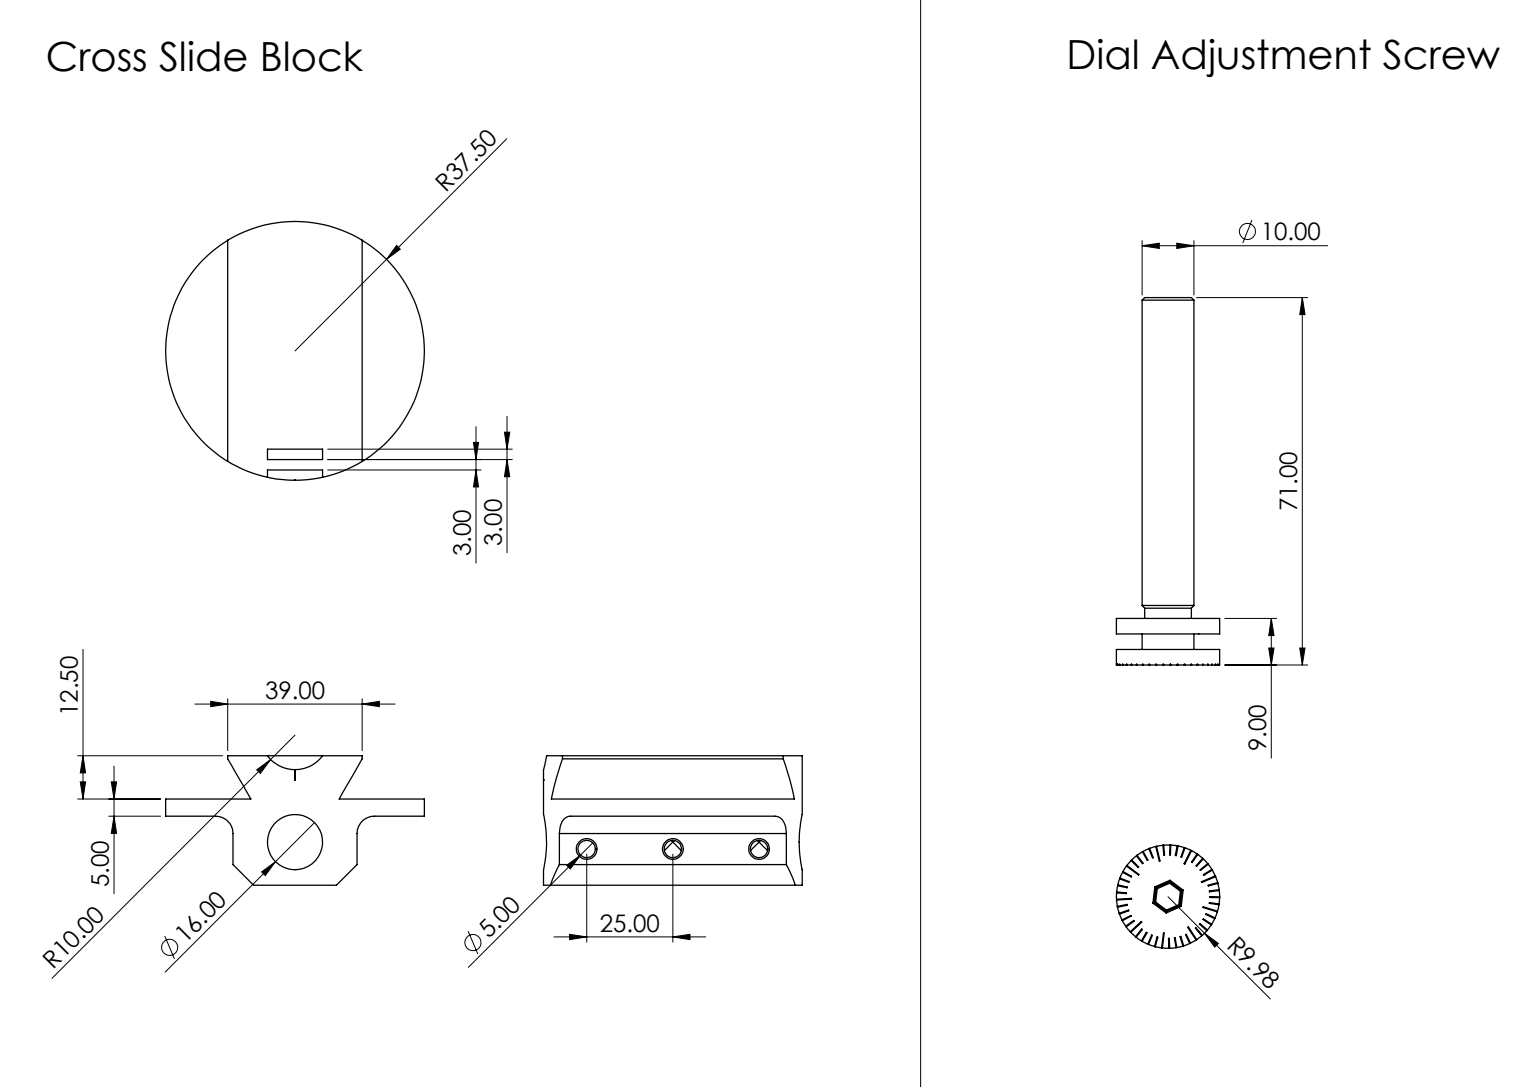
ISO-10303-21;
HEADER;
FILE_DESCRIPTION (('STEP AP214'),
    '1' );
FILE_NAME ('Dial Adjustment Screw.step',
    '2026-10-09T18:50:44',
    ( '' ),
    ( '' ),
    'SwSTEP 2.0',
    'SolidWorks 2026',
    '' );
FILE_SCHEMA (( 'AUTOMOTIVE_DESIGN' ));
ENDSEC;

DATA;
#4=EDGE_CURVE ( 'NONE', #9153, #8466, #14460, .T. ) ;
#6=LINE ( 'NONE', #11551, #10906 ) ;
#7=EDGE_CURVE ( 'NONE', #9450, #4202, #8492, .T. ) ;
#8=LINE ( 'NONE', #14787, #7820 ) ;
#11=ORIENTED_EDGE ( 'NONE', *, *, #1671, .F. ) ;
#12=DIRECTION ( 'NONE',  ( 8.018662683283438208E-16, -5.975035461963189015E-16, -1.000000000000000000 ) ) ;
#13=EDGE_LOOP ( 'NONE', ( #14568, #7332, #7097, #12565 ) ) ;
#14=CARTESIAN_POINT ( 'NONE',  ( -24.38380099443793725, -15.36048369738253427, 57.00231026484397745 ) ) ;
#15=ORIENTED_EDGE ( 'NONE', *, *, #4138, .F. ) ;
#17=VERTEX_POINT ( 'NONE', #8566 ) ;
#18=AXIS2_PLACEMENT_3D ( 'NONE', #7899, #12589, #2105 ) ;
#20=ORIENTED_EDGE ( 'NONE', *, *, #787, .F. ) ;
#25=ADVANCED_FACE ( 'NONE', ( #12243 ), #13329, .T. ) ;
#27=CARTESIAN_POINT ( 'NONE',  ( -8.600581100527527667, -9.311215824554304632, 56.85231026484400019 ) ) ;
#30=PLANE ( 'NONE',  #7847 ) ;
#31=ORIENTED_EDGE ( 'NONE', *, *, #8737, .F. ) ;
#32=DIRECTION ( 'NONE',  ( 0.4895147004624025855, -0.8719950447285834683, 9.135454576425998749E-16 ) ) ;
#33=VERTEX_POINT ( 'NONE', #4056 ) ;
#34=VERTEX_POINT ( 'NONE', #8713 ) ;
#35=CARTESIAN_POINT ( 'NONE',  ( -10.39628701978575975, -6.002951807498697612, 56.85231026484398598 ) ) ;
#43=CARTESIAN_POINT ( 'NONE',  ( -15.50552586659557797, -13.55703840903364288, 56.85231026484398598 ) ) ;
#46=CARTESIAN_POINT ( 'NONE',  ( -15.17726793795939599, -10.75904990174046461, 51.00231026484399166 ) ) ;
#49=ORIENTED_EDGE ( 'NONE', *, *, #8035, .T. ) ;
#52=ORIENTED_EDGE ( 'NONE', *, *, #5707, .T. ) ;
#54=EDGE_LOOP ( 'NONE', ( #11405, #3978, #7502, #8559 ) ) ;
#55=EDGE_CURVE ( 'NONE', #11066, #9490, #2977, .T. ) ;
#56=VECTOR ( 'NONE', #14424, 999.9999999999998863 ) ;
#57=VECTOR ( 'NONE', #8652, 999.9999999999998863 ) ;
#58=DIRECTION ( 'NONE',  ( -0.5104125104778984845, -0.8599296884906632021, 1.045284632676530333E-16 ) ) ;
#61=CARTESIAN_POINT ( 'NONE',  ( -12.46042140754850713, -23.00808483377100444, 57.00231026484399166 ) ) ;
#62=ORIENTED_EDGE ( 'NONE', *, *, #12874, .F. ) ;
#63=DIRECTION ( 'NONE',  ( -0.3306575217771102193, 0.9437508163134058492, -8.290375725550400094E-16 ) ) ;
#65=DIRECTION ( 'NONE',  ( 0.9354976265738682573, -0.3533329742249642913, 9.612616959383187437E-16 ) ) ;
#66=ORIENTED_EDGE ( 'NONE', *, *, #12766, .T. ) ;
#67=CIRCLE ( 'NONE', #8607, 9.974999999999999645 ) ;
#68=AXIS2_PLACEMENT_3D ( 'NONE', #8168, #77, #12858 ) ;
#70=ORIENTED_EDGE ( 'NONE', *, *, #13189, .F. ) ;
#72=EDGE_LOOP ( 'NONE', ( #9972, #5659, #4429, #2400 ) ) ;
#77=DIRECTION ( 'NONE',  ( 0.7350174335289139105, -0.6780482080269579770, 9.945218953682734920E-16 ) ) ;
#78=DIRECTION ( 'NONE',  ( 0.9931883319083343320, -0.1165201156931293391, 8.660254037844387408E-16 ) ) ;
#80=VECTOR ( 'NONE', #13700, 1000.000000000000114 ) ;
#83=PLANE ( 'NONE',  #4186 ) ;
#84=CARTESIAN_POINT ( 'NONE',  ( -7.424382730750140880, -13.52981220323889566, 56.85231026484400019 ) ) ;
#85=ORIENTED_EDGE ( 'NONE', *, *, #97, .F. ) ;
#87=ORIENTED_EDGE ( 'NONE', *, *, #11967, .T. ) ;
#94=LINE ( 'NONE', #9566, #672 ) ;
#96=DIRECTION ( 'NONE',  ( -8.018662683283438208E-16, 5.975035461963189015E-16, 1.000000000000000000 ) ) ;
#97=EDGE_CURVE ( 'NONE', #6821, #6890, #11166, .T. ) ;
#100=LINE ( 'NONE', #14015, #4170 ) ;
#105=CARTESIAN_POINT ( 'NONE',  ( -11.67714598312096008, -19.46131314156662384, 56.85231026484400019 ) ) ;
#113=ORIENTED_EDGE ( 'NONE', *, *, #12612, .F. ) ;
#115=EDGE_CURVE ( 'NONE', #11608, #7250, #12699, .T. ) ;
#117=EDGE_CURVE ( 'NONE', #4448, #10428, #688, .T. ) ;
#118=VERTEX_POINT ( 'NONE', #5499 ) ;
#119=CARTESIAN_POINT ( 'NONE',  ( -15.49969986081092088, -13.50737899243822504, 57.00231026484397745 ) ) ;
#123=LINE ( 'NONE', #4934, #14525 ) ;
#124=COLOUR_RGB ( '', 0.72549020, 0.75294118, 0.79215686) ;
#127=ORIENTED_EDGE ( 'NONE', *, *, #115, .F. ) ;
#129=DIRECTION ( 'NONE',  ( 0.9645173894937585368, 0.2640193276336892936, 6.156614753256587028E-16 ) ) ;
#131=CARTESIAN_POINT ( 'NONE',  ( -8.744347237509680681, -17.93190845158491342, 57.00231026484399166 ) ) ;
#132=ADVANCED_FACE ( 'NONE', ( #4206 ), #14685, .F. ) ;
#135=ORIENTED_EDGE ( 'NONE', *, *, #11324, .F. ) ;
#137=VECTOR ( 'NONE', #5946, 999.9999999999998863 ) ;
#141=DIRECTION ( 'NONE',  ( -8.018662683283438208E-16, 5.975035461963189015E-16, 1.000000000000000000 ) ) ;
#149=PLANE ( 'NONE',  #14987 ) ;
#150=VERTEX_POINT ( 'NONE', #916 ) ;
#154=FACE_OUTER_BOUND ( 'NONE', #467, .T. ) ;
#156=CARTESIAN_POINT ( 'NONE',  ( -17.71860670988920816, -11.85398021090886367, 51.00231026484399166 ) ) ;
#157=VECTOR ( 'NONE', #7597, 1000.000000000000114 ) ;
#159=EDGE_CURVE ( 'NONE', #10747, #3108, #3053, .T. ) ;
#165=ORIENTED_EDGE ( 'NONE', *, *, #2149, .T. ) ;
#166=DIRECTION ( 'NONE',  ( 8.018662683283438208E-16, -5.975035461963189015E-16, -1.000000000000000000 ) ) ;
#167=ORIENTED_EDGE ( 'NONE', *, *, #12641, .F. ) ;
#169=ORIENTED_EDGE ( 'NONE', *, *, #13036, .F. ) ;
#171=CARTESIAN_POINT ( 'NONE',  ( -15.49969986081092088, -13.50737899243822504, 56.85231026484398598 ) ) ;
#173=FACE_OUTER_BOUND ( 'NONE', #4854, .T. ) ;
#175=SHAPE_REPRESENTATION_RELATIONSHIP ( 'NONE' , 'NONE' ,  #13495, #6601 ) ;
#176=CARTESIAN_POINT ( 'NONE',  ( -18.41596830400278506, -14.76384693893611910, 57.00231026484397745 ) ) ;
#178=AXIS2_PLACEMENT_3D ( 'NONE', #14596, #7550, #6095 ) ;
#183=EDGE_LOOP ( 'NONE', ( #8383, #10689, #169, #12159 ) ) ;
#185=AXIS2_PLACEMENT_3D ( 'NONE', #4466, #10423, #5753 ) ;
#186=VERTEX_POINT ( 'NONE', #14912 ) ;
#188=ORIENTED_EDGE ( 'NONE', *, *, #5314, .T. ) ;
#191=FACE_OUTER_BOUND ( 'NONE', #10169, .T. ) ;
#192=DIRECTION ( 'NONE',  ( 0.5975035461963189576, 0.8018662683283437342, 0.000000000000000000 ) ) ;
#193=EDGE_CURVE ( 'NONE', #1606, #4275, #8746, .T. ) ;
#194=EDGE_CURVE ( 'NONE', #4315, #8561, #7264, .T. ) ;
#195=CARTESIAN_POINT ( 'NONE',  ( -15.49969986081091022, -13.50737899243823215, 46.00231026484398456 ) ) ;
#196=LINE ( 'NONE', #3708, #2723 ) ;
#197=CARTESIAN_POINT ( 'NONE',  ( -8.681233859935401753, -6.226640953275941470, 56.85231026484398598 ) ) ;
#203=EDGE_LOOP ( 'NONE', ( #1328, #2305, #6910, #14868 ) ) ;
#204=ORIENTED_EDGE ( 'NONE', *, *, #10815, .T. ) ;
#207=ORIENTED_EDGE ( 'NONE', *, *, #11956, .F. ) ;
#210=CARTESIAN_POINT ( 'NONE',  ( -17.47506273705024071, -21.33739760717825718, 56.85231026484400019 ) ) ;
#211=EDGE_CURVE ( 'NONE', #12427, #2827, #11544, .T. ) ;
#212=DIRECTION ( 'NONE',  ( 0.6859287159822015090, -0.7276687409742212953, 9.848077530122081084E-16 ) ) ;
#215=ORIENTED_EDGE ( 'NONE', *, *, #13065, .F. ) ;
#217=CARTESIAN_POINT ( 'NONE',  ( -10.84210729886283531, -6.910555398701176522, 56.85231026484398598 ) ) ;
#218=ORIENTED_EDGE ( 'NONE', *, *, #1842, .T. ) ;
#221=VERTEX_POINT ( 'NONE', #11762 ) ;
#224=ORIENTED_EDGE ( 'NONE', *, *, #12134, .T. ) ;
#225=FACE_OUTER_BOUND ( 'NONE', #3388, .T. ) ;
#227=EDGE_CURVE ( 'NONE', #9086, #8293, #11691, .T. ) ;
#230=VECTOR ( 'NONE', #6999, 1000.000000000000000 ) ;
#235=DIRECTION ( 'NONE',  ( -8.018662683283438208E-16, 5.975035461963189015E-16, 1.000000000000000000 ) ) ;
#236=CARTESIAN_POINT ( 'NONE',  ( -16.32407967933980686, -20.53418644068968746, 57.00231026484399166 ) ) ;
#239=DIRECTION ( 'NONE',  ( 8.018662683283438208E-16, -5.975035461963189015E-16, -1.000000000000000000 ) ) ;
#242=CARTESIAN_POINT ( 'NONE',  ( -18.04596724311489808, -11.61005040962811563, 57.00231026484397745 ) ) ;
#247=ORIENTED_EDGE ( 'NONE', *, *, #4682, .F. ) ;
#252=DIRECTION ( 'NONE',  ( 0.5975035461963189576, 0.8018662683283437342, 0.000000000000000000 ) ) ;
#254=CARTESIAN_POINT ( 'NONE',  ( -24.01584079503567182, -10.37104457333969876, 57.00231026484397745 ) ) ;
#255=CARTESIAN_POINT ( 'NONE',  ( -15.47224238247604511, -13.54916519690201149, 56.85231026484398598 ) ) ;
#256=VECTOR ( 'NONE', #11415, 1000.000000000000114 ) ;
#257=ORIENTED_EDGE ( 'NONE', *, *, #6613, .T. ) ;
#262=ORIENTED_EDGE ( 'NONE', *, *, #3647, .F. ) ;
#263=CARTESIAN_POINT ( 'NONE',  ( -23.39388780995641781, -11.80648316271623877, 56.85231026484398598 ) ) ;
#270=CIRCLE ( 'NONE', #3683, 9.974999999999999645 ) ;
#282=EDGE_CURVE ( 'NONE', #626, #3416, #13005, .T. ) ;
#284=ADVANCED_FACE ( 'NONE', ( #2513 ), #11846, .F. ) ;
#286=AXIS2_PLACEMENT_3D ( 'NONE', #4236, #8813, #2856 ) ;
#288=EDGE_CURVE ( 'NONE', #14042, #11463, #13916, .T. ) ;
#289=CARTESIAN_POINT ( 'NONE',  ( -24.32830346761242879, -18.15026423267100597, 56.85231026484398598 ) ) ;
#291=ORIENTED_EDGE ( 'NONE', *, *, #2351, .F. ) ;
#294=ORIENTED_EDGE ( 'NONE', *, *, #11168, .F. ) ;
#295=DIRECTION ( 'NONE',  ( 0.9437508163134050720, 0.3306575217771122732, 5.591929034707472732E-16 ) ) ;
#298=LINE ( 'NONE', #4183, #349 ) ;
#306=DIRECTION ( 'NONE',  ( 0.2301973227387160703, -0.9731439732146149879, 7.660444431189776467E-16 ) ) ;
#307=VECTOR ( 'NONE', #2927, 999.9999999999998863 ) ;
#308=CIRCLE ( 'NONE', #8106, 9.974999999999999645 ) ;
#309=VECTOR ( 'NONE', #4436, 1000.000000000000000 ) ;
#310=LINE ( 'NONE', #9632, #1371 ) ;
#315=CARTESIAN_POINT ( 'NONE',  ( -23.54151295824578227, -12.77219731018227300, 57.00231026484397745 ) ) ;
#316=CARTESIAN_POINT ( 'NONE',  ( -6.938526287600617515, -8.388108336439909607, 57.00231026484399166 ) ) ;
#319=ORIENTED_EDGE ( 'NONE', *, *, #11952, .F. ) ;
#320=DIRECTION ( 'NONE',  ( -0.1855175943453192255, -0.9826409426582660700, 4.383711467890751032E-16 ) ) ;
#321=FACE_OUTER_BOUND ( 'NONE', #7198, .T. ) ;
#322=EDGE_LOOP ( 'NONE', ( #14404, #10872, #12403, #8371 ) ) ;
#323=VECTOR ( 'NONE', #13122, 1000.000000000000114 ) ;
#325=DIRECTION ( 'NONE',  ( 0.9988970074402866439, -0.04695496274985035134, 8.290375725550441510E-16 ) ) ;
#326=VECTOR ( 'NONE', #4845, 1000.000000000000000 ) ;
#329=DIRECTION ( 'NONE',  ( -8.018662683283438208E-16, 5.975035461963189015E-16, 1.000000000000000000 ) ) ;
#336=DIRECTION ( 'NONE',  ( 8.018662683283438208E-16, -5.975035461963189015E-16, -1.000000000000000000 ) ) ;
#337=VERTEX_POINT ( 'NONE', #13812 ) ;
#341=LINE ( 'NONE', #7503, #3156 ) ;
#343=ORIENTED_EDGE ( 'NONE', *, *, #4783, .T. ) ;
#346=ORIENTED_EDGE ( 'NONE', *, *, #6966, .T. ) ;
#347=LINE ( 'NONE', #11884, #5404 ) ;
#348=DIRECTION ( 'NONE',  ( 8.018662683283438208E-16, -5.975035461963189015E-16, -1.000000000000000000 ) ) ;
#349=VECTOR ( 'NONE', #8838, 1000.000000000000114 ) ;
#351=CARTESIAN_POINT ( 'NONE',  ( -16.26465502354534465, -4.464365468230401923, 56.85231026484398598 ) ) ;
#353=CARTESIAN_POINT ( 'NONE',  ( -15.49969986081091022, -13.50737899243823215, 45.50231026484398456 ) ) ;
#354=EDGE_CURVE ( 'NONE', #745, #9450, #1038, .T. ) ;
#355=CARTESIAN_POINT ( 'NONE',  ( -20.31707134655588121, -4.772760685475329723, 57.00231026484397745 ) ) ;
#358=CARTESIAN_POINT ( 'NONE',  ( -17.98267069058175593, -13.21607870320540279, 51.25231026484399166 ) ) ;
#359=CARTESIAN_POINT ( 'NONE',  ( -14.15531688186919901, -11.70317988869945580, 51.25231026484399166 ) ) ;
#361=ORIENTED_EDGE ( 'NONE', *, *, #5740, .T. ) ;
#362=VECTOR ( 'NONE', #6575, 1000.000000000000000 ) ;
#366=AXIS2_PLACEMENT_3D ( 'NONE', #8590, #7864, #7944 ) ;
#368=VECTOR ( 'NONE', #4802, 1000.000000000000000 ) ;
#369=LINE ( 'NONE', #7224, #14846 ) ;
#371=CARTESIAN_POINT ( 'NONE',  ( -9.204203523554131294, -8.449911655164932256, 56.85231026484398598 ) ) ;
#373=DIRECTION ( 'NONE',  ( -8.018662683283438208E-16, 5.975035461963189015E-16, 1.000000000000000000 ) ) ;
#375=LINE ( 'NONE', #5935, #15083 ) ;
#378=EDGE_CURVE ( 'NONE', #12795, #6835, #5541, .T. ) ;
#382=LINE ( 'NONE', #13374, #828 ) ;
#383=EDGE_LOOP ( 'NONE', ( #11482, #7292, #5223, #897 ) ) ;
#391=EDGE_CURVE ( 'NONE', #6478, #4633, #15029, .T. ) ;
#392=CARTESIAN_POINT ( 'NONE',  ( -7.829332545557822876, -7.130382030772259405, 54.00231026484399166 ) ) ;
#395=CARTESIAN_POINT ( 'NONE',  ( -10.27295246487022240, -6.088325032597582620, 56.85231026484398598 ) ) ;
#396=ORIENTED_EDGE ( 'NONE', *, *, #11686, .F. ) ;
#398=EDGE_LOOP ( 'NONE', ( #9560, #11347, #6065, #9121, #218, #1341, #14177, #5755, #9138, #2250, #8409, #841, #3009, #12196, #3012, #215, #6805, #10450, #11048, #3124, #8673, #4543, #13338, #1727, #6461, #20, #10686, #9196, #12441, #10883, #7309, #5437, #1481, #5195, #2738, #14936, #13462, #1244, #15109, #5142, #4772, #10095, #7336, #13120, #462, #7253, #2154, #14889, #4656, #3287, #6719, #5542, #5255, #5721, #5056, #7185, #6602, #11840, #12110, #9524, #2176, #7888, #3618, #840, #2267, #1060, #11943, #5202, #12654, #8703, #7274, #1364, #12906, #13394, #10919, #9271, #428, #5605, #11, #4999, #1774, #7100, #4480, #2417, #10113, #7120, #11578, #6781, #13390, #6535, #3685, #6336, #9887, #10899, #2644, #11457 ) ) ;
#400=PLANE ( 'NONE',  #4949 ) ;
#401=CARTESIAN_POINT ( 'NONE',  ( -7.426192534185826588, -13.67980128487994129, 56.85231026484400019 ) ) ;
#403=CIRCLE ( 'NONE', #7222, 9.974999999999999645 ) ;
#407=CARTESIAN_POINT ( 'NONE',  ( -8.639554752241616953, -9.247137322136806503, 57.00231026484399166 ) ) ;
#408=CARTESIAN_POINT ( 'NONE',  ( -15.83606446161809522, -16.37446674635458166, 56.75231026484397745 ) ) ;
#413=VERTEX_POINT ( 'NONE', #3179 ) ;
#414=CARTESIAN_POINT ( 'NONE',  ( -17.86883904694317593, -3.817807045405069655, 56.85231026484398598 ) ) ;
#417=CARTESIAN_POINT ( 'NONE',  ( -15.49969986081092088, -13.50737899243822504, 57.00231026484397745 ) ) ;
#420=DIRECTION ( 'NONE',  ( -8.018662683283438208E-16, 5.975035461963189015E-16, 1.000000000000000000 ) ) ;
#423=PRODUCT_DEFINITION_SHAPE ( 'NONE', 'NONE',  #14249 ) ;
#426=ORIENTED_EDGE ( 'NONE', *, *, #5229, .F. ) ;
#428=ORIENTED_EDGE ( 'NONE', *, *, #3740, .T. ) ;
#430=ORIENTED_EDGE ( 'NONE', *, *, #211, .T. ) ;
#432=PLANE ( 'NONE',  #8349 ) ;
#436=CARTESIAN_POINT ( 'NONE',  ( -15.54961651457173488, -13.51026476396819831, 56.85231026484398598 ) ) ;
#439=FACE_OUTER_BOUND ( 'NONE', #5049, .T. ) ;
#440=CARTESIAN_POINT ( 'NONE',  ( -6.488891646287396675, -12.42729319905174634, 57.00231026484399166 ) ) ;
#443=CARTESIAN_POINT ( 'NONE',  ( -18.18846581869435042, -17.11577719991577595, 48.00231026484398456 ) ) ;
#446=LINE ( 'NONE', #6386, #12519 ) ;
#449=CARTESIAN_POINT ( 'NONE',  ( -14.10579935493720782, -22.47500361547664127, 56.85231026484400019 ) ) ;
#450=ORIENTED_EDGE ( 'NONE', *, *, #10660, .T. ) ;
#451=DIRECTION ( 'NONE',  ( -0.4491835085186243748, -0.8934395198752397294, 1.736481776669299976E-16 ) ) ;
#452=AXIS2_PLACEMENT_3D ( 'NONE', #12447, #14978, #15050 ) ;
#456=AXIS2_PLACEMENT_3D ( 'NONE', #14616, #2988, #10880 ) ;
#457=FACE_OUTER_BOUND ( 'NONE', #11590, .T. ) ;
#462=ORIENTED_EDGE ( 'NONE', *, *, #5462, .T. ) ;
#464=CARTESIAN_POINT ( 'NONE',  ( -6.766506000727597225, -11.03906478995046214, 57.00231026484399166 ) ) ;
#467=EDGE_LOOP ( 'NONE', ( #13198, #13690 ) ) ;
#469=ORIENTED_EDGE ( 'NONE', *, *, #1383, .F. ) ;
#471=DIRECTION ( 'NONE',  ( 0.02283895005205794151, -0.9997391571607663341, 6.156614753256579139E-16 ) ) ;
#473=ADVANCED_FACE ( 'NONE', ( #4936 ), #4865, .T. ) ;
#474=EDGE_CURVE ( 'NONE', #5883, #11022, #2563, .T. ) ;
#475=CARTESIAN_POINT ( 'NONE',  ( -9.452813543643186378, -20.27468391147722926, 56.85231026484400019 ) ) ;
#480=PLANE ( 'NONE',  #13859 ) ;
#482=EDGE_CURVE ( 'NONE', #8690, #13854, #8445, .T. ) ;
#485=ORIENTED_EDGE ( 'NONE', *, *, #2144, .T. ) ;
#489=PLANE ( 'NONE',  #5895 ) ;
#494=DIRECTION ( 'NONE',  ( -8.018662683283438208E-16, 5.975035461963189015E-16, 1.000000000000000000 ) ) ;
#495=DIRECTION ( 'NONE',  ( 8.018662683283438208E-16, -5.975035461963189015E-16, -1.000000000000000000 ) ) ;
#497=FACE_OUTER_BOUND ( 'NONE', #9125, .T. ) ;
#498=ORIENTED_EDGE ( 'NONE', *, *, #6384, .T. ) ;
#500=DIRECTION ( 'NONE',  ( -8.018662683283438208E-16, 5.975035461963189015E-16, 1.000000000000000000 ) ) ;
#501=ORIENTED_EDGE ( 'NONE', *, *, #8338, .F. ) ;
#502=ORIENTED_EDGE ( 'NONE', *, *, #12063, .T. ) ;
#503=EDGE_CURVE ( 'NONE', #10963, #7558, #4786, .T. ) ;
#505=VERTEX_POINT ( 'NONE', #5991 ) ;
#506=CARTESIAN_POINT ( 'NONE',  ( -25.21423696146293736, -11.24278324042066046, 54.00231026484397745 ) ) ;
#512=CARTESIAN_POINT ( 'NONE',  ( -11.08622897860377954, -4.561882931743225456, 56.85231026484398598 ) ) ;
#514=EDGE_LOOP ( 'NONE', ( #9562, #13979, #13683, #11446 ) ) ;
#517=DIRECTION ( 'NONE',  ( -8.018662683283438208E-16, 5.975035461963189015E-16, 1.000000000000000000 ) ) ;
#519=LINE ( 'NONE', #449, #1066 ) ;
#520=ORIENTED_EDGE ( 'NONE', *, *, #7971, .F. ) ;
#522=VECTOR ( 'NONE', #10897, 1000.000000000000114 ) ;
#523=FACE_OUTER_BOUND ( 'NONE', #3562, .T. ) ;
#524=CARTESIAN_POINT ( 'NONE',  ( -7.426192534185826588, -13.67980128487993952, 57.00231026484399166 ) ) ;
#527=ORIENTED_EDGE ( 'NONE', *, *, #9531, .T. ) ;
#529=LINE ( 'NONE', #4977, #7993 ) ;
#530=AXIS2_PLACEMENT_3D ( 'NONE', #12947, #6943, #12 ) ;
#532=VERTEX_POINT ( 'NONE', #13131 ) ;
#533=ORIENTED_EDGE ( 'NONE', *, *, #1466, .T. ) ;
#536=ORIENTED_EDGE ( 'NONE', *, *, #10912, .T. ) ;
#537=DIRECTION ( 'NONE',  ( 0.1165201156931293391, 0.9931883319083343320, -4.999999999999998416E-16 ) ) ;
#538=DIRECTION ( 'NONE',  ( -0.9673062255102924389, 0.2536112499260064768, -9.271838545667833343E-16 ) ) ;
#539=VECTOR ( 'NONE', #6589, 999.9999999999998863 ) ;
#541=VECTOR ( 'NONE', #2213, 1000.000000000000000 ) ;
#544=CARTESIAN_POINT ( 'NONE',  ( -5.526612771747954511, -13.70272205979775215, 57.00231026484399166 ) ) ;
#550=CIRCLE ( 'NONE', #2008, 5.000000000000000000 ) ;
#551=VERTEX_POINT ( 'NONE', #4711 ) ;
#552=AXIS2_PLACEMENT_3D ( 'NONE', #3432, #12781, #11690 ) ;
#553=ORIENTED_EDGE ( 'NONE', *, *, #12726, .F. ) ;
#555=ORIENTED_EDGE ( 'NONE', *, *, #2708, .T. ) ;
#557=CIRCLE ( 'NONE', #1776, 9.974999999999999645 ) ;
#560=VERTEX_POINT ( 'NONE', #197 ) ;
#561=DIRECTION ( 'NONE',  ( -0.9183863840214728791, -0.3956847857120156520, -4.999999999999998416E-16 ) ) ;
#564=CARTESIAN_POINT ( 'NONE',  ( -9.204203523554131294, -8.449911655164932256, 56.85231026484398598 ) ) ;
#568=EDGE_CURVE ( 'NONE', #9210, #8324, #1106, .T. ) ;
#572=VERTEX_POINT ( 'NONE', #7518 ) ;
#579=VECTOR ( 'NONE', #5511, 1000.000000000000000 ) ;
#580=CIRCLE ( 'NONE', #12062, 9.974999999999999645 ) ;
#585=AXIS2_PLACEMENT_3D ( 'NONE', #3960, #12144, #9989 ) ;
#586=DIRECTION ( 'NONE',  ( -8.018662683283438208E-16, 5.975035461963189015E-16, 1.000000000000000000 ) ) ;
#588=ORIENTED_EDGE ( 'NONE', *, *, #6627, .F. ) ;
#591=CARTESIAN_POINT ( 'NONE',  ( -12.69917084408742269, -12.16466883763078144, 57.00231026484397745 ) ) ;
#592=EDGE_LOOP ( 'NONE', ( #1009, #7727, #14645, #8081 ) ) ;
#593=EDGE_CURVE ( 'NONE', #3314, #3333, #9963, .T. ) ;
#595=PLANE ( 'NONE',  #7643 ) ;
#596=AXIS2_PLACEMENT_3D ( 'NONE', #4175, #9910, #7609 ) ;
#597=ORIENTED_EDGE ( 'NONE', *, *, #4963, .F. ) ;
#598=LINE ( 'NONE', #13310, #13985 ) ;
#599=VECTOR ( 'NONE', #12678, 1000.000000000000114 ) ;
#600=FACE_OUTER_BOUND ( 'NONE', #3661, .T. ) ;
#601=EDGE_CURVE ( 'NONE', #7394, #8222, #3773, .T. ) ;
#602=CARTESIAN_POINT ( 'NONE',  ( -24.36945568363038461, -11.58678490633884373, 56.85231026484398598 ) ) ;
#604=DIRECTION ( 'NONE',  ( -8.018662683283439195E-16, 5.975035461963190001E-16, 1.000000000000000000 ) ) ;
#612=VERTEX_POINT ( 'NONE', #6137 ) ;
#614=FACE_OUTER_BOUND ( 'NONE', #3144, .T. ) ;
#615=ORIENTED_EDGE ( 'NONE', *, *, #11602, .F. ) ;
#616=CARTESIAN_POINT ( 'NONE',  ( -22.67472226038933059, -17.21206232108429290, 56.85231026484398598 ) ) ;
#617=LINE ( 'NONE', #14613, #11114 ) ;
#618=VECTOR ( 'NONE', #14146, 1000.000000000000000 ) ;
#619=EDGE_CURVE ( 'NONE', #13349, #1021, #9822, .T. ) ;
#621=CARTESIAN_POINT ( 'NONE',  ( -8.971570239337625097, -21.04953708182106453, 54.00231026484400587 ) ) ;
#625=DIRECTION ( 'NONE',  ( 8.018662683283438208E-16, -5.975035461963189015E-16, -1.000000000000000000 ) ) ;
#626=VERTEX_POINT ( 'NONE', #2711 ) ;
#628=LINE ( 'NONE', #12406, #4473 ) ;
#629=ORIENTED_EDGE ( 'NONE', *, *, #8780, .T. ) ;
#631=DIRECTION ( 'NONE',  ( 0.7953815700667045130, 0.6061090314441981430, 2.756373558170028881E-16 ) ) ;
#635=ADVANCED_FACE ( 'NONE', ( #7365 ), #7594, .F. ) ;
#636=LINE ( 'NONE', #10968, #4651 ) ;
#637=DIRECTION ( 'NONE',  ( 0.9885168150181788960, -0.1511109077013150503, 8.829475928589270966E-16 ) ) ;
#638=EDGE_CURVE ( 'NONE', #2290, #7645, #5016, .T. ) ;
#639=CIRCLE ( 'NONE', #9181, 5.000000000000000000 ) ;
#640=DIRECTION ( 'NONE',  ( 0.2196982563774038943, 0.9755678736739584744, -4.067366430757999696E-16 ) ) ;
#642=VERTEX_POINT ( 'NONE', #14489 ) ;
#643=LINE ( 'NONE', #8596, #7755 ) ;
#646=ORIENTED_EDGE ( 'NONE', *, *, #10912, .F. ) ;
#652=CARTESIAN_POINT ( 'NONE',  ( -7.902754534677060683, -18.47202114588016642, 57.00231026484399166 ) ) ;
#653=ADVANCED_FACE ( 'NONE', ( #8814 ), #3427, .T. ) ;
#656=EDGE_CURVE ( 'NONE', #2388, #14032, #13686, .T. ) ;
#657=DIRECTION ( 'NONE',  ( 0.9918751611018171710, 0.1272150336605075427, 7.193398003386516820E-16 ) ) ;
#659=ORIENTED_EDGE ( 'NONE', *, *, #13177, .F. ) ;
#660=DIRECTION ( 'NONE',  ( -8.018662683283438208E-16, 5.975035461963189015E-16, 1.000000000000000000 ) ) ;
#662=EDGE_CURVE ( 'NONE', #1582, #10428, #4356, .T. ) ;
#664=CARTESIAN_POINT ( 'NONE',  ( -25.21423696146293736, -11.24278324042065869, 57.00231026484397745 ) ) ;
#667=CARTESIAN_POINT ( 'NONE',  ( -20.33437667196779586, -7.039214636791314206, 57.00231026484397745 ) ) ;
#668=PLANE ( 'NONE',  #10986 ) ;
#669=EDGE_CURVE ( 'NONE', #6892, #5883, #6927, .T. ) ;
#671=FACE_OUTER_BOUND ( 'NONE', #6924, .T. ) ;
#672=VECTOR ( 'NONE', #3759, 1000.000000000000000 ) ;
#673=CARTESIAN_POINT ( 'NONE',  ( -22.55857771067089246, -13.99059064457067336, 56.85231026484398598 ) ) ;
#674=LINE ( 'NONE', #5559, #2557 ) ;
#675=ORIENTED_EDGE ( 'NONE', *, *, #3273, .T. ) ;
#678=ORIENTED_EDGE ( 'NONE', *, *, #6782, .T. ) ;
#679=VECTOR ( 'NONE', #12925, 1000.000000000000000 ) ;
#683=ORIENTED_EDGE ( 'NONE', *, *, #15059, .F. ) ;
#685=VECTOR ( 'NONE', #13993, 1000.000000000000000 ) ;
#686=VECTOR ( 'NONE', #8907, 1000.000000000000000 ) ;
#688=LINE ( 'NONE', #14986, #1664 ) ;
#689=FACE_OUTER_BOUND ( 'NONE', #11088, .T. ) ;
#692=AXIS2_PLACEMENT_3D ( 'NONE', #11251, #12556, #6566 ) ;
#693=DIRECTION ( 'NONE',  ( 8.018662683283438208E-16, -5.975035461963189015E-16, -1.000000000000000000 ) ) ;
#694=CARTESIAN_POINT ( 'NONE',  ( -15.82213178366242978, -16.25570808313599258, 51.00231026484399166 ) ) ;
#695=VECTOR ( 'NONE', #3479, 1000.000000000000000 ) ;
#696=CARTESIAN_POINT ( 'NONE',  ( -10.39628701978575975, -6.002951807498697612, 57.00231026484397745 ) ) ;
#699=LINE ( 'NONE', #12712, #5166 ) ;
#701=FACE_OUTER_BOUND ( 'NONE', #3699, .T. ) ;
#704=ORIENTED_EDGE ( 'NONE', *, *, #9052, .F. ) ;
#705=VECTOR ( 'NONE', #1786, 1000.000000000000000 ) ;
#707=DIRECTION ( 'NONE',  ( -0.9999272109403024578, 0.01206535623792159839, -8.090169943749490479E-16 ) ) ;
#710=PLANE ( 'NONE',  #9268 ) ;
#711=DIRECTION ( 'NONE',  ( 8.018662683283438208E-16, -5.975035461963189015E-16, -1.000000000000000000 ) ) ;
#712=FACE_OUTER_BOUND ( 'NONE', #3959, .T. ) ;
#715=CARTESIAN_POINT ( 'NONE',  ( -12.72810521832141362, -22.14910990341453001, 56.85231026484400019 ) ) ;
#719=CARTESIAN_POINT ( 'NONE',  ( -14.19354049678269192, -21.47604090745013750, 57.00231026484399166 ) ) ;
#721=ORIENTED_EDGE ( 'NONE', *, *, #9534, .T. ) ;
#725=ORIENTED_EDGE ( 'NONE', *, *, #11167, .T. ) ;
#727=VECTOR ( 'NONE', #4187, 1000.000000000000114 ) ;
#729=EDGE_CURVE ( 'NONE', #10731, #4396, #14907, .T. ) ;
#731=PLANE ( 'NONE',  #6812 ) ;
#735=ORIENTED_EDGE ( 'NONE', *, *, #7834, .F. ) ;
#737=PLANE ( 'NONE',  #10590 ) ;
#738=ORIENTED_EDGE ( 'NONE', *, *, #13177, .T. ) ;
#739=PLANE ( 'NONE',  #6134 ) ;
#743=EDGE_CURVE ( 'NONE', #11608, #1039, #13759, .T. ) ;
#744=LINE ( 'NONE', #11372, #7897 ) ;
#745=VERTEX_POINT ( 'NONE', #8076 ) ;
#747=EDGE_CURVE ( 'NONE', #1568, #4448, #14520, .T. ) ;
#748=DIRECTION ( 'NONE',  ( 0.05771543059946733500, -0.9983330752162417054, 6.427876096865391919E-16 ) ) ;
#751=AXIS2_PLACEMENT_3D ( 'NONE', #13106, #11949, #1467 ) ;
#754=CARTESIAN_POINT ( 'NONE',  ( -22.64031343690345111, -17.27870339600297811, 56.85231026484398598 ) ) ;
#757=DIRECTION ( 'NONE',  ( 0.5975035461963189576, 0.8018662683283437342, 0.000000000000000000 ) ) ;
#758=ADVANCED_FACE ( 'NONE', ( #14979 ), #10465, .T. ) ;
#764=DIRECTION ( 'NONE',  ( 0.5975035461963189576, 0.8018662683283437342, 0.000000000000000000 ) ) ;
#769=VECTOR ( 'NONE', #4307, 1000.000000000000000 ) ;
#772=FACE_OUTER_BOUND ( 'NONE', #10937, .T. ) ;
#773=ORIENTED_EDGE ( 'NONE', *, *, #13542, .F. ) ;
#782=ORIENTED_EDGE ( 'NONE', *, *, #10510, .F. ) ;
#783=CIRCLE ( 'NONE', #9322, 9.974999999999999645 ) ;
#784=CARTESIAN_POINT ( 'NONE',  ( -19.55678615628314532, -20.48959216528617233, 57.00231026484397745 ) ) ;
#785=CARTESIAN_POINT ( 'NONE',  ( -12.72810521832141362, -22.14910990341453001, 56.85231026484400019 ) ) ;
#787=EDGE_CURVE ( 'NONE', #6222, #34, #13589, .T. ) ;
#788=EDGE_CURVE ( 'NONE', #4102, #4546, #10127, .T. ) ;
#789=AXIS2_PLACEMENT_3D ( 'NONE', #6840, #972, #4339 ) ;
#791=DIRECTION ( 'NONE',  ( -0.9885168150181790070, 0.1511109077013141622, -8.829475928589267021E-16 ) ) ;
#792=AXIS2_PLACEMENT_3D ( 'NONE', #7913, #13894, #1044 ) ;
#796=ORIENTED_EDGE ( 'NONE', *, *, #4234, .T. ) ;
#797=PLANE ( 'NONE',  #14704 ) ;
#799=DIRECTION ( 'NONE',  ( -8.018662683283438208E-16, 5.975035461963189015E-16, 1.000000000000000000 ) ) ;
#800=ORIENTED_EDGE ( 'NONE', *, *, #7591, .F. ) ;
#801=EDGE_LOOP ( 'NONE', ( #1209, #6569, #11149, #361 ) ) ;
#805=CIRCLE ( 'NONE', #7388, 4.499999999999998224 ) ;
#806=AXIS2_PLACEMENT_3D ( 'NONE', #12633, #6793, #12710 ) ;
#807=LINE ( 'NONE', #13439, #14531 ) ;
#808=DIRECTION ( 'NONE',  ( 0.8772189822852974883, -0.4800904676395346682, 9.902680687415700047E-16 ) ) ;
#812=DIRECTION ( 'NONE',  ( -0.1165201156931293391, -0.9931883319083343320, 4.999999999999998416E-16 ) ) ;
#814=ORIENTED_EDGE ( 'NONE', *, *, #6711, .T. ) ;
#817=ORIENTED_EDGE ( 'NONE', *, *, #4925, .F. ) ;
#819=AXIS2_PLACEMENT_3D ( 'NONE', #10441, #15107, #1187 ) ;
#822=AXIS2_PLACEMENT_3D ( 'NONE', #13222, #373, #9613 ) ;
#825=ORIENTED_EDGE ( 'NONE', *, *, #1377, .T. ) ;
#826=CARTESIAN_POINT ( 'NONE',  ( -14.00594099532011683, -11.50271332161736915, 51.00231026484399166 ) ) ;
#828=VECTOR ( 'NONE', #1734, 1000.000000000000000 ) ;
#829=ADVANCED_FACE ( 'NONE', ( #5322 ), #8908, .F. ) ;
#830=DIRECTION ( 'NONE',  ( -0.7276687409742212953, -0.6859287159822015090, -1.736481776669299729E-16 ) ) ;
#831=CARTESIAN_POINT ( 'NONE',  ( -6.405625242116715690, -17.60596799715947114, 54.00231026484400587 ) ) ;
#832=LINE ( 'NONE', #11155, #5240 ) ;
#833=ADVANCED_FACE ( 'NONE', ( #14511 ), #1957, .F. ) ;
#834=ORIENTED_EDGE ( 'NONE', *, *, #12625, .T. ) ;
#839=CARTESIAN_POINT ( 'NONE',  ( -15.16333526000375187, -10.64029123852186132, 56.75231026484397745 ) ) ;
#840=ORIENTED_EDGE ( 'NONE', *, *, #4770, .F. ) ;
#841=ORIENTED_EDGE ( 'NONE', *, *, #7865, .F. ) ;
#843=FACE_OUTER_BOUND ( 'NONE', #937, .T. ) ;
#845=FACE_OUTER_BOUND ( 'NONE', #6168, .T. ) ;
#848=CARTESIAN_POINT ( 'NONE',  ( -11.71495923925436955, -5.812446346369147143, 56.85231026484398598 ) ) ;
#850=VECTOR ( 'NONE', #9016, 1000.000000000000000 ) ;
#852=CARTESIAN_POINT ( 'NONE',  ( -8.561607448813433052, -9.375294326971793879, 56.85231026484400019 ) ) ;
#853=CARTESIAN_POINT ( 'NONE',  ( -23.49646891012291050, -9.216349422280851300, 57.00231026484397745 ) ) ;
#854=CARTESIAN_POINT ( 'NONE',  ( -17.47506273705024071, -21.33739760717825718, 56.85231026484400019 ) ) ;
#856=CARTESIAN_POINT ( 'NONE',  ( -5.859109405273538407, -10.94619944609606677, 56.85231026484400019 ) ) ;
#857=ORIENTED_EDGE ( 'NONE', *, *, #5983, .F. ) ;
#858=VERTEX_POINT ( 'NONE', #4329 ) ;
#860=ORIENTED_EDGE ( 'NONE', *, *, #8404, .T. ) ;
#864=LINE ( 'NONE', #5521, #4901 ) ;
#867=ORIENTED_EDGE ( 'NONE', *, *, #6524, .T. ) ;
#868=LINE ( 'NONE', #11344, #14453 ) ;
#869=DIRECTION ( 'NONE',  ( 8.018662683283438208E-16, -5.975035461963189015E-16, -1.000000000000000000 ) ) ;
#870=ORIENTED_EDGE ( 'NONE', *, *, #5351, .F. ) ;
#873=CARTESIAN_POINT ( 'NONE',  ( -10.16926643994361967, -19.57302854922115287, 56.85231026484400019 ) ) ;
#875=ORIENTED_EDGE ( 'NONE', *, *, #14446, .F. ) ;
#877=DIRECTION ( 'NONE',  ( -0.9805849309054472940, -0.1960948578651647567, -6.691306063588586415E-16 ) ) ;
#878=EDGE_LOOP ( 'NONE', ( #6994, #13171 ) ) ;
#883=VECTOR ( 'NONE', #3949, 1000.000000000000000 ) ;
#889=CARTESIAN_POINT ( 'NONE',  ( -21.24026693782044717, -7.828337292084670551, 56.85231026484398598 ) ) ;
#891=ORIENTED_EDGE ( 'NONE', *, *, #9996, .T. ) ;
#892=ORIENTED_EDGE ( 'NONE', *, *, #11461, .F. ) ;
#893=CARTESIAN_POINT ( 'NONE',  ( -11.58094331127308507, -5.879823872646938732, 56.85231026484398598 ) ) ;
#896=CARTESIAN_POINT ( 'NONE',  ( -15.53979317422733786, -13.47750381512840967, 56.85231026484398598 ) ) ;
#897=ORIENTED_EDGE ( 'NONE', *, *, #7816, .T. ) ;
#898=LINE ( 'NONE', #7919, #2506 ) ;
#902=VECTOR ( 'NONE', #9320, 999.9999999999998863 ) ;
#903=CARTESIAN_POINT ( 'NONE',  ( -15.49969986081092088, -13.50737899243822504, 57.00231026484397745 ) ) ;
#904=CARTESIAN_POINT ( 'NONE',  ( -17.40065610530428586, -5.145404622917534532, 57.00231026484397745 ) ) ;
#905=ORIENTED_EDGE ( 'NONE', *, *, #10838, .F. ) ;
#909=VECTOR ( 'NONE', #11459, 1000.000000000000000 ) ;
#910=ORIENTED_EDGE ( 'NONE', *, *, #13189, .T. ) ;
#915=DIRECTION ( 'NONE',  ( 8.018662683283438208E-16, -5.975035461963189015E-16, -1.000000000000000000 ) ) ;
#916=CARTESIAN_POINT ( 'NONE',  ( -15.34686821047329808, -23.48120812104550481, 57.00231026484399166 ) ) ;
#917=VECTOR ( 'NONE', #12215, 1000.000000000000000 ) ;
#918=EDGE_CURVE ( 'NONE', #15017, #6821, #3177, .T. ) ;
#921=CARTESIAN_POINT ( 'NONE',  ( -7.785174720008381399, -8.727488632615573394, 56.85231026484400019 ) ) ;
#922=LINE ( 'NONE', #7863, #14085 ) ;
#924=AXIS2_PLACEMENT_3D ( 'NONE', #9119, #4238, #5750 ) ;
#926=DIRECTION ( 'NONE',  ( 0.8772189822852964891, -0.4800904676395362780, 9.902680687415700047E-16 ) ) ;
#928=ORIENTED_EDGE ( 'NONE', *, *, #12469, .F. ) ;
#931=DIRECTION ( 'NONE',  ( 8.018662683283438208E-16, -5.975035461963189015E-16, -1.000000000000000000 ) ) ;
#932=ORIENTED_EDGE ( 'NONE', *, *, #12744, .T. ) ;
#934=EDGE_CURVE ( 'NONE', #6732, #13413, #5465, .T. ) ;
#936=EDGE_CURVE ( 'NONE', #12614, #1243, #12290, .T. ) ;
#937=EDGE_LOOP ( 'NONE', ( #1043, #14759, #7080, #4736 ) ) ;
#940=AXIS2_PLACEMENT_3D ( 'NONE', #10481, #5955, #3518 ) ;
#943=ORIENTED_EDGE ( 'NONE', *, *, #194, .F. ) ;
#949=ORIENTED_EDGE ( 'NONE', *, *, #5249, .F. ) ;
#950=PLANE ( 'NONE',  #12385 ) ;
#951=VERTEX_POINT ( 'NONE', #12745 ) ;
#955=ADVANCED_FACE ( 'NONE', ( #11434 ), #13956, .F. ) ;
#956=ORIENTED_EDGE ( 'NONE', *, *, #1466, .F. ) ;
#964=VERTEX_POINT ( 'NONE', #3327 ) ;
#965=PLANE ( 'NONE',  #1419 ) ;
#966=AXIS2_PLACEMENT_3D ( 'NONE', #3927, #561, #13271 ) ;
#968=EDGE_LOOP ( 'NONE', ( #5953, #3847, #10193, #5384 ) ) ;
#972=DIRECTION ( 'NONE',  ( -8.018662683283438208E-16, 5.975035461963189015E-16, 1.000000000000000000 ) ) ;
#976=LINE ( 'NONE', #4567, #14165 ) ;
#979=EDGE_CURVE ( 'NONE', #13413, #2196, #9368, .T. ) ;
#982=AXIS2_PLACEMENT_3D ( 'NONE', #10415, #14932, #7803 ) ;
#983=ORIENTED_EDGE ( 'NONE', *, *, #9725, .T. ) ;
#985=( BOUNDED_CURVE ( )  B_SPLINE_CURVE ( 3, ( #10218, #8919, #14893, #13522 ),
 .UNSPECIFIED., .F., .T. ) 
 B_SPLINE_CURVE_WITH_KNOTS ( ( 4, 4 ),
 ( 3.141592653589792672, 4.712388980384689674 ),
 .UNSPECIFIED. ) 
 CURVE ( )  GEOMETRIC_REPRESENTATION_ITEM ( )  RATIONAL_B_SPLINE_CURVE ( ( 1.000000000000000000, 0.8047378541243649375, 0.8047378541243649375, 1.000000000000000000 ) ) 
 REPRESENTATION_ITEM ( '' )  );
#987=DIRECTION ( 'NONE',  ( -8.018662683283438208E-16, 5.975035461963189015E-16, 1.000000000000000000 ) ) ;
#988=PLANE ( 'NONE',  #14150 ) ;
#989=ORIENTED_EDGE ( 'NONE', *, *, #11826, .F. ) ;
#990=EDGE_LOOP ( 'NONE', ( #3817, #11633, #11103, #5759 ) ) ;
#991=DIRECTION ( 'NONE',  ( 0.1165201156931293391, 0.9931883319083343320, -4.999999999999998416E-16 ) ) ;
#993=AXIS2_PLACEMENT_3D ( 'NONE', #8792, #10014, #8719 ) ;
#995=CARTESIAN_POINT ( 'NONE',  ( -24.53816276005083452, -12.69040994830970703, 57.00231026484397745 ) ) ;
#999=DIRECTION ( 'NONE',  ( 8.018662683283438208E-16, -5.975035461963189015E-16, -1.000000000000000000 ) ) ;
#1003=VERTEX_POINT ( 'NONE', #11587 ) ;
#1004=CARTESIAN_POINT ( 'NONE',  ( -22.70654572567255869, -20.40389968624657513, 57.00231026484397745 ) ) ;
#1005=LINE ( 'NONE', #6798, #579 ) ;
#1009=ORIENTED_EDGE ( 'NONE', *, *, #2438, .T. ) ;
#1010=CARTESIAN_POINT ( 'NONE',  ( -23.43263029221230198, -15.01730109988151440, 57.00231026484397745 ) ) ;
#1014=ORIENTED_EDGE ( 'NONE', *, *, #11151, .F. ) ;
#1017=ORIENTED_EDGE ( 'NONE', *, *, #13083, .T. ) ;
#1018=CARTESIAN_POINT ( 'NONE',  ( -11.30335942247960546, -22.55676305576680818, 56.85231026484400019 ) ) ;
#1020=LINE ( 'NONE', #3317, #4324 ) ;
#1021=VERTEX_POINT ( 'NONE', #6832 ) ;
#1022=VERTEX_POINT ( 'NONE', #5762 ) ;
#1023=PLANE ( 'NONE',  #4211 ) ;
#1029=DIRECTION ( 'NONE',  ( 8.018662683283438208E-16, -5.975035461963189015E-16, -1.000000000000000000 ) ) ;
#1031=LINE ( 'NONE', #3474, #9523 ) ;
#1034=ADVANCED_FACE ( 'NONE', ( #4550 ), #10434, .T. ) ;
#1035=ADVANCED_FACE ( 'NONE', ( #13129 ), #9671, .T. ) ;
#1037=PLANE ( 'NONE',  #13732 ) ;
#1038=LINE ( 'NONE', #13736, #15097 ) ;
#1039=VERTEX_POINT ( 'NONE', #9593 ) ;
#1041=DIRECTION ( 'NONE',  ( -8.018662683283439195E-16, 5.975035461963190001E-16, 1.000000000000000000 ) ) ;
#1043=ORIENTED_EDGE ( 'NONE', *, *, #1994, .T. ) ;
#1044=DIRECTION ( 'NONE',  ( 8.018662683283438208E-16, -5.975035461963189015E-16, -1.000000000000000000 ) ) ;
#1048=CARTESIAN_POINT ( 'NONE',  ( -5.524802968312260809, -13.55273297815670119, 57.00231026484399166 ) ) ;
#1049=VECTOR ( 'NONE', #12327, 999.9999999999998863 ) ;
#1057=DIRECTION ( 'NONE',  ( -0.5691548339926012501, -0.8222303661035965661, 3.489949670251134954E-17 ) ) ;
#1059=CARTESIAN_POINT ( 'NONE',  ( -15.49969986081092088, -13.50737899243822504, 57.00231026484397745 ) ) ;
#1060=ORIENTED_EDGE ( 'NONE', *, *, #211, .F. ) ;
#1061=DIRECTION ( 'NONE',  ( -0.9918751611018178371, -0.1272150336605033238, -7.193398003386547388E-16 ) ) ;
#1062=ORIENTED_EDGE ( 'NONE', *, *, #6172, .F. ) ;
#1063=LINE ( 'NONE', #4812, #9093 ) ;
#1065=EDGE_CURVE ( 'NONE', #3619, #10638, #2411, .T. ) ;
#1066=VECTOR ( 'NONE', #11148, 1000.000000000000114 ) ;
#1069=DIRECTION ( 'NONE',  ( 8.018662683283438208E-16, -5.975035461963189015E-16, -1.000000000000000000 ) ) ;
#1070=LINE ( 'NONE', #6640, #9198 ) ;
#1073=DIRECTION ( 'NONE',  ( 0.5196486895212314439, -0.8543800322332368857, 9.271838545667882647E-16 ) ) ;
#1074=CIRCLE ( 'NONE', #5710, 9.974999999999999645 ) ;
#1075=CARTESIAN_POINT ( 'NONE',  ( -12.81093390292747713, -9.898980784960684787, 46.00231026484398456 ) ) ;
#1076=ORIENTED_EDGE ( 'NONE', *, *, #13342, .T. ) ;
#1083=VERTEX_POINT ( 'NONE', #11813 ) ;
#1085=EDGE_CURVE ( 'NONE', #13264, #8564, #9747, .T. ) ;
#1086=CARTESIAN_POINT ( 'NONE',  ( -22.55857771067089246, -13.99059064457067336, 57.00231026484397745 ) ) ;
#1087=VECTOR ( 'NONE', #14752, 1000.000000000000000 ) ;
#1088=DIRECTION ( 'NONE',  ( -0.9085715390340232123, 0.4177292884839972631, -9.781476007338056784E-16 ) ) ;
#1090=ORIENTED_EDGE ( 'NONE', *, *, #13626, .T. ) ;
#1095=ORIENTED_EDGE ( 'NONE', *, *, #8887, .F. ) ;
#1096=STYLED_ITEM ( 'NONE', ( #2295 ), #7285 ) ;
#1098=EDGE_LOOP ( 'NONE', ( #10426, #1549, #6086, #13428 ) ) ;
#1106=LINE ( 'NONE', #1413, #14279 ) ;
#1110=ORIENTED_EDGE ( 'NONE', *, *, #4, .F. ) ;
#1114=CARTESIAN_POINT ( 'NONE',  ( -8.701256315749452241, -15.46758698257906950, 56.85231026484400019 ) ) ;
#1115=ORIENTED_EDGE ( 'NONE', *, *, #13289, .T. ) ;
#1116=CARTESIAN_POINT ( 'NONE',  ( -22.80943503306988873, -20.29474937510043375, 54.00231026484399166 ) ) ;
#1118=EDGE_CURVE ( 'NONE', #13967, #642, #123, .T. ) ;
#1120=CARTESIAN_POINT ( 'NONE',  ( -7.731023390221355207, -11.30308411758414877, 57.00231026484399166 ) ) ;
#1122=CARTESIAN_POINT ( 'NONE',  ( -15.49969986081092088, -13.50737899243822504, 57.00231026484397745 ) ) ;
#1123=CARTESIAN_POINT ( 'NONE',  ( -24.21370508435883906, -8.652820519829269585, 57.00231026484397745 ) ) ;
#1129=ORIENTED_EDGE ( 'NONE', *, *, #13105, .F. ) ;
#1134=EDGE_CURVE ( 'NONE', #13353, #11163, #4261, .T. ) ;
#1138=CARTESIAN_POINT ( 'NONE',  ( -15.16333526000375187, -10.64029123852186132, 56.75231026484397745 ) ) ;
#1139=DIRECTION ( 'NONE',  ( 0.5975035461963189576, 0.8018662683283437342, 0.000000000000000000 ) ) ;
#1142=CARTESIAN_POINT ( 'NONE',  ( -15.12053853660593283, -5.441285657357897598, 56.85231026484398598 ) ) ;
#1146=VERTEX_POINT ( 'NONE', #1489 ) ;
#1147=CARTESIAN_POINT ( 'NONE',  ( -19.55678615628314532, -20.48959216528617233, 56.85231026484398598 ) ) ;
#1152=ORIENTED_EDGE ( 'NONE', *, *, #4117, .T. ) ;
#1153=VECTOR ( 'NONE', #6236, 999.9999999999998863 ) ;
#1158=VECTOR ( 'NONE', #12137, 999.9999999999998863 ) ;
#1165=VERTEX_POINT ( 'NONE', #10822 ) ;
#1167=ORIENTED_EDGE ( 'NONE', *, *, #4732, .F. ) ;
#1168=CARTESIAN_POINT ( 'NONE',  ( -15.49969986081091378, -13.50737899243822859, 51.00231026484399166 ) ) ;
#1169=ORIENTED_EDGE ( 'NONE', *, *, #6172, .T. ) ;
#1171=LINE ( 'NONE', #1402, #14226 ) ;
#1173=CONICAL_SURFACE ( 'NONE', #7510, 5.000000000000000000, 0.7853981633974476129 ) ;
#1175=CARTESIAN_POINT ( 'NONE',  ( -5.650856670168512785, -15.08880645082408556, 57.00231026484399166 ) ) ;
#1177=VECTOR ( 'NONE', #10955, 1000.000000000000227 ) ;
#1181=ADVANCED_FACE ( 'NONE', ( #2709 ), #10664, .F. ) ;
#1186=CARTESIAN_POINT ( 'NONE',  ( -24.39712111458418775, -18.01698208283363556, 54.00231026484399166 ) ) ;
#1187=DIRECTION ( 'NONE',  ( -0.5975035461963188466, -0.8018662683283439563, 0.000000000000000000 ) ) ;
#1188=ORIENTED_EDGE ( 'NONE', *, *, #5624, .T. ) ;
#1190=CARTESIAN_POINT ( 'NONE',  ( -7.064541492512758758, -18.83173137575486678, 54.00231026484400587 ) ) ;
#1192=DIRECTION ( 'NONE',  ( -8.018662683283438208E-16, 5.975035461963189015E-16, 1.000000000000000000 ) ) ;
#1195=ORIENTED_EDGE ( 'NONE', *, *, #11513, .T. ) ;
#1200=LINE ( 'NONE', #13754, #10653 ) ;
#1201=EDGE_CURVE ( 'NONE', #12600, #10787, #12478, .T. ) ;
#1207=EDGE_CURVE ( 'NONE', #9069, #118, #5432, .T. ) ;
#1209=ORIENTED_EDGE ( 'NONE', *, *, #3266, .T. ) ;
#1211=ORIENTED_EDGE ( 'NONE', *, *, #1496, .F. ) ;
#1212=FACE_BOUND ( 'NONE', #878, .T. ) ;
#1214=ADVANCED_FACE ( 'NONE', ( #7439 ), #9097, .F. ) ;
#1215=CIRCLE ( 'NONE', #11469, 9.974999999999999645 ) ;
#1216=CARTESIAN_POINT ( 'NONE',  ( -17.12834591918736749, -6.622385381944812188, 56.85231026484398598 ) ) ;
#1217=SURFACE_SIDE_STYLE ('',( #13995 ) ) ;
#1218=CARTESIAN_POINT ( 'NONE',  ( -18.86735971344653962, -5.080035572537331845, 57.00231026484397745 ) ) ;
#1226=DIRECTION ( 'NONE',  ( 0.5975035461963188466, 0.8018662683283437342, 0.000000000000000000 ) ) ;
#1227=ORIENTED_EDGE ( 'NONE', *, *, #3624, .T. ) ;
#1228=CARTESIAN_POINT ( 'NONE',  ( -19.45253106704483770, -6.466019006254929202, 56.85231026484398598 ) ) ;
#1230=ORIENTED_EDGE ( 'NONE', *, *, #13605, .F. ) ;
#1232=CARTESIAN_POINT ( 'NONE',  ( -23.12048770254168062, -16.17743848078839619, 56.85231026484398598 ) ) ;
#1233=ORIENTED_EDGE ( 'NONE', *, *, #9921, .T. ) ;
#1234=CARTESIAN_POINT ( 'NONE',  ( -12.84854673063649599, -12.36513540471286809, 51.25231026484399166 ) ) ;
#1236=CARTESIAN_POINT ( 'NONE',  ( -7.285742840713465007, -17.36641515085804599, 56.85231026484400019 ) ) ;
#1239=CYLINDRICAL_SURFACE ( 'NONE', #3766, 0.2500000000000004441 ) ;
#1240=DIRECTION ( 'NONE',  ( -0.5975035461963188466, -0.8018662683283439563, 0.000000000000000000 ) ) ;
#1243=VERTEX_POINT ( 'NONE', #2148 ) ;
#1244=ORIENTED_EDGE ( 'NONE', *, *, #4054, .F. ) ;
#1245=ORIENTED_EDGE ( 'NONE', *, *, #14708, .T. ) ;
#1246=DIRECTION ( 'NONE',  ( 0.7276687409742212953, 0.6859287159822015090, 1.736481776669299976E-16 ) ) ;
#1248=AXIS2_PLACEMENT_3D ( 'NONE', #13525, #7691, #12375 ) ;
#1250=EDGE_CURVE ( 'NONE', #1699, #13647, #7714, .T. ) ;
#1253=AXIS2_PLACEMENT_3D ( 'NONE', #8330, #166, #9328 ) ;
#1254=DIRECTION ( 'NONE',  ( 8.018662683283438208E-16, -5.975035461963189015E-16, -1.000000000000000000 ) ) ;
#1256=CARTESIAN_POINT ( 'NONE',  ( -19.87664613915258371, -5.557310358991672139, 57.00231026484397745 ) ) ;
#1258=FACE_OUTER_BOUND ( 'NONE', #72, .T. ) ;
#1269=ADVANCED_FACE ( 'NONE', ( #12632 ), #4370, .F. ) ;
#1271=LINE ( 'NONE', #10840, #12360 ) ;
#1272=PLANE ( 'NONE',  #15007 ) ;
#1273=VECTOR ( 'NONE', #11597, 1000.000000000000114 ) ;
#1274=ORIENTED_EDGE ( 'NONE', *, *, #14320, .F. ) ;
#1275=CARTESIAN_POINT ( 'NONE',  ( -17.72286745096104355, -3.783277446994212312, 54.00231026484397745 ) ) ;
#1276=AXIS2_PLACEMENT_3D ( 'NONE', #1608, #11091, #13328 ) ;
#1277=LINE ( 'NONE', #5937, #679 ) ;
#1280=AXIS2_PLACEMENT_3D ( 'NONE', #7638, #12245, #11247 ) ;
#1283=DIRECTION ( 'NONE',  ( -0.02283895005206026604, 0.9997391571607663341, -6.156614753256598861E-16 ) ) ;
#1285=CARTESIAN_POINT ( 'NONE',  ( -7.425287632467987287, -13.60480674405941492, 56.85231026484400019 ) ) ;
#1287=CARTESIAN_POINT ( 'NONE',  ( -22.04595456446742929, -18.23578246029658345, 56.85231026484398598 ) ) ;
#1288=ADVANCED_FACE ( 'NONE', ( #4217 ), #8871, .T. ) ;
#1289=LINE ( 'NONE', #9629, #10065 ) ;
#1291=VECTOR ( 'NONE', #13358, 1000.000000000000000 ) ;
#1292=VECTOR ( 'NONE', #13779, 1000.000000000000114 ) ;
#1295=FACE_OUTER_BOUND ( 'NONE', #14589, .T. ) ;
#1296=ORIENTED_EDGE ( 'NONE', *, *, #7957, .T. ) ;
#1298=LINE ( 'NONE', #8326, #6779 ) ;
#1299=LINE ( 'NONE', #4670, #10833 ) ;
#1300=ORIENTED_EDGE ( 'NONE', *, *, #5722, .T. ) ;
#1301=PLANE ( 'NONE',  #14942 ) ;
#1304=ADVANCED_FACE ( 'NONE', ( #13776 ), #6715, .F. ) ;
#1305=FACE_OUTER_BOUND ( 'NONE', #8694, .T. ) ;
#1306=ORIENTED_EDGE ( 'NONE', *, *, #5188, .T. ) ;
#1310=DIRECTION ( 'NONE',  ( 0.8018662683283436232, -0.5975035461963189576, 9.999999999999996833E-16 ) ) ;
#1313=CARTESIAN_POINT ( 'NONE',  ( -23.36093307149983289, -11.66014798166512634, 57.00231026484397745 ) ) ;
#1315=EDGE_CURVE ( 'NONE', #10582, #1699, #3140, .T. ) ;
#1316=LINE ( 'NONE', #8419, #6466 ) ;
#1318=CARTESIAN_POINT ( 'NONE',  ( -21.67659902633306146, -21.33978230808610022, 56.85231026484398598 ) ) ;
#1320=CARTESIAN_POINT ( 'NONE',  ( -18.15085299098534222, -14.64962258016358732, 56.89875687425072215 ) ) ;
#1323=FACE_OUTER_BOUND ( 'NONE', #14535, .T. ) ;
#1325=VERTEX_POINT ( 'NONE', #5577 ) ;
#1328=ORIENTED_EDGE ( 'NONE', *, *, #3030, .T. ) ;
#1329=ORIENTED_EDGE ( 'NONE', *, *, #11138, .T. ) ;
#1330=DIRECTION ( 'NONE',  ( -8.018662683283438208E-16, 5.975035461963189015E-16, 1.000000000000000000 ) ) ;
#1331=ORIENTED_EDGE ( 'NONE', *, *, #3928, .F. ) ;
#1332=CARTESIAN_POINT ( 'NONE',  ( -10.84210729886283531, -6.910555398701176522, 57.00231026484397745 ) ) ;
#1333=VECTOR ( 'NONE', #8633, 1000.000000000000000 ) ;
#1341=ORIENTED_EDGE ( 'NONE', *, *, #13293, .F. ) ;
#1344=ORIENTED_EDGE ( 'NONE', *, *, #13456, .T. ) ;
#1345=ORIENTED_EDGE ( 'NONE', *, *, #2264, .F. ) ;
#1347=ADVANCED_FACE ( 'NONE', ( #3932 ), #13278, .T. ) ;
#1349=VERTEX_POINT ( 'NONE', #1375 ) ;
#1350=DIRECTION ( 'NONE',  ( -0.9983330752162417054, -0.05771543059946733500, -7.660444431189781397E-16 ) ) ;
#1351=VECTOR ( 'NONE', #1366, 1000.000000000000000 ) ;
#1352=PLANE ( 'NONE',  #3170 ) ;
#1354=PLANE ( 'NONE',  #15041 ) ;
#1355=PLANE ( 'NONE',  #3232 ) ;
#1357=CARTESIAN_POINT ( 'NONE',  ( -12.38873450203231030, -7.152605626181999909, 56.85231026484398598 ) ) ;
#1360=ADVANCED_FACE ( 'NONE', ( #7094 ), #4521, .F. ) ;
#1361=DIRECTION ( 'NONE',  ( -8.018662683283438208E-16, 5.975035461963189015E-16, 1.000000000000000000 ) ) ;
#1363=LINE ( 'NONE', #8314, #10601 ) ;
#1364=ORIENTED_EDGE ( 'NONE', *, *, #8217, .F. ) ;
#1366=DIRECTION ( 'NONE',  ( 8.018662683283438208E-16, -5.975035461963189015E-16, -1.000000000000000000 ) ) ;
#1368=FILL_AREA_STYLE ('',( #14149 ) ) ;
#1370=CARTESIAN_POINT ( 'NONE',  ( -9.251715890255169938, -8.391880844292892050, 57.00231026484397745 ) ) ;
#1371=VECTOR ( 'NONE', #14303, 1000.000000000000000 ) ;
#1372=LINE ( 'NONE', #14229, #10895 ) ;
#1374=DIRECTION ( 'NONE',  ( -8.018662683283438208E-16, 5.975035461963189015E-16, 1.000000000000000000 ) ) ;
#1375=CARTESIAN_POINT ( 'NONE',  ( -7.480766807389218620, -12.55450823271226746, 57.00231026484399166 ) ) ;
#1377=EDGE_CURVE ( 'NONE', #1475, #9010, #11552, .T. ) ;
#1378=VERTEX_POINT ( 'NONE', #84 ) ;
#1381=ORIENTED_EDGE ( 'NONE', *, *, #12726, .T. ) ;
#1383=EDGE_CURVE ( 'NONE', #7657, #9919, #8251, .T. ) ;
#1384=DIRECTION ( 'NONE',  ( 8.018662683283438208E-16, -5.975035461963189015E-16, -1.000000000000000000 ) ) ;
#1387=FACE_OUTER_BOUND ( 'NONE', #203, .T. ) ;
#1390=LINE ( 'NONE', #14017, #1912 ) ;
#1392=AXIS2_PLACEMENT_3D ( 'NONE', #13825, #830, #8925 ) ;
#1394=EDGE_CURVE ( 'NONE', #11477, #118, #11776, .T. ) ;
#1396=EDGE_CURVE ( 'NONE', #5861, #745, #8020, .T. ) ;
#1402=CARTESIAN_POINT ( 'NONE',  ( -22.54723635769173384, -9.564857042577559199, 56.85231026484398598 ) ) ;
#1403=ORIENTED_EDGE ( 'NONE', *, *, #11594, .F. ) ;
#1404=DIRECTION ( 'NONE',  ( -8.018662683283438208E-16, 5.975035461963189015E-16, 1.000000000000000000 ) ) ;
#1405=LINE ( 'NONE', #3849, #8849 ) ;
#1407=EDGE_CURVE ( 'NONE', #2678, #8358, #1298, .T. ) ;
#1408=CARTESIAN_POINT ( 'NONE',  ( -14.07534335717186202, -5.558639560896826204, 56.85231026484398598 ) ) ;
#1409=CIRCLE ( 'NONE', #4101, 9.974999999999999645 ) ;
#1410=LINE ( 'NONE', #6059, #7036 ) ;
#1411=DIRECTION ( 'NONE',  ( -8.018662683283438208E-16, 5.975035461963189015E-16, 1.000000000000000000 ) ) ;
#1413=CARTESIAN_POINT ( 'NONE',  ( -8.667632128016617088, -19.48099602858229318, 57.00231026484399166 ) ) ;
#1416=CARTESIAN_POINT ( 'NONE',  ( -15.49969986081092088, -13.50737899243822504, 56.85231026484398598 ) ) ;
#1419=AXIS2_PLACEMENT_3D ( 'NONE', #5617, #10131, #3181 ) ;
#1420=CARTESIAN_POINT ( 'NONE',  ( -8.791486474964735010, -6.124933722071896014, 57.00231026484397745 ) ) ;
#1421=ORIENTED_EDGE ( 'NONE', *, *, #8034, .T. ) ;
#1425=CARTESIAN_POINT ( 'NONE',  ( -11.30335942247960190, -22.55676305576680818, 54.00231026484399166 ) ) ;
#1433=DIRECTION ( 'NONE',  ( -8.018662683283439195E-16, 5.975035461963190001E-16, 1.000000000000000000 ) ) ;
#1436=PLANE ( 'NONE',  #6755 ) ;
#1437=FACE_OUTER_BOUND ( 'NONE', #183, .T. ) ;
#1440=DIRECTION ( 'NONE',  ( -8.018662683283439195E-16, 5.975035461963190001E-16, 1.000000000000000000 ) ) ;
#1441=ORIENTED_EDGE ( 'NONE', *, *, #7113, .T. ) ;
#1443=ORIENTED_EDGE ( 'NONE', *, *, #5114, .T. ) ;
#1448=ADVANCED_FACE ( 'NONE', ( #1453 ), #1173, .T. ) ;
#1449=FACE_OUTER_BOUND ( 'NONE', #11049, .T. ) ;
#1451=VERTEX_POINT ( 'NONE', #9863 ) ;
#1453=FACE_OUTER_BOUND ( 'NONE', #7463, .T. ) ;
#1454=PLANE ( 'NONE',  #7150 ) ;
#1455=VERTEX_POINT ( 'NONE', #13243 ) ;
#1460=VERTEX_POINT ( 'NONE', #14530 ) ;
#1461=ORIENTED_EDGE ( 'NONE', *, *, #1671, .T. ) ;
#1462=VECTOR ( 'NONE', #2494, 1000.000000000000000 ) ;
#1463=DIRECTION ( 'NONE',  ( -0.3533329742249643468, -0.9354976265738683683, 2.756373558169988451E-16 ) ) ;
#1466=EDGE_CURVE ( 'NONE', #2901, #8324, #6287, .T. ) ;
#1467=DIRECTION ( 'NONE',  ( 0.5975035461963188466, 0.8018662683283437342, 0.000000000000000000 ) ) ;
#1470=DIRECTION ( 'NONE',  ( -0.02283895005205794151, 0.9997391571607663341, -6.156614753256579139E-16 ) ) ;
#1472=ORIENTED_EDGE ( 'NONE', *, *, #4194, .T. ) ;
#1475=VERTEX_POINT ( 'NONE', #8636 ) ;
#1476=( BOUNDED_CURVE ( )  B_SPLINE_CURVE ( 3, ( #1533, #8487, #10714, #242 ),
 .UNSPECIFIED., .F., .T. ) 
 B_SPLINE_CURVE_WITH_KNOTS ( ( 4, 4 ),
 ( -8.881784197001252323E-16, 1.570796326794895670 ),
 .UNSPECIFIED. ) 
 CURVE ( )  GEOMETRIC_REPRESENTATION_ITEM ( )  RATIONAL_B_SPLINE_CURVE ( ( 1.000000000000000000, 0.8047378541243649375, 0.8047378541243649375, 1.000000000000000000 ) ) 
 REPRESENTATION_ITEM ( '' )  );
#1477=LINE ( 'NONE', #13191, #12443 ) ;
#1478=ORIENTED_EDGE ( 'NONE', *, *, #10848, .F. ) ;
#1481=ORIENTED_EDGE ( 'NONE', *, *, #1803, .T. ) ;
#1482=CARTESIAN_POINT ( 'NONE',  ( -8.681233859935403530, -6.226640953275949464, 54.00231026484399166 ) ) ;
#1483=CARTESIAN_POINT ( 'NONE',  ( -6.424455519809837867, -13.54187755947681993, 56.85231026484400019 ) ) ;
#1484=EDGE_CURVE ( 'NONE', #3312, #4359, #4097, .T. ) ;
#1489=CARTESIAN_POINT ( 'NONE',  ( -19.27841348868324545, -22.73895244004356897, 56.85231026484400019 ) ) ;
#1491=DIRECTION ( 'NONE',  ( -8.018662683283438208E-16, 5.975035461963189015E-16, 1.000000000000000000 ) ) ;
#1496=EDGE_CURVE ( 'NONE', #11960, #951, #7556, .T. ) ;
#1497=EDGE_LOOP ( 'NONE', ( #9660, #8651, #10886, #469 ) ) ;
#1498=DIRECTION ( 'NONE',  ( 0.7276687409742212953, 0.6859287159822015090, 1.736481776669299976E-16 ) ) ;
#1499=ORIENTED_EDGE ( 'NONE', *, *, #15040, .F. ) ;
#1501=EDGE_CURVE ( 'NONE', #2831, #10753, #529, .T. ) ;
#1504=AXIS2_PLACEMENT_3D ( 'NONE', #14260, #6843, #10451 ) ;
#1510=PLANE ( 'NONE',  #3630 ) ;
#1511=ORIENTED_EDGE ( 'NONE', *, *, #2712, .F. ) ;
#1512=VECTOR ( 'NONE', #8602, 1000.000000000000227 ) ;
#1517=DIRECTION ( 'NONE',  ( 8.018662683283438208E-16, -5.975035461963189015E-16, -1.000000000000000000 ) ) ;
#1519=FACE_OUTER_BOUND ( 'NONE', #6294, .T. ) ;
#1521=EDGE_CURVE ( 'NONE', #14564, #3602, #10864, .T. ) ;
#1525=VECTOR ( 'NONE', #13691, 1000.000000000000000 ) ;
#1532=ORIENTED_EDGE ( 'NONE', *, *, #14867, .T. ) ;
#1533=CARTESIAN_POINT ( 'NONE',  ( -17.81448839017816965, -11.78253482624722182, 56.75231026484397745 ) ) ;
#1534=EDGE_LOOP ( 'NONE', ( #4719, #13247, #10313, #11778 ) ) ;
#1535=EDGE_CURVE ( 'NONE', #413, #14491, #6253, .T. ) ;
#1540=AXIS2_PLACEMENT_3D ( 'NONE', #1483, #9361, #14033 ) ;
#1541=CARTESIAN_POINT ( 'NONE',  ( -11.16775676328319200, -22.49263881059494707, 56.85231026484400019 ) ) ;
#1542=DIRECTION ( 'NONE',  ( -8.018662683283438208E-16, 5.975035461963189015E-16, 1.000000000000000000 ) ) ;
#1544=CARTESIAN_POINT ( 'NONE',  ( -5.898712304418589625, -10.80152183767200214, 56.85231026484400019 ) ) ;
#1549=ORIENTED_EDGE ( 'NONE', *, *, #5722, .F. ) ;
#1550=CARTESIAN_POINT ( 'NONE',  ( -11.55178736972959008, -19.37894070656199474, 57.00231026484399166 ) ) ;
#1554=EDGE_CURVE ( 'NONE', #12810, #14661, #10938, .T. ) ;
#1558=FACE_OUTER_BOUND ( 'NONE', #9767, .T. ) ;
#1560=LINE ( 'NONE', #1630, #4366 ) ;
#1562=DIRECTION ( 'NONE',  ( -8.018662683283439195E-16, 5.975035461963190001E-16, 1.000000000000000000 ) ) ;
#1563=DIRECTION ( 'NONE',  ( 0.5975035461963189576, 0.8018662683283437342, 0.000000000000000000 ) ) ;
#1564=CARTESIAN_POINT ( 'NONE',  ( -20.00744539586189319, -5.630737564061013778, 56.85231026484398598 ) ) ;
#1568=VERTEX_POINT ( 'NONE', #14826 ) ;
#1571=EDGE_CURVE ( 'NONE', #13071, #7355, #12161, .T. ) ;
#1572=CARTESIAN_POINT ( 'NONE',  ( -24.88854884048805971, -16.87637585156647191, 57.00231026484397745 ) ) ;
#1573=ORIENTED_EDGE ( 'NONE', *, *, #10585, .T. ) ;
#1574=EDGE_CURVE ( 'NONE', #2365, #4448, #9080, .T. ) ;
#1577=CARTESIAN_POINT ( 'NONE',  ( -24.32830346761242879, -18.15026423267100597, 57.00231026484397745 ) ) ;
#1578=CARTESIAN_POINT ( 'NONE',  ( -24.93814746875458610, -16.73481322911949931, 54.00231026484397745 ) ) ;
#1580=DIRECTION ( 'NONE',  ( -0.6780482080269577549, -0.7350174335289139105, -1.045284632676540317E-16 ) ) ;
#1582=VERTEX_POINT ( 'NONE', #3280 ) ;
#1584=CARTESIAN_POINT ( 'NONE',  ( -23.40321606353253614, -15.16438883951732741, 56.85231026484398598 ) ) ;
#1586=DIRECTION ( 'NONE',  ( 0.5975035461963189576, 0.8018662683283437342, 0.000000000000000000 ) ) ;
#1588=PLANE ( 'NONE',  #7166 ) ;
#1594=CARTESIAN_POINT ( 'NONE',  ( -17.72867398697626129, -22.30470383268854562, 56.85231026484400019 ) ) ;
#1595=DIRECTION ( 'NONE',  ( -0.9225966037272086417, 0.3857661296576204712, -9.702957262759976898E-16 ) ) ;
#1596=PLANE ( 'NONE',  #9628 ) ;
#1600=ORIENTED_EDGE ( 'NONE', *, *, #3069, .F. ) ;
#1601=CARTESIAN_POINT ( 'NONE',  ( -8.667632128016617088, -19.48099602858229318, 56.85231026484400019 ) ) ;
#1603=EDGE_CURVE ( 'NONE', #2842, #10291, #8931, .T. ) ;
#1604=ORIENTED_EDGE ( 'NONE', *, *, #7269, .F. ) ;
#1606=VERTEX_POINT ( 'NONE', #14906 ) ;
#1608=CARTESIAN_POINT ( 'NONE',  ( -15.49969986081092088, -13.50737899243822504, 57.00231026484397745 ) ) ;
#1611=VECTOR ( 'NONE', #14316, 1000.000000000000114 ) ;
#1612=DIRECTION ( 'NONE',  ( -8.018662683283438208E-16, 5.975035461963189015E-16, 1.000000000000000000 ) ) ;
#1617=EDGE_CURVE ( 'NONE', #7427, #6732, #1277, .T. ) ;
#1619=CARTESIAN_POINT ( 'NONE',  ( -23.42445533997705454, -9.084766574938008432, 57.00231026484397745 ) ) ;
#1623=LINE ( 'NONE', #14403, #9014 ) ;
#1630=CARTESIAN_POINT ( 'NONE',  ( -9.291286065451624054, -6.887949398765353060, 57.00231026484397745 ) ) ;
#1631=AXIS2_PLACEMENT_3D ( 'NONE', #14464, #1542, #13474 ) ;
#1632=EDGE_CURVE ( 'NONE', #2532, #6446, #6775, .T. ) ;
#1639=ORIENTED_EDGE ( 'NONE', *, *, #12846, .F. ) ;
#1640=LINE ( 'NONE', #10596, #10649 ) ;
#1646=CARTESIAN_POINT ( 'NONE',  ( -23.37741044072812713, -11.73331557219068877, 57.00231026484397745 ) ) ;
#1654=CARTESIAN_POINT ( 'NONE',  ( -13.74242962142780478, -4.603826257390357668, 56.85231026484398598 ) ) ;
#1655=AXIS2_PLACEMENT_3D ( 'NONE', #14779, #707, #9031 ) ;
#1660=APPLICATION_CONTEXT ( 'automotive_design' ) ;
#1663=FACE_OUTER_BOUND ( 'NONE', #12423, .T. ) ;
#1664=VECTOR ( 'NONE', #5646, 1000.000000000000000 ) ;
#1665=DIRECTION ( 'NONE',  ( -8.018662683283438208E-16, 5.975035461963189015E-16, 1.000000000000000000 ) ) ;
#1666=EDGE_CURVE ( 'NONE', #8353, #2842, #10464, .T. ) ;
#1667=CARTESIAN_POINT ( 'NONE',  ( -17.54662770128649285, -5.179934221328323929, 57.00231026484397745 ) ) ;
#1670=CARTESIAN_POINT ( 'NONE',  ( -15.49969986081091733, -13.50737899243822682, 54.00231026484399166 ) ) ;
#1671=EDGE_CURVE ( 'NONE', #3333, #15014, #7014, .T. ) ;
#1674=AXIS2_PLACEMENT_3D ( 'NONE', #4104, #3026, #11144 ) ;
#1675=CARTESIAN_POINT ( 'NONE',  ( -15.49969986081092088, -13.50737899243822504, 57.00231026484397745 ) ) ;
#1676=EDGE_LOOP ( 'NONE', ( #3977, #3251, #588, #13714 ) ) ;
#1681=ORIENTED_EDGE ( 'NONE', *, *, #7069, .T. ) ;
#1683=DIRECTION ( 'NONE',  ( -8.018662683283439195E-16, 5.975035461963190001E-16, 1.000000000000000000 ) ) ;
#1688=EDGE_CURVE ( 'NONE', #2290, #10422, #8075, .T. ) ;
#1690=DIRECTION ( 'NONE',  ( -8.018662683283439195E-16, 5.975035461963190001E-16, 1.000000000000000000 ) ) ;
#1696=ORIENTED_EDGE ( 'NONE', *, *, #1250, .T. ) ;
#1697=LINE ( 'NONE', #12108, #10242 ) ;
#1699=VERTEX_POINT ( 'NONE', #4805 ) ;
#1701=CARTESIAN_POINT ( 'NONE',  ( -19.19431052208641475, -4.241825740657185762, 56.85231026484398598 ) ) ;
#1703=CYLINDRICAL_SURFACE ( 'NONE', #2024, 4.499999999999999112 ) ;
#1704=AXIS2_PLACEMENT_3D ( 'NONE', #5318, #808, #4025 ) ;
#1706=CARTESIAN_POINT ( 'NONE',  ( -13.74242962142780478, -4.603826257390357668, 57.00231026484397745 ) ) ;
#1707=ADVANCED_FACE ( 'NONE', ( #5858 ), #4654, .F. ) ;
#1711=ORIENTED_EDGE ( 'NONE', *, *, #7591, .T. ) ;
#1713=ORIENTED_EDGE ( 'NONE', *, *, #288, .T. ) ;
#1718=ORIENTED_EDGE ( 'NONE', *, *, #227, .F. ) ;
#1719=CARTESIAN_POINT ( 'NONE',  ( -15.83606446161809167, -16.37446674635458521, 51.00231026484399166 ) ) ;
#1722=DIRECTION ( 'NONE',  ( 0.09252159378507134047, -0.9957106782009873536, 6.691306063588577540E-16 ) ) ;
#1726=FACE_OUTER_BOUND ( 'NONE', #5471, .T. ) ;
#1727=ORIENTED_EDGE ( 'NONE', *, *, #13289, .F. ) ;
#1729=DIRECTION ( 'NONE',  ( -0.04695496274985035828, -0.9988970074402867549, 5.591929034707432303E-16 ) ) ;
#1733=ORIENTED_EDGE ( 'NONE', *, *, #1808, .F. ) ;
#1734=DIRECTION ( 'NONE',  ( 0.1165201156931293391, 0.9931883319083343320, -4.999999999999998416E-16 ) ) ;
#1736=DIRECTION ( 'NONE',  ( 0.5975035461963189576, 0.8018662683283437342, 0.000000000000000000 ) ) ;
#1738=VECTOR ( 'NONE', #3700, 1000.000000000000227 ) ;
#1739=LINE ( 'NONE', #11076, #9021 ) ;
#1742=DIRECTION ( 'NONE',  ( 8.018662683283438208E-16, -5.975035461963189015E-16, -1.000000000000000000 ) ) ;
#1743=FACE_OUTER_BOUND ( 'NONE', #13369, .T. ) ;
#1744=ORIENTED_EDGE ( 'NONE', *, *, #4194, .F. ) ;
#1749=EDGE_LOOP ( 'NONE', ( #9395, #13866, #8340, #4658 ) ) ;
#1753=VERTEX_POINT ( 'NONE', #11682 ) ;
#1754=EDGE_CURVE ( 'NONE', #8324, #7478, #4887, .T. ) ;
#1757=ADVANCED_FACE ( 'NONE', ( #8542 ), #14434, .T. ) ;
#1759=DIRECTION ( 'NONE',  ( -8.018662683283438208E-16, 5.975035461963189015E-16, 1.000000000000000000 ) ) ;
#1762=AXIS2_PLACEMENT_3D ( 'NONE', #4116, #9853, #7473 ) ;
#1764=DIRECTION ( 'NONE',  ( 0.5975035461963217331, 0.8018662683283416248, 0.000000000000000000 ) ) ;
#1766=ADVANCED_FACE ( 'NONE', ( #7389 ), #6085, .T. ) ;
#1767=LINE ( 'NONE', #1619, #12286 ) ;
#1769=CARTESIAN_POINT ( 'NONE',  ( -15.49969986081086226, -13.50737899243826767, -13.49768973515600301 ) ) ;
#1770=AXIS2_PLACEMENT_3D ( 'NONE', #8491, #537, #4989 ) ;
#1772=LINE ( 'NONE', #12034, #5116 ) ;
#1773=DIRECTION ( 'NONE',  ( -8.018662683283438208E-16, 5.975035461963189015E-16, 1.000000000000000000 ) ) ;
#1774=ORIENTED_EDGE ( 'NONE', *, *, #7676, .T. ) ;
#1776=AXIS2_PLACEMENT_3D ( 'NONE', #10188, #5823, #5598 ) ;
#1778=DIRECTION ( 'NONE',  ( 0.1511109077013141899, 0.9885168150181791180, -4.694715627858909121E-16 ) ) ;
#1781=VERTEX_POINT ( 'NONE', #2584 ) ;
#1783=DIRECTION ( 'NONE',  ( -8.018662683283438208E-16, 5.975035461963189015E-16, 1.000000000000000000 ) ) ;
#1785=DIRECTION ( 'NONE',  ( -0.4177292884839868270, -0.9085715390340278752, 2.079116908177700458E-16 ) ) ;
#1786=DIRECTION ( 'NONE',  ( -8.018662683283438208E-16, 5.975035461963189015E-16, 1.000000000000000000 ) ) ;
#1789=CARTESIAN_POINT ( 'NONE',  ( -24.36945568363038461, -11.58678490633884373, 56.85231026484398598 ) ) ;
#1790=CARTESIAN_POINT ( 'NONE',  ( -22.61924992783766797, -9.696439889920343447, 56.85231026484398598 ) ) ;
#1792=CARTESIAN_POINT ( 'NONE',  ( -18.10194853779420043, -23.13696500758647190, 54.00231026484399166 ) ) ;
#1793=VERTEX_POINT ( 'NONE', #6232 ) ;
#1794=LINE ( 'NONE', #13351, #11380 ) ;
#1795=ORIENTED_EDGE ( 'NONE', *, *, #4686, .F. ) ;
#1796=ORIENTED_EDGE ( 'NONE', *, *, #5413, .F. ) ;
#1800=ORIENTED_EDGE ( 'NONE', *, *, #12612, .T. ) ;
#1802=VECTOR ( 'NONE', #6555, 1000.000000000000114 ) ;
#1803=EDGE_CURVE ( 'NONE', #1165, #7506, #4327, .T. ) ;
#1805=LINE ( 'NONE', #6304, #10117 ) ;
#1806=PLANE ( 'NONE',  #1704 ) ;
#1807=CARTESIAN_POINT ( 'NONE',  ( -12.11547932532413263, -20.83938426843124603, 57.00231026484399166 ) ) ;
#1808=EDGE_CURVE ( 'NONE', #10889, #6707, #6009, .T. ) ;
#1809=VECTOR ( 'NONE', #14780, 1000.000000000000000 ) ;
#1810=CARTESIAN_POINT ( 'NONE',  ( -6.488891646287396675, -12.42729319905174634, 56.85231026484400019 ) ) ;
#1811=DIRECTION ( 'NONE',  ( 0.5975035461963189576, 0.8018662683283437342, 0.000000000000000000 ) ) ;
#1820=DIRECTION ( 'NONE',  ( 0.5975035461963189576, 0.8018662683283437342, 0.000000000000000000 ) ) ;
#1823=LINE ( 'NONE', #6469, #1887 ) ;
#1824=EDGE_CURVE ( 'NONE', #2908, #4255, #3953, .T. ) ;
#1825=PLANE ( 'NONE',  #5279 ) ;
#1826=LINE ( 'NONE', #8927, #4996 ) ;
#1829=DIRECTION ( 'NONE',  ( 8.018662683283438208E-16, -5.975035461963189015E-16, -1.000000000000000000 ) ) ;
#1830=ORIENTED_EDGE ( 'NONE', *, *, #7449, .F. ) ;
#1832=ORIENTED_EDGE ( 'NONE', *, *, #8780, .F. ) ;
#1833=EDGE_LOOP ( 'NONE', ( #1115, #6516, #7526, #11408 ) ) ;
#1834=DIRECTION ( 'NONE',  ( -0.5779813897169993053, 0.8160499452489450301, -9.510565162951571123E-16 ) ) ;
#1835=CARTESIAN_POINT ( 'NONE',  ( -11.55238169831532957, -21.67927775123549594, 57.00231026484399166 ) ) ;
#1837=DIRECTION ( 'NONE',  ( 8.018662683283438208E-16, -5.975035461963189015E-16, -1.000000000000000000 ) ) ;
#1841=CARTESIAN_POINT ( 'NONE',  ( -16.99345872630171428, -15.51204466325908982, 51.25231026484399166 ) ) ;
#1842=EDGE_CURVE ( 'NONE', #7908, #8391, #3593, .T. ) ;
#1844=DIRECTION ( 'NONE',  ( -0.6061090314442014737, 0.7953815700667020705, -9.612616959383187437E-16 ) ) ;
#1846=ADVANCED_FACE ( 'NONE', ( #9616 ), #1510, .F. ) ;
#1847=EDGE_LOOP ( 'NONE', ( #5397, #11160, #13721, #7720 ) ) ;
#1849=ORIENTED_EDGE ( 'NONE', *, *, #1085, .T. ) ;
#1850=PLANE ( 'NONE',  #6796 ) ;
#1852=ORIENTED_EDGE ( 'NONE', *, *, #1484, .T. ) ;
#1853=CARTESIAN_POINT ( 'NONE',  ( -9.328067836852527606, -18.71527762440592468, 56.85231026484400019 ) ) ;
#1855=VERTEX_POINT ( 'NONE', #13073 ) ;
#1856=VECTOR ( 'NONE', #7773, 1000.000000000000000 ) ;
#1859=CARTESIAN_POINT ( 'NONE',  ( -6.540243082598547808, -14.95284924095401458, 56.85231026484400019 ) ) ;
#1861=ADVANCED_FACE ( 'NONE', ( #1437 ), #4958, .F. ) ;
#1864=DIRECTION ( 'NONE',  ( 8.018662683283438208E-16, -5.975035461963189015E-16, -1.000000000000000000 ) ) ;
#1865=EDGE_CURVE ( 'NONE', #13612, #8489, #12217, .T. ) ;
#1866=VERTEX_POINT ( 'NONE', #10213 ) ;
#1873=ADVANCED_FACE ( 'NONE', ( #13516 ), #7826, .T. ) ;
#1875=VECTOR ( 'NONE', #6712, 1000.000000000000000 ) ;
#1877=DIRECTION ( 'NONE',  ( 0.1272150336605032961, -0.9918751611018177261, 6.946583704589934213E-16 ) ) ;
#1878=CARTESIAN_POINT ( 'NONE',  ( -12.84854673063650132, -12.36513540471286454, 56.75231026484397745 ) ) ;
#1879=CIRCLE ( 'NONE', #14342, 9.974999999999999645 ) ;
#1880=EDGE_CURVE ( 'NONE', #2588, #6205, #14660, .T. ) ;
#1882=EDGE_CURVE ( 'NONE', #1083, #13264, #3103, .T. ) ;
#1887=VECTOR ( 'NONE', #3818, 1000.000000000000114 ) ;
#1889=ORIENTED_EDGE ( 'NONE', *, *, #6659, .F. ) ;
#1893=EDGE_LOOP ( 'NONE', ( #5402, #520, #6069, #2568 ) ) ;
#1894=CARTESIAN_POINT ( 'NONE',  ( -9.031792552787402784, -10.63903015472409486, 56.85231026484400019 ) ) ;
#1895=CARTESIAN_POINT ( 'NONE',  ( -15.49969986081092088, -13.50737899243822504, 57.00231026484397745 ) ) ;
#1898=PLANE ( 'NONE',  #1392 ) ;
#1899=VECTOR ( 'NONE', #11749, 1000.000000000000000 ) ;
#1901=CARTESIAN_POINT ( 'NONE',  ( -24.39712111458419130, -18.01698208283363556, 56.85231026484398598 ) ) ;
#1905=ORIENTED_EDGE ( 'NONE', *, *, #8887, .T. ) ;
#1906=VECTOR ( 'NONE', #3559, 1000.000000000000000 ) ;
#1907=CARTESIAN_POINT ( 'NONE',  ( -8.525484111995742964, -7.700351810740323266, 57.00231026484399166 ) ) ;
#1909=VERTEX_POINT ( 'NONE', #9984 ) ;
#1910=FACE_OUTER_BOUND ( 'NONE', #5741, .T. ) ;
#1912=VECTOR ( 'NONE', #6196, 1000.000000000000114 ) ;
#1913=FACE_OUTER_BOUND ( 'NONE', #2325, .T. ) ;
#1915=ADVANCED_FACE ( 'NONE', ( #5545 ), #9914, .T. ) ;
#1916=ADVANCED_FACE ( 'NONE', ( #5473 ), #14736, .F. ) ;
#1917=CARTESIAN_POINT ( 'NONE',  ( -20.39403028972282428, -7.084672814149619136, 56.85231026484398598 ) ) ;
#1920=CARTESIAN_POINT ( 'NONE',  ( -15.83606446161808456, -16.37446674635458876, 51.10586365543726117 ) ) ;
#1926=ORIENTED_EDGE ( 'NONE', *, *, #10584, .T. ) ;
#1927=DIRECTION ( 'NONE',  ( 0.7276687409742212953, 0.6859287159822015090, 1.736481776669299976E-16 ) ) ;
#1930=ORIENTED_EDGE ( 'NONE', *, *, #10174, .F. ) ;
#1931=CARTESIAN_POINT ( 'NONE',  ( -9.959408463899000807, -21.80230492564002276, 54.00231026484400587 ) ) ;
#1933=DIRECTION ( 'NONE',  ( -8.018662683283438208E-16, 5.975035461963189015E-16, 1.000000000000000000 ) ) ;
#1935=VECTOR ( 'NONE', #96, 1000.000000000000000 ) ;
#1938=VECTOR ( 'NONE', #7417, 1000.000000000000114 ) ;
#1939=ORIENTED_EDGE ( 'NONE', *, *, #13456, .F. ) ;
#1943=ORIENTED_EDGE ( 'NONE', *, *, #4054, .T. ) ;
#1946=CARTESIAN_POINT ( 'NONE',  ( -8.971570239337626873, -21.04953708182106098, 57.00231026484399166 ) ) ;
#1948=VECTOR ( 'NONE', #11790, 1000.000000000000000 ) ;
#1950=CARTESIAN_POINT ( 'NONE',  ( -12.76843194806299842, -13.82780931059433271, 56.75231026484399166 ) ) ;
#1952=EDGE_CURVE ( 'NONE', #8358, #6010, #11068, .T. ) ;
#1954=CARTESIAN_POINT ( 'NONE',  ( -5.526612771747946518, -13.70272205979775748, 56.85231026484400019 ) ) ;
#1957=PLANE ( 'NONE',  #6193 ) ;
#1960=VERTEX_POINT ( 'NONE', #10132 ) ;
#1961=FACE_OUTER_BOUND ( 'NONE', #14494, .T. ) ;
#1962=DIRECTION ( 'NONE',  ( 0.9040177279761104634, 0.4274949678123838859, 4.694715627858909121E-16 ) ) ;
#1964=ORIENTED_EDGE ( 'NONE', *, *, #10838, .T. ) ;
#1965=FACE_OUTER_BOUND ( 'NONE', #9078, .T. ) ;
#1967=CARTESIAN_POINT ( 'NONE',  ( -18.43409448121630945, -5.984417261063049942, 56.85231026484398598 ) ) ;
#1968=LINE ( 'NONE', #10061, #12820 ) ;
#1972=ADVANCED_FACE ( 'NONE', ( #11220 ), #737, .F. ) ;
#1974=CARTESIAN_POINT ( 'NONE',  ( -15.45180655762527699, -13.52173975529984418, 56.85231026484398598 ) ) ;
#1980=CARTESIAN_POINT ( 'NONE',  ( -18.15085299098534577, -14.64962258016358199, 56.75231026484397745 ) ) ;
#1983=ORIENTED_EDGE ( 'NONE', *, *, #3367, .F. ) ;
#1985=LINE ( 'NONE', #7783, #11547 ) ;
#1987=EDGE_CURVE ( 'NONE', #5856, #642, #8685, .T. ) ;
#1988=DIRECTION ( 'NONE',  ( -0.9957106782009873536, -0.09252159378507134047, -7.431448254773946593E-16 ) ) ;
#1993=DIRECTION ( 'NONE',  ( -8.018662683283438208E-16, 5.975035461963189015E-16, 1.000000000000000000 ) ) ;
#1994=EDGE_CURVE ( 'NONE', #7908, #1793, #3332, .T. ) ;
#1995=LINE ( 'NONE', #9171, #10574 ) ;
#1998=LINE ( 'NONE', #10691, #3351 ) ;
#1999=CARTESIAN_POINT ( 'NONE',  ( -9.251715890255169938, -8.391880844292892050, 56.85231026484398598 ) ) ;
#2000=EDGE_LOOP ( 'NONE', ( #9896, #8367, #1939, #14550, #9331, #7410, #910, #10343, #14966, #2582, #3013, #9491, #9674, #4922, #5681, #7893, #3016, #725, #11089, #13395, #7140, #11239, #8234, #12200, #11532, #11838, #2033, #6383, #4052, #1090, #2136, #4221, #1403, #5996, #11920, #11963, #892, #9564, #11403, #13099, #8619, #4823, #10537, #9188, #11351, #5824, #8576, #14215, #8041, #13149, #4145, #2623, #10185, #2845, #13325, #2439, #5132, #8048, #4508, #735, #13449, #6191, #10853, #5120, #14332, #8200, #9101, #7690, #12126, #10347, #15073, #9430, #11895, #2736, #4037, #6352, #1983, #3068, #10997, #6871, #5073, #8581, #14641, #2342, #2309, #5128, #2095, #9777, #8804, #15069, #7631, #2847, #2718, #5362, #13193, #9829, #13079, #5922, #5765, #773, #659, #11259, #12675, #262, #6089, #14810, #11593, #4195, #4465, #12949, #3043, #2684, #9023, #9785, #533, #10287, #13024, #6773, #10364, #4152, #4871, #6630, #10079, #6422, #3558, #10272, #8950, #9508, #1188, #905, #1852, #8740, #4243, #2080, #5034, #875, #3821, #1796, #8258, #10403, #6297, #9755, #7143, #2703, #12716, #10408, #8785, #7334, #257, #6107, #6449, #11724, #2905, #14417, #4111, #9008, #14386, #5234, #12014, #10038, #85, #10520, #5979, #11834, #14681, #11645, #4031, #1573, #11487, #11188, #6424, #5512, #6611, #1167, #5713, #7487, #1499, #5859, #3710, #1461, #9409, #1795 ) ) ;
#2002=DIRECTION ( 'NONE',  ( 0.5975035461963189576, 0.8018662683283437342, 0.000000000000000000 ) ) ;
#2003=ORIENTED_EDGE ( 'NONE', *, *, #4497, .T. ) ;
#2004=CIRCLE ( 'NONE', #3705, 9.974999999999999645 ) ;
#2007=CARTESIAN_POINT ( 'NONE',  ( -5.923714809816988058, -16.30043024566306187, 54.00231026484400587 ) ) ;
#2008=AXIS2_PLACEMENT_3D ( 'NONE', #7616, #10918, #12298 ) ;
#2010=DIRECTION ( 'NONE',  ( -8.018662683283439195E-16, 5.975035461963190001E-16, 1.000000000000000000 ) ) ;
#2014=DIRECTION ( 'NONE',  ( 0.04695496274984587576, 0.9988970074402868660, -5.591929034707467802E-16 ) ) ;
#2015=ORIENTED_EDGE ( 'NONE', *, *, #9387, .T. ) ;
#2020=VERTEX_POINT ( 'NONE', #2341 ) ;
#2024=AXIS2_PLACEMENT_3D ( 'NONE', #4230, #2704, #8583 ) ;
#2033=ORIENTED_EDGE ( 'NONE', *, *, #14429, .T. ) ;
#2036=ORIENTED_EDGE ( 'NONE', *, *, #2242, .T. ) ;
#2038=FACE_OUTER_BOUND ( 'NONE', #6532, .T. ) ;
#2039=AXIS2_PLACEMENT_3D ( 'NONE', #12387, #9930, #11161 ) ;
#2044=ORIENTED_EDGE ( 'NONE', *, *, #4686, .T. ) ;
#2046=CARTESIAN_POINT ( 'NONE',  ( -22.33089034576175180, -8.323646113680169378, 57.00231026484397745 ) ) ;
#2048=AXIS2_PLACEMENT_3D ( 'NONE', #3286, #7934, #10469 ) ;
#2050=CARTESIAN_POINT ( 'NONE',  ( -8.639554752241616953, -9.247137322136806503, 56.85231026484400019 ) ) ;
#2051=EDGE_CURVE ( 'NONE', #4847, #13967, #11515, .T. ) ;
#2061=CARTESIAN_POINT ( 'NONE',  ( -15.16333526000375365, -10.64029123852185776, 56.89875687425070794 ) ) ;
#2065=DIRECTION ( 'NONE',  ( 8.018662683283438208E-16, -5.975035461963189015E-16, -1.000000000000000000 ) ) ;
#2068=PLANE ( 'NONE',  #2985 ) ;
#2069=LINE ( 'NONE', #5502, #850 ) ;
#2075=FACE_OUTER_BOUND ( 'NONE', #2759, .T. ) ;
#2076=ORIENTED_EDGE ( 'NONE', *, *, #5249, .T. ) ;
#2077=DIRECTION ( 'NONE',  ( -8.018662683283438208E-16, 5.975035461963189015E-16, 1.000000000000000000 ) ) ;
#2078=CARTESIAN_POINT ( 'NONE',  ( -18.43409448121630945, -5.984417261063049942, 57.00231026484397745 ) ) ;
#2079=FACE_OUTER_BOUND ( 'NONE', #3086, .T. ) ;
#2080=ORIENTED_EDGE ( 'NONE', *, *, #2193, .F. ) ;
#2081=ORIENTED_EDGE ( 'NONE', *, *, #5399, .F. ) ;
#2087=ADVANCED_FACE ( 'NONE', ( #8140 ), #12673, .T. ) ;
#2094=DIRECTION ( 'NONE',  ( 8.018662683283438208E-16, -5.975035461963189015E-16, -1.000000000000000000 ) ) ;
#2095=ORIENTED_EDGE ( 'NONE', *, *, #12824, .T. ) ;
#2096=FACE_OUTER_BOUND ( 'NONE', #1893, .T. ) ;
#2097=ORIENTED_EDGE ( 'NONE', *, *, #9986, .F. ) ;
#2098=ORIENTED_EDGE ( 'NONE', *, *, #2319, .F. ) ;
#2101=CARTESIAN_POINT ( 'NONE',  ( -7.264457220180047692, -15.89840986842769333, 56.85231026484400019 ) ) ;
#2102=ADVANCED_FACE ( 'NONE', ( #5696 ), #4556, .F. ) ;
#2103=EDGE_CURVE ( 'NONE', #11708, #8808, #7400, .T. ) ;
#2104=CIRCLE ( 'NONE', #4796, 9.974999999999999645 ) ;
#2105=DIRECTION ( 'NONE',  ( -0.9805849309054471830, -0.1960948578651655061, -6.691306063588582470E-16 ) ) ;
#2106=CARTESIAN_POINT ( 'NONE',  ( -15.49969986081092088, -13.50737899243822504, 56.85231026484398598 ) ) ;
#2109=DIRECTION ( 'NONE',  ( 0.5975035461963188466, 0.8018662683283437342, 0.000000000000000000 ) ) ;
#2111=ORIENTED_EDGE ( 'NONE', *, *, #8347, .F. ) ;
#2114=VERTEX_POINT ( 'NONE', #12124 ) ;
#2115=ORIENTED_EDGE ( 'NONE', *, *, #8226, .T. ) ;
#2118=ORIENTED_EDGE ( 'NONE', *, *, #3346, .F. ) ;
#2122=DIRECTION ( 'NONE',  ( -0.8885476655824650072, -0.4587843131450243805, -4.383711467890778149E-16 ) ) ;
#2124=DIRECTION ( 'NONE',  ( -8.018662683283438208E-16, 5.975035461963189015E-16, 1.000000000000000000 ) ) ;
#2125=DIRECTION ( 'NONE',  ( -0.01206535623791937448, -0.9999272109403024578, 5.877852522924727828E-16 ) ) ;
#2134=VERTEX_POINT ( 'NONE', #1420 ) ;
#2136=ORIENTED_EDGE ( 'NONE', *, *, #11513, .F. ) ;
#2138=CARTESIAN_POINT ( 'NONE',  ( -23.54151295824578227, -12.77219731018227300, 56.85231026484398598 ) ) ;
#2142=CARTESIAN_POINT ( 'NONE',  ( -14.00164528647249007, -5.572553380472728968, 57.00231026484397745 ) ) ;
#2143=CARTESIAN_POINT ( 'NONE',  ( -15.49969986081091200, -13.50737899243823215, 48.00231026484398456 ) ) ;
#2144=EDGE_CURVE ( 'NONE', #5192, #10261, #6221, .T. ) ;
#2146=CARTESIAN_POINT ( 'NONE',  ( -15.49969986081092088, -13.50737899243822504, 57.00231026484397745 ) ) ;
#2148=CARTESIAN_POINT ( 'NONE',  ( -5.596483669297570351, -12.31283553816471432, 56.85231026484400019 ) ) ;
#2149=EDGE_CURVE ( 'NONE', #5040, #15014, #8290, .T. ) ;
#2150=CARTESIAN_POINT ( 'NONE',  ( -19.06972223273333711, -21.85101071153832919, 56.85231026484400019 ) ) ;
#2151=VECTOR ( 'NONE', #2496, 1000.000000000000000 ) ;
#2154=ORIENTED_EDGE ( 'NONE', *, *, #13626, .F. ) ;
#2157=ORIENTED_EDGE ( 'NONE', *, *, #13527, .F. ) ;
#2159=CARTESIAN_POINT ( 'NONE',  ( -21.79090396836353705, -19.33464257641254136, 57.00231026484397745 ) ) ;
#2160=CARTESIAN_POINT ( 'NONE',  ( -15.83606446161809522, -16.37446674635458166, 56.75231026484397745 ) ) ;
#2165=AXIS2_PLACEMENT_3D ( 'NONE', #11467, #12933, #8243 ) ;
#2168=DIRECTION ( 'NONE',  ( -8.018662683283438208E-16, 5.975035461963189015E-16, 1.000000000000000000 ) ) ;
#2169=ORIENTED_EDGE ( 'NONE', *, *, #12328, .F. ) ;
#2171=ORIENTED_EDGE ( 'NONE', *, *, #12744, .F. ) ;
#2173=CARTESIAN_POINT ( 'NONE',  ( -20.59651154950486784, -18.41489981358536809, 56.85231026484398598 ) ) ;
#2176=ORIENTED_EDGE ( 'NONE', *, *, #14828, .T. ) ;
#2177=CARTESIAN_POINT ( 'NONE',  ( -15.49969986081091200, -13.50737899243823037, 48.00231026484398456 ) ) ;
#2180=PLANE ( 'NONE',  #18 ) ;
#2183=LINE ( 'NONE', #4552, #10835 ) ;
#2186=CARTESIAN_POINT ( 'NONE',  ( -21.79090396836353705, -19.33464257641254136, 56.85231026484398598 ) ) ;
#2193=EDGE_CURVE ( 'NONE', #13665, #3051, #11894, .T. ) ;
#2194=DIRECTION ( 'NONE',  ( -0.4491835085186243748, -0.8934395198752397294, 1.736481776669299976E-16 ) ) ;
#2195=FACE_OUTER_BOUND ( 'NONE', #9256, .T. ) ;
#2196=VERTEX_POINT ( 'NONE', #14192 ) ;
#2197=DIRECTION ( 'NONE',  ( 8.018662683283438208E-16, -5.975035461963189015E-16, -1.000000000000000000 ) ) ;
#2199=VECTOR ( 'NONE', #9977, 1000.000000000000000 ) ;
#2200=CARTESIAN_POINT ( 'NONE',  ( -20.54757852167729837, -19.81012014412530320, 57.00231026484397745 ) ) ;
#2201=LINE ( 'NONE', #8156, #6447 ) ;
#2203=ORIENTED_EDGE ( 'NONE', *, *, #4234, .F. ) ;
#2207=ADVANCED_FACE ( 'NONE', ( #9753 ), #13057, .F. ) ;
#2208=CARTESIAN_POINT ( 'NONE',  ( -10.95221305062249684, -4.629260458021021485, 56.85231026484398598 ) ) ;
#2209=EDGE_LOOP ( 'NONE', ( #1296, #13653, #4393, #3487 ) ) ;
#2213=DIRECTION ( 'NONE',  ( -8.018662683283438208E-16, 5.975035461963189015E-16, 1.000000000000000000 ) ) ;
#2215=CARTESIAN_POINT ( 'NONE',  ( -16.34789837066771767, -3.568506607309358092, 54.00231026484397745 ) ) ;
#2216=VECTOR ( 'NONE', #12876, 999.9999999999998863 ) ;
#2219=CARTESIAN_POINT ( 'NONE',  ( -13.57551609484869282, -3.719726473329895811, 57.00231026484397745 ) ) ;
#2220=CARTESIAN_POINT ( 'NONE',  ( -10.84210729886283531, -6.910555398701176522, 56.85231026484398598 ) ) ;
#2221=CARTESIAN_POINT ( 'NONE',  ( -16.41401162527548507, -4.478243707298169340, 57.00231026484397745 ) ) ;
#2222=LINE ( 'NONE', #4371, #4233 ) ;
#2223=EDGE_CURVE ( 'NONE', #7254, #11993, #1640, .T. ) ;
#2225=FACE_OUTER_BOUND ( 'NONE', #8148, .T. ) ;
#2226=ORIENTED_EDGE ( 'NONE', *, *, #13237, .T. ) ;
#2229=EDGE_LOOP ( 'NONE', ( #10517, #10508, #4637, #14470 ) ) ;
#2231=FACE_OUTER_BOUND ( 'NONE', #9448, .T. ) ;
#2234=CARTESIAN_POINT ( 'NONE',  ( -19.51793069539949599, -6.502732608789604463, 57.00231026484397745 ) ) ;
#2235=VECTOR ( 'NONE', #8892, 1000.000000000000000 ) ;
#2236=DIRECTION ( 'NONE',  ( -8.018662683283438208E-16, 5.975035461963189015E-16, 1.000000000000000000 ) ) ;
#2237=EDGE_LOOP ( 'NONE', ( #14384, #10976, #3945, #8743 ) ) ;
#2239=ADVANCED_FACE ( 'NONE', ( #10826 ), #6140, .F. ) ;
#2242=EDGE_CURVE ( 'NONE', #10422, #14849, #6514, .T. ) ;
#2247=VECTOR ( 'NONE', #10805, 1000.000000000000114 ) ;
#2248=EDGE_CURVE ( 'NONE', #17, #10747, #2104, .T. ) ;
#2249=CARTESIAN_POINT ( 'NONE',  ( -9.452813543643186378, -20.27468391147722926, 57.00231026484399166 ) ) ;
#2250=ORIENTED_EDGE ( 'NONE', *, *, #10858, .T. ) ;
#2256=VECTOR ( 'NONE', #14650, 1000.000000000000000 ) ;
#2257=VECTOR ( 'NONE', #6759, 1000.000000000000114 ) ;
#2258=VECTOR ( 'NONE', #11093, 1000.000000000000114 ) ;
#2260=CARTESIAN_POINT ( 'NONE',  ( -10.96544185377836911, -6.825182173602284408, 57.00231026484397745 ) ) ;
#2261=CARTESIAN_POINT ( 'NONE',  ( -23.36093307149983289, -11.66014798166512634, 56.85231026484398598 ) ) ;
#2262=ORIENTED_EDGE ( 'NONE', *, *, #7855, .T. ) ;
#2264=EDGE_CURVE ( 'NONE', #12036, #10807, #1794, .T. ) ;
#2267=ORIENTED_EDGE ( 'NONE', *, *, #7549, .T. ) ;
#2268=EDGE_LOOP ( 'NONE', ( #11162, #2666, #11805, #3888 ) ) ;
#2270=ADVANCED_FACE ( 'NONE', ( #10037 ), #5237, .T. ) ;
#2274=ORIENTED_EDGE ( 'NONE', *, *, #4328, .F. ) ;
#2279=PLANE ( 'NONE',  #10446 ) ;
#2280=VECTOR ( 'NONE', #7101, 1000.000000000000227 ) ;
#2281=DIRECTION ( 'NONE',  ( -0.8599296884906622029, 0.5104125104779001498, -9.945218953682734920E-16 ) ) ;
#2287=CARTESIAN_POINT ( 'NONE',  ( -8.194314379747492438, -16.94868586237404529, 56.85231026484400019 ) ) ;
#2290=VERTEX_POINT ( 'NONE', #12426 ) ;
#2291=PLANE ( 'NONE',  #9591 ) ;
#2293=AXIS2_PLACEMENT_3D ( 'NONE', #8624, #10996, #2884 ) ;
#2294=FACE_OUTER_BOUND ( 'NONE', #2000, .T. ) ;
#2295=PRESENTATION_STYLE_ASSIGNMENT (( #10545 ) ) ;
#2296=ADVANCED_FACE ( 'NONE', ( #2862 ), #4239, .T. ) ;
#2297=CARTESIAN_POINT ( 'NONE',  ( -15.45180655762527699, -13.52173975529984418, 56.85231026484398598 ) ) ;
#2303=ORIENTED_EDGE ( 'NONE', *, *, #11629, .F. ) ;
#2305=ORIENTED_EDGE ( 'NONE', *, *, #9974, .F. ) ;
#2308=ORIENTED_EDGE ( 'NONE', *, *, #10566, .T. ) ;
#2309=ORIENTED_EDGE ( 'NONE', *, *, #7, .F. ) ;
#2310=PLANE ( 'NONE',  #2632 ) ;
#2311=ORIENTED_EDGE ( 'NONE', *, *, #5771, .T. ) ;
#2313=PLANE ( 'NONE',  #4874 ) ;
#2314=CARTESIAN_POINT ( 'NONE',  ( -15.45180655762527699, -13.52173975529984418, 56.85231026484398598 ) ) ;
#2315=VECTOR ( 'NONE', #7697, 1000.000000000000000 ) ;
#2317=CARTESIAN_POINT ( 'NONE',  ( -6.405625242116718354, -17.60596799715946759, 56.85231026484400019 ) ) ;
#2319=EDGE_CURVE ( 'NONE', #8706, #14042, #10975, .T. ) ;
#2321=ORIENTED_EDGE ( 'NONE', *, *, #8050, .F. ) ;
#2325=EDGE_LOOP ( 'NONE', ( #7781, #5567, #10277, #9935 ) ) ;
#2326=EDGE_LOOP ( 'NONE', ( #5933, #8488, #7665, #9351 ) ) ;
#2327=VECTOR ( 'NONE', #13331, 1000.000000000000000 ) ;
#2331=EDGE_CURVE ( 'NONE', #12982, #3306, #7521, .T. ) ;
#2338=DIRECTION ( 'NONE',  ( -0.4895147004624045839, 0.8719950447285823580, -9.135454576426008610E-16 ) ) ;
#2340=DIRECTION ( 'NONE',  ( 0.5975035461963189576, 0.8018662683283437342, 0.000000000000000000 ) ) ;
#2341=CARTESIAN_POINT ( 'NONE',  ( -20.31707134655588121, -4.772760685475329723, 56.85231026484398598 ) ) ;
#2342=ORIENTED_EDGE ( 'NONE', *, *, #6057, .F. ) ;
#2346=LINE ( 'NONE', #1425, #9833 ) ;
#2349=ORIENTED_EDGE ( 'NONE', *, *, #13751, .T. ) ;
#2351=EDGE_CURVE ( 'NONE', #10077, #9919, #10425, .T. ) ;
#2356=DIRECTION ( 'NONE',  ( 0.5975035461963189576, 0.8018662683283437342, 0.000000000000000000 ) ) ;
#2360=AXIS2_PLACEMENT_3D ( 'NONE', #2146, #10628, #1139 ) ;
#2363=CARTESIAN_POINT ( 'NONE',  ( -8.131654986474892155, -16.81240013151894530, 56.85231026484400019 ) ) ;
#2364=ORIENTED_EDGE ( 'NONE', *, *, #7247, .T. ) ;
#2365=VERTEX_POINT ( 'NONE', #8817 ) ;
#2366=DIRECTION ( 'NONE',  ( -8.018662683283439195E-16, 5.975035461963190001E-16, 1.000000000000000000 ) ) ;
#2369=DIRECTION ( 'NONE',  ( -8.018662683283438208E-16, 5.975035461963189015E-16, 1.000000000000000000 ) ) ;
#2370=AXIS2_PLACEMENT_3D ( 'NONE', #7771, #10300, #14900 ) ;
#2373=LINE ( 'NONE', #7171, #11402 ) ;
#2374=VECTOR ( 'NONE', #4375, 1000.000000000000114 ) ;
#2375=CARTESIAN_POINT ( 'NONE',  ( -23.09568838840838012, -16.24821979201191979, 57.00231026484397745 ) ) ;
#2378=FACE_OUTER_BOUND ( 'NONE', #6931, .T. ) ;
#2379=ORIENTED_EDGE ( 'NONE', *, *, #3812, .F. ) ;
#2380=LINE ( 'NONE', #10635, #12264 ) ;
#2381=ORIENTED_EDGE ( 'NONE', *, *, #9731, .T. ) ;
#2382=PLANE ( 'NONE',  #14009 ) ;
#2384=EDGE_CURVE ( 'NONE', #1325, #6707, #6748, .T. ) ;
#2387=DIRECTION ( 'NONE',  ( 0.9437508163134059602, 0.3306575217771102193, 5.591929034707491467E-16 ) ) ;
#2388=VERTEX_POINT ( 'NONE', #5604 ) ;
#2390=DIRECTION ( 'NONE',  ( -8.018662683283438208E-16, 5.975035461963189015E-16, 1.000000000000000000 ) ) ;
#2391=LINE ( 'NONE', #5970, #7440 ) ;
#2393=VECTOR ( 'NONE', #12672, 1000.000000000000000 ) ;
#2394=CARTESIAN_POINT ( 'NONE',  ( -15.83606446161809167, -16.37446674635458521, 51.25231026484399166 ) ) ;
#2398=VERTEX_POINT ( 'NONE', #2173 ) ;
#2400=ORIENTED_EDGE ( 'NONE', *, *, #11514, .T. ) ;
#2401=ORIENTED_EDGE ( 'NONE', *, *, #2223, .F. ) ;
#2402=ORIENTED_EDGE ( 'NONE', *, *, #6901, .T. ) ;
#2404=DIRECTION ( 'NONE',  ( -8.018662683283438208E-16, 5.975035461963189015E-16, 1.000000000000000000 ) ) ;
#2405=VERTEX_POINT ( 'NONE', #4696 ) ;
#2407=VECTOR ( 'NONE', #5945, 1000.000000000000114 ) ;
#2408=VECTOR ( 'NONE', #8499, 999.9999999999998863 ) ;
#2409=CARTESIAN_POINT ( 'NONE',  ( -13.92794721577312878, -5.586467200048621073, 57.00231026484397745 ) ) ;
#2411=LINE ( 'NONE', #10896, #14768 ) ;
#2412=LINE ( 'NONE', #12827, #14989 ) ;
#2414=EDGE_LOOP ( 'NONE', ( #2044, #6800, #2303, #14872 ) ) ;
#2415=DIRECTION ( 'NONE',  ( 8.018662683283438208E-16, -5.975035461963189015E-16, -1.000000000000000000 ) ) ;
#2417=ORIENTED_EDGE ( 'NONE', *, *, #9174, .F. ) ;
#2420=ADVANCED_FACE ( 'NONE', ( #9274 ), #11423, .F. ) ;
#2423=CARTESIAN_POINT ( 'NONE',  ( -13.18491133144367389, -15.23222315862922827, 51.25231026484399166 ) ) ;
#2426=ADVANCED_FACE ( 'NONE', ( #8199 ), #3463, .T. ) ;
#2429=DIRECTION ( 'NONE',  ( 8.018662683283438208E-16, -5.975035461963189015E-16, -1.000000000000000000 ) ) ;
#2432=ORIENTED_EDGE ( 'NONE', *, *, #5391, .T. ) ;
#2435=ORIENTED_EDGE ( 'NONE', *, *, #10473, .F. ) ;
#2436=ADVANCED_FACE ( 'NONE', ( #6819 ), #13799, .T. ) ;
#2437=CARTESIAN_POINT ( 'NONE',  ( -19.62128088291994388, -20.45131122700032833, 56.85231026484398598 ) ) ;
#2438=EDGE_CURVE ( 'NONE', #5451, #7506, #13720, .T. ) ;
#2439=ORIENTED_EDGE ( 'NONE', *, *, #6440, .F. ) ;
#2442=DIRECTION ( 'NONE',  ( -0.8543800322332384400, -0.5196486895212286683, -3.746065934159129782E-16 ) ) ;
#2443=CARTESIAN_POINT ( 'NONE',  ( -23.02734322232803521, -10.58405290357860373, 56.85231026484398598 ) ) ;
#2445=VECTOR ( 'NONE', #14669, 1000.000000000000114 ) ;
#2447=CARTESIAN_POINT ( 'NONE',  ( -22.13265177292497299, -18.11337496850924822, 56.85231026484398598 ) ) ;
#2449=CARTESIAN_POINT ( 'NONE',  ( -15.16333526000374832, -10.64029123852186487, 51.00231026484399166 ) ) ;
#2451=ORIENTED_EDGE ( 'NONE', *, *, #11284, .F. ) ;
#2452=CARTESIAN_POINT ( 'NONE',  ( -9.452813543643186378, -20.27468391147722926, 56.85231026484400019 ) ) ;
#2454=EDGE_CURVE ( 'NONE', #4255, #4418, #11350, .T. ) ;
#2458=ORIENTED_EDGE ( 'NONE', *, *, #669, .T. ) ;
#2460=CIRCLE ( 'NONE', #8053, 9.974999999999999645 ) ;
#2461=DIRECTION ( 'NONE',  ( 8.018662683283438208E-16, -5.975035461963189015E-16, -1.000000000000000000 ) ) ;
#2463=CARTESIAN_POINT ( 'NONE',  ( -7.424382730750140880, -13.52981220323889566, 56.85231026484400019 ) ) ;
#2464=DIRECTION ( 'NONE',  ( -0.8543800322332379960, -0.5196486895212294455, -3.746065934159121401E-16 ) ) ;
#2465=LINE ( 'NONE', #7109, #8800 ) ;
#2467=ADVANCED_FACE ( 'NONE', ( #2096 ), #950, .F. ) ;
#2468=DIRECTION ( 'NONE',  ( 0.9183863840214728791, 0.3956847857120156520, 4.999999999999998416E-16 ) ) ;
#2473=ORIENTED_EDGE ( 'NONE', *, *, #13170, .T. ) ;
#2475=ORIENTED_EDGE ( 'NONE', *, *, #6921, .T. ) ;
#2479=EDGE_CURVE ( 'NONE', #8450, #2196, #1020, .T. ) ;
#2485=CARTESIAN_POINT ( 'NONE',  ( -16.24681173062539230, -5.467015265965240012, 56.85231026484398598 ) ) ;
#2487=ORIENTED_EDGE ( 'NONE', *, *, #8691, .F. ) ;
#2489=ORIENTED_EDGE ( 'NONE', *, *, #1571, .T. ) ;
#2493=VECTOR ( 'NONE', #13084, 1000.000000000000114 ) ;
#2494=DIRECTION ( 'NONE',  ( -8.018662683283438208E-16, 5.975035461963189015E-16, 1.000000000000000000 ) ) ;
#2496=DIRECTION ( 'NONE',  ( -8.018662683283438208E-16, 5.975035461963189015E-16, 1.000000000000000000 ) ) ;
#2499=ADVANCED_FACE ( 'NONE', ( #9191 ), #10504, .F. ) ;
#2501=ORIENTED_EDGE ( 'NONE', *, *, #5983, .T. ) ;
#2503=VECTOR ( 'NONE', #4583, 1000.000000000000114 ) ;
#2504=DIRECTION ( 'NONE',  ( 8.018662683283438208E-16, -5.975035461963189015E-16, -1.000000000000000000 ) ) ;
#2506=VECTOR ( 'NONE', #7833, 1000.000000000000000 ) ;
#2507=AXIS2_PLACEMENT_3D ( 'NONE', #14562, #5302, #1864 ) ;
#2508=DIRECTION ( 'NONE',  ( 8.018662683283438208E-16, -5.975035461963189015E-16, -1.000000000000000000 ) ) ;
#2510=CARTESIAN_POINT ( 'NONE',  ( -15.49969986081092088, -13.50737899243822504, 57.00231026484397745 ) ) ;
#2513=FACE_OUTER_BOUND ( 'NONE', #5196, .T. ) ;
#2517=EDGE_CURVE ( 'NONE', #5816, #1460, #11877, .T. ) ;
#2518=DIRECTION ( 'NONE',  ( -8.018662683283438208E-16, 5.975035461963189015E-16, 1.000000000000000000 ) ) ;
#2525=LINE ( 'NONE', #8483, #11808 ) ;
#2526=ORIENTED_EDGE ( 'NONE', *, *, #12935, .F. ) ;
#2527=FACE_OUTER_BOUND ( 'NONE', #5546, .T. ) ;
#2529=LINE ( 'NONE', #8412, #5685 ) ;
#2530=ORIENTED_EDGE ( 'NONE', *, *, #6558, .T. ) ;
#2531=EDGE_CURVE ( 'NONE', #3877, #10428, #1879, .T. ) ;
#2532=VERTEX_POINT ( 'NONE', #8097 ) ;
#2534=DIRECTION ( 'NONE',  ( -8.018662683283438208E-16, 5.975035461963189015E-16, 1.000000000000000000 ) ) ;
#2536=VERTEX_POINT ( 'NONE', #11480 ) ;
#2538=DIRECTION ( 'NONE',  ( -0.2975196656469967227, 0.9547156899063193869, -8.090169943749448078E-16 ) ) ;
#2539=DIRECTION ( 'NONE',  ( -0.7582332219680880669, 0.6519834208811540188, -9.975640502598240034E-16 ) ) ;
#2541=EDGE_CURVE ( 'NONE', #5847, #7651, #1998, .T. ) ;
#2542=LINE ( 'NONE', #14091, #2645 ) ;
#2544=DIRECTION ( 'NONE',  ( 8.018662683283438208E-16, -5.975035461963189015E-16, -1.000000000000000000 ) ) ;
#2545=DIRECTION ( 'NONE',  ( 0.8772189822852964891, -0.4800904676395362780, 9.902680687415700047E-16 ) ) ;
#2549=VERTEX_POINT ( 'NONE', #1004 ) ;
#2550=ORIENTED_EDGE ( 'NONE', *, *, #8810, .T. ) ;
#2551=CARTESIAN_POINT ( 'NONE',  ( -24.53816276005083452, -12.69040994830970703, 56.85231026484398598 ) ) ;
#2552=ORIENTED_EDGE ( 'NONE', *, *, #5549, .F. ) ;
#2557=VECTOR ( 'NONE', #11379, 999.9999999999998863 ) ;
#2561=AXIS2_PLACEMENT_3D ( 'NONE', #11278, #11212, #5387 ) ;
#2563=LINE ( 'NONE', #1256, #3634 ) ;
#2567=ORIENTED_EDGE ( 'NONE', *, *, #13882, .T. ) ;
#2568=ORIENTED_EDGE ( 'NONE', *, *, #13277, .T. ) ;
#2573=EDGE_CURVE ( 'NONE', #1325, #8489, #10406, .T. ) ;
#2574=EDGE_CURVE ( 'NONE', #13689, #8949, #12796, .T. ) ;
#2576=CARTESIAN_POINT ( 'NONE',  ( -7.829332545557824652, -7.130382030772257629, 56.85231026484400019 ) ) ;
#2581=LINE ( 'NONE', #1578, #14503 ) ;
#2582=ORIENTED_EDGE ( 'NONE', *, *, #7637, .T. ) ;
#2583=DIRECTION ( 'NONE',  ( -8.018662683283438208E-16, 5.975035461963189015E-16, 1.000000000000000000 ) ) ;
#2584=CARTESIAN_POINT ( 'NONE',  ( -17.58300953724144122, -11.95501924286632267, 51.00231026484399166 ) ) ;
#2585=ORIENTED_EDGE ( 'NONE', *, *, #10869, .F. ) ;
#2586=CARTESIAN_POINT ( 'NONE',  ( -24.03943920472178775, -16.57887731378902885, 56.85231026484398598 ) ) ;
#2587=CARTESIAN_POINT ( 'NONE',  ( -25.45346213993001427, -14.15794911993140204, 54.00231026484397745 ) ) ;
#2588=VERTEX_POINT ( 'NONE', #1147 ) ;
#2589=CARTESIAN_POINT ( 'NONE',  ( -13.11366204365393706, -12.47935976348540876, 51.00231026484399166 ) ) ;
#2590=VERTEX_POINT ( 'NONE', #14850 ) ;
#2592=DIRECTION ( 'NONE',  ( -0.9437508163134049610, -0.3306575217771128283, -5.591929034707468788E-16 ) ) ;
#2595=PLANE ( 'NONE',  #14821 ) ;
#2596=CIRCLE ( 'NONE', #12859, 5.000000000000000000 ) ;
#2601=CARTESIAN_POINT ( 'NONE',  ( -12.32172653804166096, -7.186294389320899256, 56.85231026484398598 ) ) ;
#2602=ORIENTED_EDGE ( 'NONE', *, *, #9123, .T. ) ;
#2603=DIRECTION ( 'NONE',  ( 0.8160499452489450301, 0.5779813897169993053, 3.090169943749371762E-16 ) ) ;
#2604=ORIENTED_EDGE ( 'NONE', *, *, #5229, .T. ) ;
#2605=CARTESIAN_POINT ( 'NONE',  ( -16.73644428586258570, -23.40541355628489839, 54.00231026484399166 ) ) ;
#2606=ORIENTED_EDGE ( 'NONE', *, *, #9382, .F. ) ;
#2608=EDGE_CURVE ( 'NONE', #2877, #5325, #5510, .T. ) ;
#2609=DIRECTION ( 'NONE',  ( 0.5975035461963188466, 0.8018662683283437342, 0.000000000000000000 ) ) ;
#2610=EDGE_LOOP ( 'NONE', ( #10492, #4620, #10315, #14610 ) ) ;
#2611=EDGE_CURVE ( 'NONE', #7684, #5071, #5295, .T. ) ;
#2615=AXIS2_PLACEMENT_3D ( 'NONE', #848, #4214, #3056 ) ;
#2617=FACE_OUTER_BOUND ( 'NONE', #13816, .T. ) ;
#2618=CARTESIAN_POINT ( 'NONE',  ( -9.969334273478565933, -7.622966832294271633, 56.85231026484398598 ) ) ;
#2621=ORIENTED_EDGE ( 'NONE', *, *, #9185, .F. ) ;
#2623=ORIENTED_EDGE ( 'NONE', *, *, #8139, .F. ) ;
#2624=ADVANCED_FACE ( 'NONE', ( #8390 ), #3302, .T. ) ;
#2625=CARTESIAN_POINT ( 'NONE',  ( -23.09568838840838012, -16.24821979201191979, 56.85231026484398598 ) ) ;
#2626=EDGE_CURVE ( 'NONE', #11664, #6233, #10994, .T. ) ;
#2629=FACE_OUTER_BOUND ( 'NONE', #6185, .T. ) ;
#2631=PLANE ( 'NONE',  #12974 ) ;
#2632=AXIS2_PLACEMENT_3D ( 'NONE', #4679, #11632, #14083 ) ;
#2633=FACE_OUTER_BOUND ( 'NONE', #7296, .T. ) ;
#2634=( BOUNDED_CURVE ( )  B_SPLINE_CURVE ( 3, ( #12643, #6499, #10175, #4530 ),
 .UNSPECIFIED., .F., .F. ) 
 B_SPLINE_CURVE_WITH_KNOTS ( ( 4, 4 ),
 ( 4.712388980384688786, 6.283185307179585344 ),
 .UNSPECIFIED. ) 
 CURVE ( )  GEOMETRIC_REPRESENTATION_ITEM ( )  RATIONAL_B_SPLINE_CURVE ( ( 1.000000000000000000, 0.8047378541243648264, 0.8047378541243648264, 1.000000000000000000 ) ) 
 REPRESENTATION_ITEM ( '' )  );
#2636=CARTESIAN_POINT ( 'NONE',  ( -8.667632128016617088, -19.48099602858229318, 56.85231026484400019 ) ) ;
#2642=DIRECTION ( 'NONE',  ( 8.018662683283438208E-16, -5.975035461963189015E-16, -1.000000000000000000 ) ) ;
#2644=ORIENTED_EDGE ( 'NONE', *, *, #10067, .F. ) ;
#2645=VECTOR ( 'NONE', #11871, 1000.000000000000000 ) ;
#2649=EDGE_LOOP ( 'NONE', ( #3507, #9065, #989, #7814 ) ) ;
#2655=EDGE_CURVE ( 'NONE', #10807, #13936, #12394, .T. ) ;
#2661=ORIENTED_EDGE ( 'NONE', *, *, #12766, .F. ) ;
#2664=ORIENTED_EDGE ( 'NONE', *, *, #10952, .F. ) ;
#2666=ORIENTED_EDGE ( 'NONE', *, *, #5413, .T. ) ;
#2667=VECTOR ( 'NONE', #9721, 1000.000000000000000 ) ;
#2669=DIRECTION ( 'NONE',  ( -8.018662683283439195E-16, 5.975035461963190001E-16, 1.000000000000000000 ) ) ;
#2670=DIRECTION ( 'NONE',  ( 0.5196486895212287793, -0.8543800322332385511, 9.271838545667868842E-16 ) ) ;
#2671=LINE ( 'NONE', #1667, #4569 ) ;
#2672=EDGE_CURVE ( 'NONE', #6427, #12430, #5036, .T. ) ;
#2675=CARTESIAN_POINT ( 'NONE',  ( -9.539601987502633662, -5.508762965863004624, 48.00231026484398456 ) ) ;
#2677=DIRECTION ( 'NONE',  ( 0.4491835085186243748, 0.8934395198752397294, -1.736481776669301208E-16 ) ) ;
#2678=VERTEX_POINT ( 'NONE', #4890 ) ;
#2681=ORIENTED_EDGE ( 'NONE', *, *, #2574, .F. ) ;
#2682=DIRECTION ( 'NONE',  ( -8.018662683283438208E-16, 5.975035461963189015E-16, 1.000000000000000000 ) ) ;
#2684=ORIENTED_EDGE ( 'NONE', *, *, #11079, .F. ) ;
#2686=CARTESIAN_POINT ( 'NONE',  ( -9.031792552787402784, -10.63903015472409486, 56.85231026484400019 ) ) ;
#2697=ORIENTED_EDGE ( 'NONE', *, *, #14813, .F. ) ;
#2698=DIRECTION ( 'NONE',  ( 0.2640193276337003403, -0.9645173894937555392, 7.880107536067285830E-16 ) ) ;
#2703=ORIENTED_EDGE ( 'NONE', *, *, #10815, .F. ) ;
#2704=DIRECTION ( 'NONE',  ( -8.018662683283438208E-16, 5.975035461963189015E-16, 1.000000000000000000 ) ) ;
#2708=EDGE_CURVE ( 'NONE', #12018, #2885, #985, .T. ) ;
#2709=FACE_OUTER_BOUND ( 'NONE', #12674, .T. ) ;
#2711=CARTESIAN_POINT ( 'NONE',  ( -23.02734322232803521, -10.58405290357860373, 56.85231026484398598 ) ) ;
#2712=EDGE_CURVE ( 'NONE', #8545, #4445, #5330, .T. ) ;
#2715=VERTEX_POINT ( 'NONE', #10756 ) ;
#2718=ORIENTED_EDGE ( 'NONE', *, *, #11769, .F. ) ;
#2723=VECTOR ( 'NONE', #13130, 1000.000000000000000 ) ;
#2724=LINE ( 'NONE', #7382, #8735 ) ;
#2725=EDGE_CURVE ( 'NONE', #5304, #1083, #8572, .T. ) ;
#2726=ADVANCED_FACE ( 'NONE', ( #7425 ), #480, .T. ) ;
#2728=DIRECTION ( 'NONE',  ( -0.09252159378507134047, 0.9957106782009873536, -6.691306063588577540E-16 ) ) ;
#2731=DIRECTION ( 'NONE',  ( -8.018662683283439195E-16, 5.975035461963190001E-16, 1.000000000000000000 ) ) ;
#2732=ORIENTED_EDGE ( 'NONE', *, *, #7186, .T. ) ;
#2734=VECTOR ( 'NONE', #5531, 1000.000000000000114 ) ;
#2736=ORIENTED_EDGE ( 'NONE', *, *, #8421, .T. ) ;
#2737=DIRECTION ( 'NONE',  ( 0.5975035461963188466, 0.8018662683283437342, 0.000000000000000000 ) ) ;
#2738=ORIENTED_EDGE ( 'NONE', *, *, #9988, .F. ) ;
#2741=LINE ( 'NONE', #8320, #1351 ) ;
#2746=VECTOR ( 'NONE', #9832, 1000.000000000000000 ) ;
#2748=VECTOR ( 'NONE', #2369, 1000.000000000000000 ) ;
#2750=FACE_OUTER_BOUND ( 'NONE', #13309, .T. ) ;
#2751=ORIENTED_EDGE ( 'NONE', *, *, #6273, .T. ) ;
#2752=CARTESIAN_POINT ( 'NONE',  ( -7.064541492512761423, -18.83173137575486322, 56.85231026484400019 ) ) ;
#2758=ORIENTED_EDGE ( 'NONE', *, *, #14490, .T. ) ;
#2759=EDGE_LOOP ( 'NONE', ( #2926, #3220, #13340, #3548 ) ) ;
#2760=LINE ( 'NONE', #4055, #12772 ) ;
#2761=ORIENTED_EDGE ( 'NONE', *, *, #9743, .T. ) ;
#2766=CARTESIAN_POINT ( 'NONE',  ( -21.21771647519868154, -9.340181373223902739, 56.85231026484398598 ) ) ;
#2767=CARTESIAN_POINT ( 'NONE',  ( -25.46211945451987191, -14.00819915864900622, 57.00231026484397745 ) ) ;
#2768=CARTESIAN_POINT ( 'NONE',  ( -15.21745595230144232, -22.57829892241827352, 56.85231026484400019 ) ) ;
#2771=DIRECTION ( 'NONE',  ( -8.018662683283438208E-16, 5.975035461963189015E-16, 1.000000000000000000 ) ) ;
#2772=VECTOR ( 'NONE', #8211, 1000.000000000000000 ) ;
#2777=CARTESIAN_POINT ( 'NONE',  ( -23.54764701038621411, -12.84694604531765272, 56.85231026484398598 ) ) ;
#2778=EDGE_LOOP ( 'NONE', ( #7984, #14473, #2402, #2606 ) ) ;
#2779=CARTESIAN_POINT ( 'NONE',  ( -24.41321522311770664, -15.21339595774672127, 56.85231026484398598 ) ) ;
#2781=AXIS2_PLACEMENT_3D ( 'NONE', #13990, #1283, #9466 ) ;
#2783=LINE ( 'NONE', #11035, #11210 ) ;
#2788=VERTEX_POINT ( 'NONE', #4139 ) ;
#2792=VERTEX_POINT ( 'NONE', #7713 ) ;
#2793=EDGE_LOOP ( 'NONE', ( #597, #14137, #9046, #1905 ) ) ;
#2796=ORIENTED_EDGE ( 'NONE', *, *, #11028, .F. ) ;
#2797=EDGE_CURVE ( 'NONE', #7651, #13913, #11100, .T. ) ;
#2798=VECTOR ( 'NONE', #1411, 1000.000000000000000 ) ;
#2802=( GEOMETRIC_REPRESENTATION_CONTEXT ( 3 ) GLOBAL_UNCERTAINTY_ASSIGNED_CONTEXT ( ( #10126 ) ) GLOBAL_UNIT_ASSIGNED_CONTEXT ( ( #5799, #10475, #4817 ) ) REPRESENTATION_CONTEXT ( 'NONE', 'WORKASPACE' ) );
#2807=VERTEX_POINT ( 'NONE', #8794 ) ;
#2808=PLANE ( 'NONE',  #3113 ) ;
#2811=CARTESIAN_POINT ( 'NONE',  ( -7.707227416580196611, -8.855645637450560770, 57.00231026484399166 ) ) ;
#2812=DIRECTION ( 'NONE',  ( 0.5975035461963188466, 0.8018662683283437342, 0.000000000000000000 ) ) ;
#2816=LINE ( 'NONE', #7545, #13496 ) ;
#2817=AXIS2_PLACEMENT_3D ( 'NONE', #2314, #12875, #11713 ) ;
#2819=EDGE_CURVE ( 'NONE', #8808, #11708, #11634, .T. ) ;
#2820=FACE_BOUND ( 'NONE', #10503, .T. ) ;
#2824=ORIENTED_EDGE ( 'NONE', *, *, #4138, .T. ) ;
#2825=LINE ( 'NONE', #11308, #9943 ) ;
#2827=VERTEX_POINT ( 'NONE', #4369 ) ;
#2831=VERTEX_POINT ( 'NONE', #5505 ) ;
#2832=DIRECTION ( 'NONE',  ( -0.4274949678123838859, 0.9040177279761104634, -8.829475928589268008E-16 ) ) ;
#2834=CARTESIAN_POINT ( 'NONE',  ( -15.49969986081091200, -13.50737899243823215, 48.00231026484398456 ) ) ;
#2835=CIRCLE ( 'NONE', #5516, 9.974999999999999645 ) ;
#2837=CARTESIAN_POINT ( 'NONE',  ( -20.52642601085533869, -22.12321610861327770, 57.00231026484397745 ) ) ;
#2839=DIRECTION ( 'NONE',  ( -8.018662683283438208E-16, 5.975035461963189015E-16, 1.000000000000000000 ) ) ;
#2841=FACE_OUTER_BOUND ( 'NONE', #3843, .T. ) ;
#2842=VERTEX_POINT ( 'NONE', #11323 ) ;
#2845=ORIENTED_EDGE ( 'NONE', *, *, #2611, .T. ) ;
#2847=ORIENTED_EDGE ( 'NONE', *, *, #3607, .F. ) ;
#2848=DIRECTION ( 'NONE',  ( 0.5975035461963189576, 0.8018662683283437342, 0.000000000000000000 ) ) ;
#2850=CARTESIAN_POINT ( 'NONE',  ( -5.650856670168519003, -15.08880645082409444, 56.85231026484400019 ) ) ;
#2851=VECTOR ( 'NONE', #4285, 1000.000000000000114 ) ;
#2853=VECTOR ( 'NONE', #3921, 1000.000000000000000 ) ;
#2855=EDGE_CURVE ( 'NONE', #1460, #9210, #922, .T. ) ;
#2856=DIRECTION ( 'NONE',  ( 0.5975035461963189576, 0.8018662683283437342, 0.000000000000000000 ) ) ;
#2862=FACE_OUTER_BOUND ( 'NONE', #13166, .T. ) ;
#2863=VERTEX_POINT ( 'NONE', #14771 ) ;
#2864=VERTEX_POINT ( 'NONE', #14918 ) ;
#2867=VECTOR ( 'NONE', #9635, 1000.000000000000000 ) ;
#2870=DIRECTION ( 'NONE',  ( 0.5975035461963188466, 0.8018662683283437342, 0.000000000000000000 ) ) ;
#2871=DIRECTION ( 'NONE',  ( -0.5401126942952660936, -0.8415927028326163351, 6.975647374412055055E-17 ) ) ;
#2874=EDGE_CURVE ( 'NONE', #6427, #6628, #13103, .T. ) ;
#2877=VERTEX_POINT ( 'NONE', #9096 ) ;
#2878=LINE ( 'NONE', #7536, #917 ) ;
#2879=CARTESIAN_POINT ( 'NONE',  ( -22.94870171817393256, -18.69135635822624053, 56.85231026484398598 ) ) ;
#2883=ORIENTED_EDGE ( 'NONE', *, *, #6078, .T. ) ;
#2884=DIRECTION ( 'NONE',  ( -8.018662683283438208E-16, 5.975035461963189015E-16, 1.000000000000000000 ) ) ;
#2885=VERTEX_POINT ( 'NONE', #12398 ) ;
#2886=DIRECTION ( 'NONE',  ( -8.018662683283438208E-16, 5.975035461963189015E-16, 1.000000000000000000 ) ) ;
#2888=CARTESIAN_POINT ( 'NONE',  ( -25.26605094763165482, -15.53691377877616553, 56.85231026484398598 ) ) ;
#2891=AXIS2_PLACEMENT_3D ( 'NONE', #7284, #11970, #495 ) ;
#2892=LINE ( 'NONE', #831, #11147 ) ;
#2894=DIRECTION ( 'NONE',  ( -8.018662683283438208E-16, 5.975035461963189015E-16, 1.000000000000000000 ) ) ;
#2895=ORIENTED_EDGE ( 'NONE', *, *, #979, .F. ) ;
#2900=ADVANCED_FACE ( 'NONE', ( #1295 ), #7942, .T. ) ;
#2901=VERTEX_POINT ( 'NONE', #6866 ) ;
#2905=ORIENTED_EDGE ( 'NONE', *, *, #1394, .F. ) ;
#2908=VERTEX_POINT ( 'NONE', #2220 ) ;
#2911=DIRECTION ( 'NONE',  ( -8.018662683283438208E-16, 5.975035461963189015E-16, 1.000000000000000000 ) ) ;
#2912=DIRECTION ( 'NONE',  ( -8.018662683283438208E-16, 5.975035461963189015E-16, 1.000000000000000000 ) ) ;
#2914=DIRECTION ( 'NONE',  ( 0.7109061395677488404, -0.7032868978765923762, 9.902680687415717796E-16 ) ) ;
#2916=VECTOR ( 'NONE', #3307, 1000.000000000000114 ) ;
#2917=CIRCLE ( 'NONE', #4141, 9.974999999999999645 ) ;
#2919=EDGE_LOOP ( 'NONE', ( #31, #10350, #3578, #12871 ) ) ;
#2921=CARTESIAN_POINT ( 'NONE',  ( -5.615565924346637594, -12.16405426399944645, 57.00231026484399166 ) ) ;
#2922=ORIENTED_EDGE ( 'NONE', *, *, #1085, .F. ) ;
#2924=DIRECTION ( 'NONE',  ( -0.4491835085186243748, -0.8934395198752397294, 1.736481776669299976E-16 ) ) ;
#2925=VERTEX_POINT ( 'NONE', #3591 ) ;
#2926=ORIENTED_EDGE ( 'NONE', *, *, #979, .T. ) ;
#2927=DIRECTION ( 'NONE',  ( 0.08178736187250883194, 0.9966498018049948504, -5.299192642332142575E-16 ) ) ;
#2929=VERTEX_POINT ( 'NONE', #8090 ) ;
#2931=VECTOR ( 'NONE', #12822, 1000.000000000000000 ) ;
#2933=CARTESIAN_POINT ( 'NONE',  ( -25.26605094763165482, -15.53691377877616553, 57.00231026484397745 ) ) ;
#2936=CARTESIAN_POINT ( 'NONE',  ( -15.51120972694785749, -13.45872179377749589, 56.85231026484398598 ) ) ;
#2937=DIRECTION ( 'NONE',  ( -0.2975196656470009415, 0.9547156899063180546, -8.090169943749472730E-16 ) ) ;
#2940=CARTESIAN_POINT ( 'NONE',  ( -15.49969986081092088, -13.50737899243822504, 57.00231026484397745 ) ) ;
#2941=VERTEX_POINT ( 'NONE', #2375 ) ;
#2945=CARTESIAN_POINT ( 'NONE',  ( -22.80943503306988873, -20.29474937510043020, 56.85231026484398598 ) ) ;
#2946=VECTOR ( 'NONE', #1933, 1000.000000000000000 ) ;
#2952=ORIENTED_EDGE ( 'NONE', *, *, #5790, .T. ) ;
#2953=FACE_OUTER_BOUND ( 'NONE', #7582, .T. ) ;
#2955=ORIENTED_EDGE ( 'NONE', *, *, #7732, .T. ) ;
#2956=DIRECTION ( 'NONE',  ( 0.5975035461963189576, 0.8018662683283437342, 0.000000000000000000 ) ) ;
#2957=LINE ( 'NONE', #10920, #14262 ) ;
#2959=CARTESIAN_POINT ( 'NONE',  ( -16.34789837066772122, -3.568506607309356315, 57.00231026484397745 ) ) ;
#2960=VECTOR ( 'NONE', #3270, 1000.000000000000000 ) ;
#2961=EDGE_CURVE ( 'NONE', #14007, #2929, #8208, .T. ) ;
#2963=EDGE_CURVE ( 'NONE', #6250, #15017, #7089, .T. ) ;
#2965=CARTESIAN_POINT ( 'NONE',  ( -7.517426579539127296, -14.72759957212633530, 56.85231026484400019 ) ) ;
#2966=LINE ( 'NONE', #13460, #5009 ) ;
#2968=LINE ( 'NONE', #3975, #14595 ) ;
#2970=AXIS2_PLACEMENT_3D ( 'NONE', #9734, #11104, #2771 ) ;
#2977=LINE ( 'NONE', #1835, #1938 ) ;
#2978=EDGE_CURVE ( 'NONE', #2807, #9210, #10477, .T. ) ;
#2979=AXIS2_PLACEMENT_3D ( 'NONE', #11130, #4017, #5159 ) ;
#2980=LINE ( 'NONE', #11391, #9083 ) ;
#2983=CIRCLE ( 'NONE', #1276, 9.974999999999999645 ) ;
#2985=AXIS2_PLACEMENT_3D ( 'NONE', #1917, #7568, #14765 ) ;
#2986=EDGE_CURVE ( 'NONE', #1083, #6348, #6, .T. ) ;
#2987=LINE ( 'NONE', #6194, #3828 ) ;
#2988=DIRECTION ( 'NONE',  ( -0.4800904676395363335, -0.8772189822852964891, 1.391731009600659432E-16 ) ) ;
#2990=EDGE_CURVE ( 'NONE', #9086, #4893, #11393, .T. ) ;
#2991=DIRECTION ( 'NONE',  ( -0.8018662683283438453, 0.5975035461963189576, -1.000000000000000275E-15 ) ) ;
#2994=EDGE_LOOP ( 'NONE', ( #7895, #7935, #14871, #4050 ) ) ;
#2998=CIRCLE ( 'NONE', #7875, 4.999999999999999112 ) ;
#3000=LINE ( 'NONE', #13487, #1809 ) ;
#3008=PLANE ( 'NONE',  #14727 ) ;
#3009=ORIENTED_EDGE ( 'NONE', *, *, #10032, .T. ) ;
#3011=DIRECTION ( 'NONE',  ( -8.018662683283439195E-16, 5.975035461963190001E-16, 1.000000000000000000 ) ) ;
#3012=ORIENTED_EDGE ( 'NONE', *, *, #11136, .F. ) ;
#3013=ORIENTED_EDGE ( 'NONE', *, *, #8586, .F. ) ;
#3015=CARTESIAN_POINT ( 'NONE',  ( -21.23124220554638697, -20.54376104222092181, 56.85231026484398598 ) ) ;
#3016=ORIENTED_EDGE ( 'NONE', *, *, #4783, .F. ) ;
#3017=LINE ( 'NONE', #7675, #2746 ) ;
#3018=VECTOR ( 'NONE', #13674, 1000.000000000000227 ) ;
#3019=DIRECTION ( 'NONE',  ( 0.7109061395677416240, -0.7032868978765995926, 9.902680687415702019E-16 ) ) ;
#3023=DIRECTION ( 'NONE',  ( 0.2975196656470014966, -0.9547156899063178326, 8.090169943749475688E-16 ) ) ;
#3024=EDGE_LOOP ( 'NONE', ( #6929, #6851, #1300, #1195 ) ) ;
#3025=LINE ( 'NONE', #10212, #5091 ) ;
#3026=DIRECTION ( 'NONE',  ( -8.018662683283439195E-16, 5.975035461963190001E-16, 1.000000000000000000 ) ) ;
#3029=DIRECTION ( 'NONE',  ( 8.018662683283438208E-16, -5.975035461963189015E-16, -1.000000000000000000 ) ) ;
#3030=EDGE_CURVE ( 'NONE', #6106, #1455, #1372, .T. ) ;
#3031=LINE ( 'NONE', #7688, #5185 ) ;
#3032=DIRECTION ( 'NONE',  ( 8.018662683283438208E-16, -5.975035461963189015E-16, -1.000000000000000000 ) ) ;
#3033=CARTESIAN_POINT ( 'NONE',  ( -19.19431052208641475, -4.241825740657185762, 57.00231026484397745 ) ) ;
#3037=VECTOR ( 'NONE', #3042, 1000.000000000000114 ) ;
#3041=CARTESIAN_POINT ( 'NONE',  ( -20.44787060326519068, -4.846187890544673138, 54.00231026484397745 ) ) ;
#3042=DIRECTION ( 'NONE',  ( 0.05771543059946734194, -0.9983330752162417054, 6.427876096865391919E-16 ) ) ;
#3043=ORIENTED_EDGE ( 'NONE', *, *, #4422, .T. ) ;
#3046=AXIS2_PLACEMENT_3D ( 'NONE', #8975, #12741, #9282 ) ;
#3049=PLANE ( 'NONE',  #2039 ) ;
#3051=VERTEX_POINT ( 'NONE', #7242 ) ;
#3052=CARTESIAN_POINT ( 'NONE',  ( -19.51793069539949599, -6.502732608789604463, 56.85231026484398598 ) ) ;
#3053=LINE ( 'NONE', #2215, #6783 ) ;
#3056=DIRECTION ( 'NONE',  ( -8.018662683283438208E-16, 5.975035461963189015E-16, 1.000000000000000000 ) ) ;
#3061=EDGE_LOOP ( 'NONE', ( #2262, #12581, #11511, #12338 ) ) ;
#3062=CARTESIAN_POINT ( 'NONE',  ( -17.14283461285079824, -15.71251123034117114, 56.75231026484397745 ) ) ;
#3063=ORIENTED_EDGE ( 'NONE', *, *, #8645, .F. ) ;
#3065=DIRECTION ( 'NONE',  ( 0.5975035461963189576, 0.8018662683283437342, 0.000000000000000000 ) ) ;
#3066=DIRECTION ( 'NONE',  ( -0.8018662683283436232, 0.5975035461963189576, -9.999999999999996833E-16 ) ) ;
#3068=ORIENTED_EDGE ( 'NONE', *, *, #14490, .F. ) ;
#3069=EDGE_CURVE ( 'NONE', #8039, #9794, #11002, .T. ) ;
#3072=ORIENTED_EDGE ( 'NONE', *, *, #10681, .F. ) ;
#3073=AXIS2_PLACEMENT_3D ( 'NONE', #1122, #15045, #2356 ) ;
#3075=DIRECTION ( 'NONE',  ( -8.018662683283438208E-16, 5.975035461963189015E-16, 1.000000000000000000 ) ) ;
#3079=CARTESIAN_POINT ( 'NONE',  ( -13.74242962142780478, -4.603826257390357668, 56.85231026484398598 ) ) ;
#3080=EDGE_CURVE ( 'NONE', #11463, #5367, #310, .T. ) ;
#3085=DIRECTION ( 'NONE',  ( -8.018662683283438208E-16, 5.975035461963189015E-16, 1.000000000000000000 ) ) ;
#3086=EDGE_LOOP ( 'NONE', ( #7544, #10735, #814, #1230 ) ) ;
#3088=EDGE_CURVE ( 'NONE', #14012, #8291, #639, .T. ) ;
#3092=VECTOR ( 'NONE', #10927, 1000.000000000000227 ) ;
#3096=CARTESIAN_POINT ( 'NONE',  ( -17.05536012119625866, -6.605120582739408164, 56.85231026484398598 ) ) ;
#3103=LINE ( 'NONE', #6460, #11449 ) ;
#3104=ORIENTED_EDGE ( 'NONE', *, *, #391, .T. ) ;
#3105=PLANE ( 'NONE',  #8343 ) ;
#3107=DIRECTION ( 'NONE',  ( 0.3306575217771128283, -0.9437508163134049610, 8.290375725550417844E-16 ) ) ;
#3108=VERTEX_POINT ( 'NONE', #4269 ) ;
#3113=AXIS2_PLACEMENT_3D ( 'NONE', #12442, #14433, #7612 ) ;
#3115=EDGE_CURVE ( 'NONE', #9104, #858, #7840, .T. ) ;
#3118=LINE ( 'NONE', #3041, #1856 ) ;
#3119=CARTESIAN_POINT ( 'NONE',  ( -24.28571865450477674, -8.784403367172062715, 56.85231026484398598 ) ) ;
#3124=ORIENTED_EDGE ( 'NONE', *, *, #12067, .F. ) ;
#3125=VECTOR ( 'NONE', #65, 1000.000000000000114 ) ;
#3126=VECTOR ( 'NONE', #2415, 1000.000000000000000 ) ;
#3129=ORIENTED_EDGE ( 'NONE', *, *, #12134, .F. ) ;
#3131=AXIS2_PLACEMENT_3D ( 'NONE', #3914, #12250, #1764 ) ;
#3135=FACE_OUTER_BOUND ( 'NONE', #9444, .T. ) ;
#3136=EDGE_CURVE ( 'NONE', #11163, #13353, #2596, .T. ) ;
#3140=LINE ( 'NONE', #3296, #7279 ) ;
#3144=EDGE_LOOP ( 'NONE', ( #9522, #4695, #6183, #11406 ) ) ;
#3145=ORIENTED_EDGE ( 'NONE', *, *, #12244, .T. ) ;
#3146=ORIENTED_EDGE ( 'NONE', *, *, #14446, .T. ) ;
#3147=LINE ( 'NONE', #2159, #11537 ) ;
#3148=DIRECTION ( 'NONE',  ( 8.018662683283438208E-16, -5.975035461963189015E-16, -1.000000000000000000 ) ) ;
#3150=ORIENTED_EDGE ( 'NONE', *, *, #10794, .F. ) ;
#3151=DIRECTION ( 'NONE',  ( -8.018662683283438208E-16, 5.975035461963189015E-16, 1.000000000000000000 ) ) ;
#3152=ADVANCED_FACE ( 'NONE', ( #14751 ), #1825, .T. ) ;
#3156=VECTOR ( 'NONE', #7428, 1000.000000000000000 ) ;
#3158=DIRECTION ( 'NONE',  ( -0.9731439732146149879, -0.2301973227387160703, -6.427876096865396850E-16 ) ) ;
#3163=DIRECTION ( 'NONE',  ( -8.018662683283438208E-16, 5.975035461963189015E-16, 1.000000000000000000 ) ) ;
#3165=VERTEX_POINT ( 'NONE', #6470 ) ;
#3170=AXIS2_PLACEMENT_3D ( 'NONE', #10836, #10678, #10606 ) ;
#3171=DIRECTION ( 'NONE',  ( -8.018662683283438208E-16, 5.975035461963189015E-16, 1.000000000000000000 ) ) ;
#3174=ADVANCED_FACE ( 'NONE', ( #4192 ), #4351, .F. ) ;
#3176=EDGE_CURVE ( 'NONE', #8000, #10077, #2892, .T. ) ;
#3177=LINE ( 'NONE', #5169, #10359 ) ;
#3179=CARTESIAN_POINT ( 'NONE',  ( -5.898712304418588737, -10.80152183767200214, 57.00231026484399166 ) ) ;
#3181=DIRECTION ( 'NONE',  ( 8.018662683283438208E-16, -5.975035461963189015E-16, -1.000000000000000000 ) ) ;
#3182=DIRECTION ( 'NONE',  ( -0.7737441449604661736, -0.6334982226805353500, -2.419218955996689845E-16 ) ) ;
#3185=EDGE_CURVE ( 'NONE', #1753, #14533, #3118, .T. ) ;
#3186=VERTEX_POINT ( 'NONE', #673 ) ;
#3187=DIRECTION ( 'NONE',  ( -0.9472588896649093426, 0.3204693369899890287, -9.510565162951525763E-16 ) ) ;
#3189=CARTESIAN_POINT ( 'NONE',  ( -13.18491133144367922, -15.23222315862922471, 56.75231026484399166 ) ) ;
#3190=LINE ( 'NONE', #4563, #8642 ) ;
#3198=ORIENTED_EDGE ( 'NONE', *, *, #13195, .F. ) ;
#3201=CARTESIAN_POINT ( 'NONE',  ( -19.45253106704483770, -6.466019006254929202, 57.00231026484397745 ) ) ;
#3203=CARTESIAN_POINT ( 'NONE',  ( -5.628190034013325516, -14.94052892857136250, 56.85231026484400019 ) ) ;
#3205=VERTEX_POINT ( 'NONE', #2050 ) ;
#3206=VECTOR ( 'NONE', #4644, 1000.000000000000000 ) ;
#3207=ADVANCED_FACE ( 'NONE', ( #5340 ), #14673, .F. ) ;
#3208=DIRECTION ( 'NONE',  ( 8.018662683283438208E-16, -5.975035461963189015E-16, -1.000000000000000000 ) ) ;
#3209=DIRECTION ( 'NONE',  ( 0.9997391571607664451, 0.02283895005205794498, 7.880107536067222722E-16 ) ) ;
#3210=CARTESIAN_POINT ( 'NONE',  ( -24.41321522311770664, -15.21339595774672127, 56.85231026484398598 ) ) ;
#3214=AXIS2_PLACEMENT_3D ( 'NONE', #1769, #7426, #12106 ) ;
#3217=CARTESIAN_POINT ( 'NONE',  ( -8.858895634567669930, -20.95051974273373929, 56.85231026484400019 ) ) ;
#3218=EDGE_LOOP ( 'NONE', ( #5826, #2203, #8296, #12869 ) ) ;
#3220=ORIENTED_EDGE ( 'NONE', *, *, #2479, .F. ) ;
#3221=DIRECTION ( 'NONE',  ( 0.5975035461963189576, 0.8018662683283437342, 0.000000000000000000 ) ) ;
#3224=ORIENTED_EDGE ( 'NONE', *, *, #662, .T. ) ;
#3225=EDGE_CURVE ( 'NONE', #13665, #8073, #403, .T. ) ;
#3230=AXIS2_PLACEMENT_3D ( 'NONE', #6318, #2886, #3889 ) ;
#3232=AXIS2_PLACEMENT_3D ( 'NONE', #1654, #3726, #7226 ) ;
#3233=CYLINDRICAL_SURFACE ( 'NONE', #9037, 5.000000000000000000 ) ;
#3236=VECTOR ( 'NONE', #2065, 1000.000000000000000 ) ;
#3241=CARTESIAN_POINT ( 'NONE',  ( -15.49969986081091733, -13.50737899243822682, 54.00231026484399166 ) ) ;
#3245=CARTESIAN_POINT ( 'NONE',  ( -10.27295246487022240, -6.088325032597582620, 57.00231026484397745 ) ) ;
#3251=ORIENTED_EDGE ( 'NONE', *, *, #4614, .T. ) ;
#3252=DIRECTION ( 'NONE',  ( -8.018662683283438208E-16, 5.975035461963189015E-16, 1.000000000000000000 ) ) ;
#3253=VECTOR ( 'NONE', #5654, 1000.000000000000000 ) ;
#3254=CARTESIAN_POINT ( 'NONE',  ( -7.985436018829471294, -20.06759727486528178, 56.85231026484400019 ) ) ;
#3256=DIRECTION ( 'NONE',  ( 0.4224988092984268695, 0.5670050759397228246, -0.7071067811865479058 ) ) ;
#3258=LINE ( 'NONE', #6833, #10086 ) ;
#3260=ORIENTED_EDGE ( 'NONE', *, *, #14867, .F. ) ;
#3261=CARTESIAN_POINT ( 'NONE',  ( -21.12809094326923187, -9.219901432974651811, 56.85231026484398598 ) ) ;
#3263=ORIENTED_EDGE ( 'NONE', *, *, #1396, .T. ) ;
#3265=CARTESIAN_POINT ( 'NONE',  ( -23.59767874945767119, -17.60420555931063902, 56.85231026484398598 ) ) ;
#3266=EDGE_CURVE ( 'NONE', #13470, #8005, #7998, .T. ) ;
#3267=DIRECTION ( 'NONE',  ( 8.018662683283438208E-16, -5.975035461963189015E-16, -1.000000000000000000 ) ) ;
#3268=AXIS2_PLACEMENT_3D ( 'NONE', #6836, #1041, #6908 ) ;
#3270=DIRECTION ( 'NONE',  ( 8.018662683283438208E-16, -5.975035461963189015E-16, -1.000000000000000000 ) ) ;
#3271=EDGE_CURVE ( 'NONE', #13499, #6704, #12610, .T. ) ;
#3272=PLANE ( 'NONE',  #4638 ) ;
#3273=EDGE_CURVE ( 'NONE', #14032, #7250, #1200, .T. ) ;
#3275=DIRECTION ( 'NONE',  ( -0.9183863840214729901, -0.3956847857120157075, -4.999999999999999402E-16 ) ) ;
#3280=CARTESIAN_POINT ( 'NONE',  ( -21.18752042047970363, -7.775019331617081697, 56.85231026484398598 ) ) ;
#3282=CARTESIAN_POINT ( 'NONE',  ( -23.54290256004220439, -7.607589560680600549, 54.00231026484397745 ) ) ;
#3284=EDGE_CURVE ( 'NONE', #5304, #5925, #3325, .T. ) ;
#3286=CARTESIAN_POINT ( 'NONE',  ( -7.307539508764906877, -16.04208977798462854, 56.85231026484400019 ) ) ;
#3287=ORIENTED_EDGE ( 'NONE', *, *, #8298, .T. ) ;
#3288=VECTOR ( 'NONE', #5409, 1000.000000000000114 ) ;
#3291=CARTESIAN_POINT ( 'NONE',  ( -18.48721759179251123, -17.51671033407994926, 51.00231026484399166 ) ) ;
#3293=CARTESIAN_POINT ( 'NONE',  ( -24.85752488709640673, -10.05314452190415331, 57.00231026484397745 ) ) ;
#3296=CARTESIAN_POINT ( 'NONE',  ( -9.884208147447516524, -5.263176313152192698, 54.00231026484399166 ) ) ;
#3297=CARTESIAN_POINT ( 'NONE',  ( -25.45346213993001783, -14.15794911993140026, 56.85231026484398598 ) ) ;
#3300=EDGE_CURVE ( 'NONE', #14388, #10152, #4549, .T. ) ;
#3301=ORIENTED_EDGE ( 'NONE', *, *, #6272, .T. ) ;
#3302=PLANE ( 'NONE',  #10928 ) ;
#3305=ORIENTED_EDGE ( 'NONE', *, *, #1603, .T. ) ;
#3306=VERTEX_POINT ( 'NONE', #3344 ) ;
#3307=DIRECTION ( 'NONE',  ( -0.9805849309054472940, -0.1960948578651647567, -6.691306063588586415E-16 ) ) ;
#3308=CIRCLE ( 'NONE', #11851, 9.974999999999997868 ) ;
#3312=VERTEX_POINT ( 'NONE', #14901 ) ;
#3314=VERTEX_POINT ( 'NONE', #9151 ) ;
#3317=CARTESIAN_POINT ( 'NONE',  ( -19.06972223273333711, -21.85101071153832919, 56.85231026484400019 ) ) ;
#3318=ORIENTED_EDGE ( 'NONE', *, *, #15084, .T. ) ;
#3319=ORIENTED_EDGE ( 'NONE', *, *, #5742, .T. ) ;
#3322=DIRECTION ( 'NONE',  ( 8.018662683283438208E-16, -5.975035461963189015E-16, -1.000000000000000000 ) ) ;
#3323=PLANE ( 'NONE',  #3046 ) ;
#3325=CIRCLE ( 'NONE', #4060, 9.974999999999999645 ) ;
#3327=CARTESIAN_POINT ( 'NONE',  ( -17.86883904694317593, -3.817807045405069655, 57.00231026484397745 ) ) ;
#3328=CARTESIAN_POINT ( 'NONE',  ( -8.430459378593662123, -7.816413432484393020, 57.00231026484399166 ) ) ;
#3332=LINE ( 'NONE', #14045, #3993 ) ;
#3333=VERTEX_POINT ( 'NONE', #8155 ) ;
#3337=DIRECTION ( 'NONE',  ( 0.5975035461963188466, 0.8018662683283437342, 0.000000000000000000 ) ) ;
#3338=ORIENTED_EDGE ( 'NONE', *, *, #3451, .F. ) ;
#3339=DIRECTION ( 'NONE',  ( 0.9966498018049947394, -0.08178736187250883194, 8.480480961564201844E-16 ) ) ;
#3342=LINE ( 'NONE', #13753, #15071 ) ;
#3343=VECTOR ( 'NONE', #11301, 1000.000000000000000 ) ;
#3344=CARTESIAN_POINT ( 'NONE',  ( -15.19545581216392627, -5.437764035151672282, 57.00231026484397745 ) ) ;
#3345=DIRECTION ( 'NONE',  ( 0.9931883319083343320, -0.1165201156931299220, 0.000000000000000000 ) ) ;
#3346=EDGE_CURVE ( 'NONE', #4275, #1606, #13114, .T. ) ;
#3347=ORIENTED_EDGE ( 'NONE', *, *, #8737, .T. ) ;
#3351=VECTOR ( 'NONE', #7949, 1000.000000000000000 ) ;
#3356=PLANE ( 'NONE',  #10321 ) ;
#3358=VECTOR ( 'NONE', #9461, 1000.000000000000000 ) ;
#3359=EDGE_CURVE ( 'NONE', #6669, #413, #13905, .T. ) ;
#3361=CARTESIAN_POINT ( 'NONE',  ( -5.923714809816990723, -16.30043024566306187, 56.85231026484400019 ) ) ;
#3362=CARTESIAN_POINT ( 'NONE',  ( -9.539601987502633662, -5.508762965863004624, 48.00231026484398456 ) ) ;
#3363=ADVANCED_FACE ( 'NONE', ( #5558 ), #13826, .T. ) ;
#3367=EDGE_CURVE ( 'NONE', #4531, #9738, #6771, .T. ) ;
#3369=VECTOR ( 'NONE', #11512, 1000.000000000000000 ) ;
#3372=AXIS2_PLACEMENT_3D ( 'NONE', #6454, #13511, #7752 ) ;
#3373=ORIENTED_EDGE ( 'NONE', *, *, #7991, .F. ) ;
#3374=LINE ( 'NONE', #8255, #11281 ) ;
#3376=DIRECTION ( 'NONE',  ( 0.9805849309054470719, 0.1960948578651654506, 6.691306063588581484E-16 ) ) ;
#3377=ORIENTED_EDGE ( 'NONE', *, *, #568, .T. ) ;
#3381=ORIENTED_EDGE ( 'NONE', *, *, #7456, .T. ) ;
#3386=EDGE_CURVE ( 'NONE', #11066, #5017, #12616, .T. ) ;
#3387=EDGE_CURVE ( 'NONE', #8000, #1003, #2835, .T. ) ;
#3388=EDGE_LOOP ( 'NONE', ( #12923, #11052, #857, #12832 ) ) ;
#3391=ORIENTED_EDGE ( 'NONE', *, *, #14678, .T. ) ;
#3394=EDGE_LOOP ( 'NONE', ( #11502, #10470, #13969, #14163 ) ) ;
#3396=DIRECTION ( 'NONE',  ( -8.018662683283438208E-16, 5.975035461963189015E-16, 1.000000000000000000 ) ) ;
#3400=ADVANCED_FACE ( 'NONE', ( #439 ), #1354, .F. ) ;
#3401=AXIS2_PLACEMENT_3D ( 'NONE', #1059, #12777, #5718 ) ;
#3402=CARTESIAN_POINT ( 'NONE',  ( -24.21370508435883906, -8.652820519829269585, 56.85231026484398598 ) ) ;
#3404=CARTESIAN_POINT ( 'NONE',  ( -15.51120972694785749, -13.45872179377749589, 56.85231026484398598 ) ) ;
#3406=VERTEX_POINT ( 'NONE', #371 ) ;
#3407=CARTESIAN_POINT ( 'NONE',  ( -5.596483669297567687, -12.31283553816471610, 54.00231026484399166 ) ) ;
#3408=CIRCLE ( 'NONE', #13917, 9.974999999999999645 ) ;
#3409=CARTESIAN_POINT ( 'NONE',  ( -13.88982576282654691, -4.575998618238553917, 56.85231026484398598 ) ) ;
#3410=EDGE_LOOP ( 'NONE', ( #7448, #14536, #13432, #9681 ) ) ;
#3412=ORIENTED_EDGE ( 'NONE', *, *, #11526, .T. ) ;
#3413=PLANE ( 'NONE',  #792 ) ;
#3414=LINE ( 'NONE', #1967, #1273 ) ;
#3415=DIRECTION ( 'NONE',  ( -0.9999272109403024578, 0.01206535623791937274, -8.090169943749475688E-16 ) ) ;
#3416=VERTEX_POINT ( 'NONE', #6005 ) ;
#3418=ADVANCED_FACE ( 'NONE', ( #9687 ), #9611, .T. ) ;
#3420=LINE ( 'NONE', #8070, #1899 ) ;
#3421=CARTESIAN_POINT ( 'NONE',  ( -16.32407967933980686, -20.53418644068968746, 56.85231026484400019 ) ) ;
#3423=VECTOR ( 'NONE', #14036, 1000.000000000000000 ) ;
#3427=PLANE ( 'NONE',  #9129 ) ;
#3428=CARTESIAN_POINT ( 'NONE',  ( -20.48903913017556633, -19.85700446605285308, 56.85231026484398598 ) ) ;
#3430=ORIENTED_EDGE ( 'NONE', *, *, #282, .T. ) ;
#3431=EDGE_CURVE ( 'NONE', #13608, #13647, #1271, .T. ) ;
#3432=CARTESIAN_POINT ( 'NONE',  ( -15.45378054160984682, -13.48759475315262613, 56.85231026484398598 ) ) ;
#3433=CARTESIAN_POINT ( 'NONE',  ( -8.703838785437527648, -17.86878899887247130, 56.85231026484400019 ) ) ;
#3437=CARTESIAN_POINT ( 'NONE',  ( -9.376966593418606166, -18.77214511605354019, 56.85231026484400019 ) ) ;
#3438=CARTESIAN_POINT ( 'NONE',  ( -17.81448839017816610, -11.78253482624722537, 51.25231026484399166 ) ) ;
#3441=PLANE ( 'NONE',  #6165 ) ;
#3449=ADVANCED_FACE ( 'NONE', ( #10683 ), #8303, .F. ) ;
#3451=EDGE_CURVE ( 'NONE', #9434, #11163, #5028, .T. ) ;
#3452=VERTEX_POINT ( 'NONE', #289 ) ;
#3454=CARTESIAN_POINT ( 'NONE',  ( -23.52886110248590867, -17.73748770914800943, 57.00231026484397745 ) ) ;
#3455=AXIS2_PLACEMENT_3D ( 'NONE', #10736, #3339, #2197 ) ;
#3456=DIRECTION ( 'NONE',  ( -8.018662683283438208E-16, 5.975035461963189015E-16, 1.000000000000000000 ) ) ;
#3458=CARTESIAN_POINT ( 'NONE',  ( -20.45368390747784204, -7.130130991507916072, 56.85231026484398598 ) ) ;
#3459=VECTOR ( 'NONE', #631, 1000.000000000000114 ) ;
#3463=PLANE ( 'NONE',  #8955 ) ;
#3464=ORIENTED_EDGE ( 'NONE', *, *, #15043, .F. ) ;
#3465=ORIENTED_EDGE ( 'NONE', *, *, #3284, .F. ) ;
#3466=VECTOR ( 'NONE', #3902, 1000.000000000000227 ) ;
#3468=FACE_OUTER_BOUND ( 'NONE', #13387, .T. ) ;
#3471=PLANE ( 'NONE',  #7869 ) ;
#3474=CARTESIAN_POINT ( 'NONE',  ( -22.42051587769119791, -8.443926053929422082, 57.00231026484397745 ) ) ;
#3476=VECTOR ( 'NONE', #4225, 1000.000000000000000 ) ;
#3478=CARTESIAN_POINT ( 'NONE',  ( -15.49969986081092088, -13.50737899243822504, 57.00231026484397745 ) ) ;
#3479=DIRECTION ( 'NONE',  ( -8.018662683283438208E-16, 5.975035461963189015E-16, 1.000000000000000000 ) ) ;
#3481=LINE ( 'NONE', #3407, #2393 ) ;
#3485=CARTESIAN_POINT ( 'NONE',  ( -18.15085299098534577, -14.64962258016358199, 56.75231026484397745 ) ) ;
#3487=ORIENTED_EDGE ( 'NONE', *, *, #6004, .F. ) ;
#3488=VECTOR ( 'NONE', #3171, 1000.000000000000000 ) ;
#3490=VERTEX_POINT ( 'NONE', #1577 ) ;
#3491=VECTOR ( 'NONE', #12558, 999.9999999999998863 ) ;
#3492=CARTESIAN_POINT ( 'NONE',  ( -20.59651154950486784, -18.41489981358536809, 56.85231026484398598 ) ) ;
#3496=AXIS2_PLACEMENT_3D ( 'NONE', #10402, #15068, #5876 ) ;
#3498=CARTESIAN_POINT ( 'NONE',  ( -21.79367780933653265, -21.24601366423100401, 54.00231026484399166 ) ) ;
#3499=ORIENTED_EDGE ( 'NONE', *, *, #5632, .F. ) ;
#3500=VECTOR ( 'NONE', #2728, 1000.000000000000114 ) ;
#3504=LINE ( 'NONE', #4655, #3892 ) ;
#3505=EDGE_LOOP ( 'NONE', ( #426, #15038 ) ) ;
#3506=CARTESIAN_POINT ( 'NONE',  ( -15.45180655762527699, -13.52173975529984418, 56.85231026484398598 ) ) ;
#3507=ORIENTED_EDGE ( 'NONE', *, *, #9532, .T. ) ;
#3508=CARTESIAN_POINT ( 'NONE',  ( -7.887638505697304403, -19.95386229157006497, 54.00231026484400587 ) ) ;
#3511=FACE_OUTER_BOUND ( 'NONE', #3410, .T. ) ;
#3514=AXIS2_PLACEMENT_3D ( 'NONE', #8054, #12826, #9131 ) ;
#3515=EDGE_CURVE ( 'NONE', #7319, #6946, #8643, .T. ) ;
#3516=CARTESIAN_POINT ( 'NONE',  ( -9.425865349984700714, -18.82901260770113794, 56.85231026484400019 ) ) ;
#3518=DIRECTION ( 'NONE',  ( -0.8415927028326188886, 0.5401126942952620968, -9.975640502598240034E-16 ) ) ;
#3520=DIRECTION ( 'NONE',  ( -0.9731439732146150989, -0.2301973227387161258, -6.427876096865397836E-16 ) ) ;
#3522=DIRECTION ( 'NONE',  ( -8.018662683283438208E-16, 5.975035461963189015E-16, 1.000000000000000000 ) ) ;
#3525=ORIENTED_EDGE ( 'NONE', *, *, #593, .T. ) ;
#3527=DIRECTION ( 'NONE',  ( -0.9040177279761056894, -0.4274949678123940444, -4.694715627858810513E-16 ) ) ;
#3535=DIRECTION ( 'NONE',  ( -0.8934395198752397294, 0.4491835085186243748, -9.848077530122081084E-16 ) ) ;
#3538=CARTESIAN_POINT ( 'NONE',  ( -15.49969986081086226, -13.50737899243826767, -13.99768973515600301 ) ) ;
#3539=EDGE_CURVE ( 'NONE', #9881, #10505, #2983, .T. ) ;
#3545=ORIENTED_EDGE ( 'NONE', *, *, #9387, .F. ) ;
#3547=DIRECTION ( 'NONE',  ( -8.018662683283439195E-16, 5.975035461963190001E-16, 1.000000000000000000 ) ) ;
#3548=ORIENTED_EDGE ( 'NONE', *, *, #12653, .T. ) ;
#3550=ADVANCED_FACE ( 'NONE', ( #321 ), #6109, .F. ) ;
#3553=ADVANCED_FACE ( 'NONE', ( #11013 ), #400, .F. ) ;
#3554=ADVANCED_FACE ( 'NONE', ( #614 ), #5059, .T. ) ;
#3556=CARTESIAN_POINT ( 'NONE',  ( -5.628190034013325516, -14.94052892857136250, 57.00231026484399166 ) ) ;
#3558=ORIENTED_EDGE ( 'NONE', *, *, #9996, .F. ) ;
#3559=DIRECTION ( 'NONE',  ( 0.1165201156931293391, 0.9931883319083343320, -4.999999999999998416E-16 ) ) ;
#3560=DIRECTION ( 'NONE',  ( -0.8160499452489514693, -0.5779813897169900905, -3.090169943749478258E-16 ) ) ;
#3562=EDGE_LOOP ( 'NONE', ( #6332, #6855, #7002, #1600 ) ) ;
#3564=LINE ( 'NONE', #6144, #11293 ) ;
#3569=FACE_OUTER_BOUND ( 'NONE', #11700, .T. ) ;
#3571=EDGE_CURVE ( 'NONE', #7124, #186, #7257, .T. ) ;
#3573=DIRECTION ( 'NONE',  ( 0.9085715390340232123, -0.4177292884839972631, 9.781476007338056784E-16 ) ) ;
#3574=ORIENTED_EDGE ( 'NONE', *, *, #3607, .T. ) ;
#3575=DIRECTION ( 'NONE',  ( 8.018662683283438208E-16, -5.975035461963189015E-16, -1.000000000000000000 ) ) ;
#3578=ORIENTED_EDGE ( 'NONE', *, *, #3451, .T. ) ;
#3579=CARTESIAN_POINT ( 'NONE',  ( -15.49969986081092088, -13.50737899243822504, 57.00231026484397745 ) ) ;
#3580=EDGE_LOOP ( 'NONE', ( #7576, #346, #4068, #6028 ) ) ;
#3581=CARTESIAN_POINT ( 'NONE',  ( -22.70913108387521007, -17.14542124616560770, 56.85231026484398598 ) ) ;
#3583=LINE ( 'NONE', #6859, #11295 ) ;
#3586=ADVANCED_FACE ( 'NONE', ( #14609 ), #10795, .T. ) ;
#3587=DIRECTION ( 'NONE',  ( 0.7032868978765922652, 0.7109061395677488404, 1.391731009600549485E-16 ) ) ;
#3590=DIRECTION ( 'NONE',  ( -8.018662683283438208E-16, 5.975035461963189015E-16, 1.000000000000000000 ) ) ;
#3591=CARTESIAN_POINT ( 'NONE',  ( -24.80452494096261873, -9.912819877918101596, 57.00231026484397745 ) ) ;
#3592=LINE ( 'NONE', #5802, #3947 ) ;
#3593=CIRCLE ( 'NONE', #12929, 9.974999999999999645 ) ;
#3595=CARTESIAN_POINT ( 'NONE',  ( -11.68798435751175369, -21.74340199640734994, 56.85231026484400019 ) ) ;
#3600=CARTESIAN_POINT ( 'NONE',  ( -23.42445533997705454, -9.084766574938008432, 56.85231026484398598 ) ) ;
#3601=ORIENTED_EDGE ( 'NONE', *, *, #8217, .T. ) ;
#3602=VERTEX_POINT ( 'NONE', #3982 ) ;
#3604=ORIENTED_EDGE ( 'NONE', *, *, #1207, .F. ) ;
#3605=AXIS2_PLACEMENT_3D ( 'NONE', #7315, #10849, #1586 ) ;
#3606=CARTESIAN_POINT ( 'NONE',  ( -12.84854673063649599, -12.36513540471286809, 51.00231026484399166 ) ) ;
#3607=EDGE_CURVE ( 'NONE', #8564, #150, #3827, .T. ) ;
#3609=CARTESIAN_POINT ( 'NONE',  ( -24.05607732349520234, -14.07716379046991584, 56.85231026484398598 ) ) ;
#3611=CIRCLE ( 'NONE', #11429, 9.974999999999999645 ) ;
#3615=CARTESIAN_POINT ( 'NONE',  ( -21.12809094326923187, -9.219901432974651811, 57.00231026484397745 ) ) ;
#3616=DIRECTION ( 'NONE',  ( -8.018662683283439195E-16, 5.975035461963190001E-16, 1.000000000000000000 ) ) ;
#3618=ORIENTED_EDGE ( 'NONE', *, *, #4318, .F. ) ;
#3619=VERTEX_POINT ( 'NONE', #13178 ) ;
#3623=CARTESIAN_POINT ( 'NONE',  ( -21.45979773411919922, -21.50599501901345789, 48.00231026484398456 ) ) ;
#3624=EDGE_CURVE ( 'NONE', #10753, #6962, #14537, .T. ) ;
#3627=CARTESIAN_POINT ( 'NONE',  ( -15.49969986081092088, -13.50737899243822504, 56.85231026484398598 ) ) ;
#3628=DIRECTION ( 'NONE',  ( 0.8160499452489514693, 0.5779813897169900905, 3.090169943749478258E-16 ) ) ;
#3630=AXIS2_PLACEMENT_3D ( 'NONE', #14209, #3730, #8387 ) ;
#3631=CARTESIAN_POINT ( 'NONE',  ( -14.51048789653087390, -15.80334495249191207, 51.00231026484399166 ) ) ;
#3634=VECTOR ( 'NONE', #2338, 1000.000000000000114 ) ;
#3635=ORIENTED_EDGE ( 'NONE', *, *, #13383, .T. ) ;
#3639=ORIENTED_EDGE ( 'NONE', *, *, #14282, .T. ) ;
#3641=DIRECTION ( 'NONE',  ( -8.018662683283438208E-16, 5.975035461963189015E-16, 1.000000000000000000 ) ) ;
#3643=AXIS2_PLACEMENT_3D ( 'NONE', #2437, #4733, #2508 ) ;
#3644=FACE_OUTER_BOUND ( 'NONE', #7884, .T. ) ;
#3646=EDGE_CURVE ( 'NONE', #3877, #10177, #3909, .T. ) ;
#3647=EDGE_CURVE ( 'NONE', #6457, #1855, #2760, .T. ) ;
#3652=EDGE_CURVE ( 'NONE', #8561, #1003, #10946, .T. ) ;
#3654=DIRECTION ( 'NONE',  ( 8.018662683283438208E-16, -5.975035461963189015E-16, -1.000000000000000000 ) ) ;
#3655=FACE_OUTER_BOUND ( 'NONE', #13669, .T. ) ;
#3656=ORIENTED_EDGE ( 'NONE', *, *, #9346, .T. ) ;
#3657=LINE ( 'NONE', #10769, #11907 ) ;
#3659=ORIENTED_EDGE ( 'NONE', *, *, #12067, .T. ) ;
#3660=PLANE ( 'NONE',  #3643 ) ;
#3661=EDGE_LOOP ( 'NONE', ( #2550, #2751, #8218, #1733 ) ) ;
#3663=VERTEX_POINT ( 'NONE', #13543 ) ;
#3668=VECTOR ( 'NONE', #7454, 1000.000000000000114 ) ;
#3669=DIRECTION ( 'NONE',  ( 0.5975035461963188466, 0.8018662683283437342, 0.000000000000000000 ) ) ;
#3677=ORIENTED_EDGE ( 'NONE', *, *, #638, .F. ) ;
#3679=VERTEX_POINT ( 'NONE', #3052 ) ;
#3680=LINE ( 'NONE', #14387, #10333 ) ;
#3681=ORIENTED_EDGE ( 'NONE', *, *, #3300, .F. ) ;
#3683=AXIS2_PLACEMENT_3D ( 'NONE', #6114, #8189, #12958 ) ;
#3684=DIRECTION ( 'NONE',  ( 0.5975035461963189576, 0.8018662683283437342, 0.000000000000000000 ) ) ;
#3685=ORIENTED_EDGE ( 'NONE', *, *, #10585, .F. ) ;
#3686=CARTESIAN_POINT ( 'NONE',  ( -8.972439834930606040, -10.77678811232731348, 56.85231026484400019 ) ) ;
#3689=CARTESIAN_POINT ( 'NONE',  ( -7.528759897616733809, -14.80173833325270571, 57.00231026484399166 ) ) ;
#3690=EDGE_CURVE ( 'NONE', #13117, #7160, #1985, .T. ) ;
#3692=CYLINDRICAL_SURFACE ( 'NONE', #6398, 0.2500000000000004441 ) ;
#3697=ORIENTED_EDGE ( 'NONE', *, *, #14916, .T. ) ;
#3698=LINE ( 'NONE', #2551, #6621 ) ;
#3699=EDGE_LOOP ( 'NONE', ( #52, #1076, #2530, #11521 ) ) ;
#3700=DIRECTION ( 'NONE',  ( -0.8018662683283436232, 0.5975035461963189576, -9.999999999999996833E-16 ) ) ;
#3701=CIRCLE ( 'NONE', #286, 9.974999999999999645 ) ;
#3702=CARTESIAN_POINT ( 'NONE',  ( -7.064541492512761423, -18.83173137575486322, 57.00231026484399166 ) ) ;
#3705=AXIS2_PLACEMENT_3D ( 'NONE', #7577, #625, #14621 ) ;
#3706=CARTESIAN_POINT ( 'NONE',  ( -15.39025577592761174, -21.58198560776530783, 56.85231026484400019 ) ) ;
#3707=EDGE_CURVE ( 'NONE', #11022, #2020, #12317, .T. ) ;
#3708=CARTESIAN_POINT ( 'NONE',  ( -21.48581293389290892, -5.528213918555016981, 54.00231026484397745 ) ) ;
#3710=ORIENTED_EDGE ( 'NONE', *, *, #11703, .F. ) ;
#3711=CYLINDRICAL_SURFACE ( 'NONE', #7511, 0.2500000000000004441 ) ;
#3714=VERTEX_POINT ( 'NONE', #2138 ) ;
#3716=LINE ( 'NONE', #11741, #9090 ) ;
#3717=ORIENTED_EDGE ( 'NONE', *, *, #11375, .T. ) ;
#3719=VECTOR ( 'NONE', #877, 1000.000000000000114 ) ;
#3720=AXIS2_PLACEMENT_3D ( 'NONE', #7584, #6206, #6283 ) ;
#3723=FACE_OUTER_BOUND ( 'NONE', #1749, .T. ) ;
#3725=ADVANCED_FACE ( 'NONE', ( #1913 ), #6708, .F. ) ;
#3726=DIRECTION ( 'NONE',  ( 0.9826409426582665141, -0.1855175943453169496, 8.987940462991673516E-16 ) ) ;
#3727=ORIENTED_EDGE ( 'NONE', *, *, #11931, .F. ) ;
#3729=VECTOR ( 'NONE', #1834, 1000.000000000000114 ) ;
#3730=DIRECTION ( 'NONE',  ( 0.4177292884839972631, 0.9085715390340232123, -2.079116908177589032E-16 ) ) ;
#3732=VECTOR ( 'NONE', #9879, 999.9999999999998863 ) ;
#3740=EDGE_CURVE ( 'NONE', #14164, #7674, #13744, .T. ) ;
#3744=LINE ( 'NONE', #1370, #4076 ) ;
#3746=EDGE_CURVE ( 'NONE', #10582, #14123, #308, .T. ) ;
#3747=ORIENTED_EDGE ( 'NONE', *, *, #10894, .F. ) ;
#3750=CARTESIAN_POINT ( 'NONE',  ( -15.49969986081092088, -13.50737899243822504, 57.00231026484397745 ) ) ;
#3753=CARTESIAN_POINT ( 'NONE',  ( -15.49969986081092088, -13.50737899243822504, 57.00231026484397745 ) ) ;
#3756=ORIENTED_EDGE ( 'NONE', *, *, #4019, .T. ) ;
#3757=ORIENTED_EDGE ( 'NONE', *, *, #9847, .T. ) ;
#3759=DIRECTION ( 'NONE',  ( -8.018662683283438208E-16, 5.975035461963189015E-16, 1.000000000000000000 ) ) ;
#3761=EDGE_LOOP ( 'NONE', ( #12177, #5435, #167, #13592 ) ) ;
#3764=PLANE ( 'NONE',  #751 ) ;
#3765=CARTESIAN_POINT ( 'NONE',  ( -11.58094331127308507, -5.879823872646938732, 56.85231026484398598 ) ) ;
#3766=AXIS2_PLACEMENT_3D ( 'NONE', #11641, #2468, #5822 ) ;
#3767=ADVANCED_FACE ( 'NONE', ( #843 ), #10081, .F. ) ;
#3768=DIRECTION ( 'NONE',  ( 0.9354976265738682573, -0.3533329742249642913, 9.612616959383187437E-16 ) ) ;
#3769=CARTESIAN_POINT ( 'NONE',  ( -23.49646891012291050, -9.216349422280851300, 56.85231026484398598 ) ) ;
#3770=ORIENTED_EDGE ( 'NONE', *, *, #9725, .F. ) ;
#3771=DIRECTION ( 'NONE',  ( 8.018662683283438208E-16, -5.975035461963189015E-16, -1.000000000000000000 ) ) ;
#3773=CIRCLE ( 'NONE', #5716, 9.974999999999999645 ) ;
#3775=ORIENTED_EDGE ( 'NONE', *, *, #4019, .F. ) ;
#3776=LINE ( 'NONE', #10657, #8088 ) ;
#3777=EDGE_LOOP ( 'NONE', ( #14658, #12854, #13022, #1711 ) ) ;
#3778=FACE_OUTER_BOUND ( 'NONE', #14022, .T. ) ;
#3780=VECTOR ( 'NONE', #6923, 1000.000000000000000 ) ;
#3781=EDGE_CURVE ( 'NONE', #14193, #11181, #5498, .T. ) ;
#3783=DIRECTION ( 'NONE',  ( 8.018662683283438208E-16, -5.975035461963189015E-16, -1.000000000000000000 ) ) ;
#3788=DIRECTION ( 'NONE',  ( -0.9957106782009863544, -0.09252159378508259535, -7.431448254773871651E-16 ) ) ;
#3793=CARTESIAN_POINT ( 'NONE',  ( -19.68577560955674954, -20.41303028871448788, 56.85231026484398598 ) ) ;
#3797=DIRECTION ( 'NONE',  ( -8.018662683283438208E-16, 5.975035461963189015E-16, 1.000000000000000000 ) ) ;
#3800=FACE_OUTER_BOUND ( 'NONE', #13614, .T. ) ;
#3801=ORIENTED_EDGE ( 'NONE', *, *, #13922, .F. ) ;
#3802=CARTESIAN_POINT ( 'NONE',  ( -9.539601987502637215, -5.508762965862999295, 54.00231026484399166 ) ) ;
#3804=ORIENTED_EDGE ( 'NONE', *, *, #1571, .F. ) ;
#3806=ORIENTED_EDGE ( 'NONE', *, *, #7802, .T. ) ;
#3808=DIRECTION ( 'NONE',  ( -8.018662683283438208E-16, 5.975035461963189015E-16, 1.000000000000000000 ) ) ;
#3809=ORIENTED_EDGE ( 'NONE', *, *, #4279, .T. ) ;
#3812=EDGE_CURVE ( 'NONE', #12430, #2788, #10155, .T. ) ;
#3814=EDGE_CURVE ( 'NONE', #14904, #4847, #5645, .T. ) ;
#3817=ORIENTED_EDGE ( 'NONE', *, *, #3515, .F. ) ;
#3818=DIRECTION ( 'NONE',  ( -0.8415927028326188886, 0.5401126942952620968, -9.975640502598240034E-16 ) ) ;
#3821=ORIENTED_EDGE ( 'NONE', *, *, #11967, .F. ) ;
#3822=DIRECTION ( 'NONE',  ( 0.5975035461963189576, 0.8018662683283437342, 0.000000000000000000 ) ) ;
#3823=ORIENTED_EDGE ( 'NONE', *, *, #5707, .F. ) ;
#3824=DIRECTION ( 'NONE',  ( 8.018662683283438208E-16, -5.975035461963189015E-16, -1.000000000000000000 ) ) ;
#3826=ORIENTED_EDGE ( 'NONE', *, *, #6229, .T. ) ;
#3827=LINE ( 'NONE', #10874, #8606 ) ;
#3828=VECTOR ( 'NONE', #7640, 1000.000000000000114 ) ;
#3830=EDGE_CURVE ( 'NONE', #4342, #7312, #8837, .T. ) ;
#3832=DIRECTION ( 'NONE',  ( -0.9645173894937585368, -0.2640193276336892936, -6.156614753256587028E-16 ) ) ;
#3839=DIRECTION ( 'NONE',  ( -0.2640193276336892936, 0.9645173894937585368, -7.880107536067216805E-16 ) ) ;
#3840=DIRECTION ( 'NONE',  ( -8.018662683283438208E-16, 5.975035461963189015E-16, 1.000000000000000000 ) ) ;
#3843=EDGE_LOOP ( 'NONE', ( #498, #11722, #5179, #7153 ) ) ;
#3844=EDGE_LOOP ( 'NONE', ( #1152, #14832, #113, #867 ) ) ;
#3847=ORIENTED_EDGE ( 'NONE', *, *, #4215, .F. ) ;
#3849=CARTESIAN_POINT ( 'NONE',  ( -21.11416342254291934, -20.63752968607602867, 56.85231026484398598 ) ) ;
#3850=ADVANCED_FACE ( 'NONE', ( #12932 ), #7003, .T. ) ;
#3851=VECTOR ( 'NONE', #13447, 1000.000000000000114 ) ;
#3853=AXIS2_PLACEMENT_3D ( 'NONE', #8031, #3148, #5514 ) ;
#3856=LINE ( 'NONE', #8518, #11274 ) ;
#3859=CARTESIAN_POINT ( 'NONE',  ( -15.16333526000374476, -10.64029123852186665, 51.10586365543726117 ) ) ;
#3861=DIRECTION ( 'NONE',  ( 0.04695496274984587576, 0.9988970074402868660, -5.591929034707467802E-16 ) ) ;
#3865=ADVANCED_FACE ( 'NONE', ( #9398 ), #2291, .F. ) ;
#3866=AXIS2_PLACEMENT_3D ( 'NONE', #4738, #10393, #15061 ) ;
#3868=LINE ( 'NONE', #14048, #13011 ) ;
#3870=VERTEX_POINT ( 'NONE', #11543 ) ;
#3871=CARTESIAN_POINT ( 'NONE',  ( -22.55857771067089246, -13.99059064457067336, 56.85231026484398598 ) ) ;
#3875=DIRECTION ( 'NONE',  ( 0.5975035461963188466, 0.8018662683283437342, 0.000000000000000000 ) ) ;
#3876=CARTESIAN_POINT ( 'NONE',  ( -19.27841348868324189, -22.73895244004356897, 54.00231026484399166 ) ) ;
#3877=VERTEX_POINT ( 'NONE', #9164 ) ;
#3878=LINE ( 'NONE', #1357, #3358 ) ;
#3887=DIRECTION ( 'NONE',  ( 0.9755678736739574752, -0.2196982563774083075, 9.135454576426028331E-16 ) ) ;
#3888=ORIENTED_EDGE ( 'NONE', *, *, #12738, .F. ) ;
#3889=DIRECTION ( 'NONE',  ( 0.5975035461963189576, 0.8018662683283437342, 0.000000000000000000 ) ) ;
#3892=VECTOR ( 'NONE', #12331, 1000.000000000000227 ) ;
#3896=DIRECTION ( 'NONE',  ( -8.018662683283438208E-16, 5.975035461963189015E-16, 1.000000000000000000 ) ) ;
#3897=ORIENTED_EDGE ( 'NONE', *, *, #14678, .F. ) ;
#3902=DIRECTION ( 'NONE',  ( 0.3857661296576155308, 0.9225966037272105291, -2.419218955996680478E-16 ) ) ;
#3903=ORIENTED_EDGE ( 'NONE', *, *, #2454, .T. ) ;
#3904=LINE ( 'NONE', #6105, #11070 ) ;
#3905=ORIENTED_EDGE ( 'NONE', *, *, #11548, .F. ) ;
#3906=EDGE_LOOP ( 'NONE', ( #3806, #1964, #14003, #1744 ) ) ;
#3909=LINE ( 'NONE', #13397, #11788 ) ;
#3911=DIRECTION ( 'NONE',  ( 0.9805849309054467389, 0.1960948578651675878, 6.691306063588567679E-16 ) ) ;
#3912=CARTESIAN_POINT ( 'NONE',  ( -12.46042140754850180, -23.00808483377099734, 56.85231026484400019 ) ) ;
#3914=CARTESIAN_POINT ( 'NONE',  ( -16.84408283975263032, -15.31157809617700316, 51.25231026484399166 ) ) ;
#3916=EDGE_CURVE ( 'NONE', #15033, #4751, #1063, .T. ) ;
#3917=LINE ( 'NONE', #13188, #57 ) ;
#3918=CIRCLE ( 'NONE', #14176, 9.974999999999999645 ) ;
#3919=ORIENTED_EDGE ( 'NONE', *, *, #3069, .T. ) ;
#3920=DIRECTION ( 'NONE',  ( -0.9578660637129379207, 0.2872152572324145892, -9.396926207859088029E-16 ) ) ;
#3921=DIRECTION ( 'NONE',  ( -8.018662683283438208E-16, 5.975035461963189015E-16, 1.000000000000000000 ) ) ;
#3923=ORIENTED_EDGE ( 'NONE', *, *, #6157, .T. ) ;
#3924=ADVANCED_FACE ( 'NONE', ( #13840, #1212 ), #3356, .F. ) ;
#3925=FACE_OUTER_BOUND ( 'NONE', #5332, .T. ) ;
#3926=ORIENTED_EDGE ( 'NONE', *, *, #7753, .F. ) ;
#3927=CARTESIAN_POINT ( 'NONE',  ( -16.38999062866295020, -11.44100962838991364, 51.25231026484399166 ) ) ;
#3928=EDGE_CURVE ( 'NONE', #1378, #9153, #11761, .T. ) ;
#3932=FACE_OUTER_BOUND ( 'NONE', #2919, .T. ) ;
#3933=CARTESIAN_POINT ( 'NONE',  ( -14.99866629829804765, -4.445910272123860807, 56.85231026484398598 ) ) ;
#3938=EDGE_CURVE ( 'NONE', #9118, #14007, #5864, .T. ) ;
#3941=VERTEX_POINT ( 'NONE', #8166 ) ;
#3942=ORIENTED_EDGE ( 'NONE', *, *, #11284, .T. ) ;
#3943=CARTESIAN_POINT ( 'NONE',  ( -12.23206416678372577, -4.082773856353239417, 54.00231026484399166 ) ) ;
#3944=DIRECTION ( 'NONE',  ( 0.4587843131450244361, -0.8885476655824651182, 8.987940462991667599E-16 ) ) ;
#3945=ORIENTED_EDGE ( 'NONE', *, *, #8691, .T. ) ;
#3946=LINE ( 'NONE', #1878, #5609 ) ;
#3947=VECTOR ( 'NONE', #10108, 1000.000000000000000 ) ;
#3948=DIRECTION ( 'NONE',  ( 0.5975035461963189576, 0.8018662683283437342, 0.000000000000000000 ) ) ;
#3949=DIRECTION ( 'NONE',  ( -8.018662683283438208E-16, 5.975035461963189015E-16, 1.000000000000000000 ) ) ;
#3953=LINE ( 'NONE', #217, #10181 ) ;
#3957=LINE ( 'NONE', #2811, #5907 ) ;
#3959=EDGE_LOOP ( 'NONE', ( #7599, #12679, #9463, #10080 ) ) ;
#3960=CARTESIAN_POINT ( 'NONE',  ( -15.49969986081092088, -13.50737899243822504, 57.00231026484397745 ) ) ;
#3968=VECTOR ( 'NONE', #2194, 1000.000000000000114 ) ;
#3969=VECTOR ( 'NONE', #14833, 1000.000000000000114 ) ;
#3971=VECTOR ( 'NONE', #3587, 1000.000000000000000 ) ;
#3973=LINE ( 'NONE', #14380, #7903 ) ;
#3975=CARTESIAN_POINT ( 'NONE',  ( -19.51793069539949599, -6.502732608789604463, 56.85231026484398598 ) ) ;
#3977=ORIENTED_EDGE ( 'NONE', *, *, #8963, .T. ) ;
#3978=ORIENTED_EDGE ( 'NONE', *, *, #12529, .T. ) ;
#3982=CARTESIAN_POINT ( 'NONE',  ( -7.829332545557824652, -7.130382030772257629, 57.00231026484399166 ) ) ;
#3984=VECTOR ( 'NONE', #7527, 1000.000000000000000 ) ;
#3985=CARTESIAN_POINT ( 'NONE',  ( -18.18846581869434686, -17.11577719991577595, 46.00231026484398456 ) ) ;
#3986=EDGE_CURVE ( 'NONE', #3051, #6590, #3583, .T. ) ;
#3988=LINE ( 'NONE', #5136, #15098 ) ;
#3989=VECTOR ( 'NONE', #11257, 1000.000000000000000 ) ;
#3993=VECTOR ( 'NONE', #5767, 1000.000000000000000 ) ;
#3994=ORIENTED_EDGE ( 'NONE', *, *, #6485, .T. ) ;
#3997=ORIENTED_EDGE ( 'NONE', *, *, #2655, .F. ) ;
#4003=EDGE_CURVE ( 'NONE', #612, #3870, #5794, .T. ) ;
#4008=AXIS2_PLACEMENT_3D ( 'NONE', #10969, #9308, #13984 ) ;
#4009=PLANE ( 'NONE',  #5875 ) ;
#4011=ORIENTED_EDGE ( 'NONE', *, *, #1754, .T. ) ;
#4017=DIRECTION ( 'NONE',  ( 8.018662683283438208E-16, -5.975035461963189015E-16, -1.000000000000000000 ) ) ;
#4018=ORIENTED_EDGE ( 'NONE', *, *, #6592, .T. ) ;
#4019=EDGE_CURVE ( 'NONE', #11184, #9234, #10043, .T. ) ;
#4021=( BOUNDED_CURVE ( )  B_SPLINE_CURVE ( 3, ( #11464, #12695, #2061, #839 ),
 .UNSPECIFIED., .F., .T. ) 
 B_SPLINE_CURVE_WITH_KNOTS ( ( 4, 4 ),
 ( 4.712388980384689674, 6.283185307179586232 ),
 .UNSPECIFIED. ) 
 CURVE ( )  GEOMETRIC_REPRESENTATION_ITEM ( )  RATIONAL_B_SPLINE_CURVE ( ( 1.000000000000000000, 0.8047378541243649375, 0.8047378541243649375, 1.000000000000000000 ) ) 
 REPRESENTATION_ITEM ( '' )  );
#4025=DIRECTION ( 'NONE',  ( 8.018662683283438208E-16, -5.975035461963189015E-16, -1.000000000000000000 ) ) ;
#4026=ADVANCED_FACE ( 'NONE', ( #225 ), #4091, .T. ) ;
#4027=VECTOR ( 'NONE', #10245, 1000.000000000000114 ) ;
#4031=ORIENTED_EDGE ( 'NONE', *, *, #1250, .F. ) ;
#4037=ORIENTED_EDGE ( 'NONE', *, *, #2961, .T. ) ;
#4039=ORIENTED_EDGE ( 'NONE', *, *, #8298, .F. ) ;
#4044=LINE ( 'NONE', #1594, #3092 ) ;
#4046=CARTESIAN_POINT ( 'NONE',  ( -15.19545581216392627, -5.437764035151672282, 56.85231026484398598 ) ) ;
#4049=DIRECTION ( 'NONE',  ( 0.5975035461963189576, 0.8018662683283437342, 0.000000000000000000 ) ) ;
#4050=ORIENTED_EDGE ( 'NONE', *, *, #5771, .F. ) ;
#4052=ORIENTED_EDGE ( 'NONE', *, *, #14799, .F. ) ;
#4054=EDGE_CURVE ( 'NONE', #12536, #13190, #13505, .T. ) ;
#4055=CARTESIAN_POINT ( 'NONE',  ( -11.68798435751175369, -21.74340199640734994, 57.00231026484399166 ) ) ;
#4056=CARTESIAN_POINT ( 'NONE',  ( -16.17213342976032209, -5.460076146431361188, 57.00231026484397745 ) ) ;
#4058=CARTESIAN_POINT ( 'NONE',  ( -11.55178736972959896, -19.37894070656198764, 56.85231026484400019 ) ) ;
#4059=LINE ( 'NONE', #8494, #2327 ) ;
#4060=AXIS2_PLACEMENT_3D ( 'NONE', #9226, #7068, #11528 ) ;
#4061=CARTESIAN_POINT ( 'NONE',  ( -12.37415300023346809, -4.034703455804747207, 56.85231026484398598 ) ) ;
#4062=CYLINDRICAL_SURFACE ( 'NONE', #3131, 0.2500000000000007216 ) ;
#4063=LINE ( 'NONE', #11253, #1049 ) ;
#4068=ORIENTED_EDGE ( 'NONE', *, *, #14054, .F. ) ;
#4069=ORIENTED_EDGE ( 'NONE', *, *, #1842, .F. ) ;
#4074=CARTESIAN_POINT ( 'NONE',  ( -15.53608329785963527, -13.54167542823733328, 56.85231026484398598 ) ) ;
#4076=VECTOR ( 'NONE', #9552, 999.9999999999998863 ) ;
#4082=VECTOR ( 'NONE', #2504, 1000.000000000000000 ) ;
#4085=ORIENTED_EDGE ( 'NONE', *, *, #1521, .F. ) ;
#4089=VERTEX_POINT ( 'NONE', #2945 ) ;
#4091=CYLINDRICAL_SURFACE ( 'NONE', #5672, 0.2499999999999997502 ) ;
#4092=EDGE_CURVE ( 'NONE', #1165, #1325, #3017, .T. ) ;
#4093=LINE ( 'NONE', #5317, #13321 ) ;
#4097=CIRCLE ( 'NONE', #9957, 9.974999999999999645 ) ;
#4098=VECTOR ( 'NONE', #8214, 1000.000000000000114 ) ;
#4100=CARTESIAN_POINT ( 'NONE',  ( -23.55378106252664239, -12.92169478045303066, 56.85231026484398598 ) ) ;
#4101=AXIS2_PLACEMENT_3D ( 'NONE', #10025, #14855, #6724 ) ;
#4102=VERTEX_POINT ( 'NONE', #12357 ) ;
#4104=CARTESIAN_POINT ( 'NONE',  ( -15.47724068538499154, -13.46270701644446177, 56.85231026484398598 ) ) ;
#4105=ORIENTED_EDGE ( 'NONE', *, *, #3781, .F. ) ;
#4106=EDGE_CURVE ( 'NONE', #6628, #5981, #6519, .T. ) ;
#4107=DIRECTION ( 'NONE',  ( -8.018662683283438208E-16, 5.975035461963189015E-16, 1.000000000000000000 ) ) ;
#4111=ORIENTED_EDGE ( 'NONE', *, *, #10681, .T. ) ;
#4113=EDGE_CURVE ( 'NONE', #7645, #1909, #6591, .T. ) ;
#4114=VECTOR ( 'NONE', #4746, 1000.000000000000114 ) ;
#4115=VECTOR ( 'NONE', #4660, 1000.000000000000000 ) ;
#4116=CARTESIAN_POINT ( 'NONE',  ( -12.66248504435161948, -4.886969368454929352, 56.85231026484398598 ) ) ;
#4117=EDGE_CURVE ( 'NONE', #13725, #4633, #6371, .T. ) ;
#4118=DIRECTION ( 'NONE',  ( 0.9755678736739583634, -0.2196982563774038943, 9.135454576426008610E-16 ) ) ;
#4122=EDGE_LOOP ( 'NONE', ( #3525, #8413, #800, #62 ) ) ;
#4127=LINE ( 'NONE', #8639, #14252 ) ;
#4129=ORIENTED_EDGE ( 'NONE', *, *, #7549, .F. ) ;
#4137=LINE ( 'NONE', #621, #11676 ) ;
#4138=EDGE_CURVE ( 'NONE', #3941, #6584, #9280, .T. ) ;
#4139=CARTESIAN_POINT ( 'NONE',  ( -13.11366204365393706, -12.47935976348540876, 51.00231026484399166 ) ) ;
#4141=AXIS2_PLACEMENT_3D ( 'NONE', #4952, #9533, #14201 ) ;
#4142=FACE_OUTER_BOUND ( 'NONE', #10254, .T. ) ;
#4145=ORIENTED_EDGE ( 'NONE', *, *, #5599, .F. ) ;
#4146=CARTESIAN_POINT ( 'NONE',  ( -6.726903101582546007, -11.18374239837452500, 56.85231026484400019 ) ) ;
#4151=CARTESIAN_POINT ( 'NONE',  ( -15.49969986081092088, -13.50737899243822504, 57.00231026484397745 ) ) ;
#4152=ORIENTED_EDGE ( 'NONE', *, *, #14745, .F. ) ;
#4154=AXIS2_PLACEMENT_3D ( 'NONE', #2106, #6830, #9283 ) ;
#4155=PLANE ( 'NONE',  #5855 ) ;
#4156=DIRECTION ( 'NONE',  ( 0.8018662683283436232, -0.5975035461963189576, 9.999999999999998805E-16 ) ) ;
#4157=EDGE_CURVE ( 'NONE', #4294, #9099, #805, .T. ) ;
#4158=ADVANCED_FACE ( 'NONE', ( #5460 ), #3471, .F. ) ;
#4159=AXIS2_PLACEMENT_3D ( 'NONE', #13806, #11505, #1029 ) ;
#4160=CARTESIAN_POINT ( 'NONE',  ( -12.60362876103445018, -23.05271278361805543, 54.00231026484399166 ) ) ;
#4162=ORIENTED_EDGE ( 'NONE', *, *, #8914, .T. ) ;
#4163=CARTESIAN_POINT ( 'NONE',  ( -11.16775676328318845, -22.49263881059495063, 54.00231026484399166 ) ) ;
#4164=DIRECTION ( 'NONE',  ( -0.5975035461963172922, -0.8018662683283449555, 0.000000000000000000 ) ) ;
#4165=ORIENTED_EDGE ( 'NONE', *, *, #2331, .F. ) ;
#4166=ORIENTED_EDGE ( 'NONE', *, *, #11514, .F. ) ;
#4167=CARTESIAN_POINT ( 'NONE',  ( -23.52886110248590867, -17.73748770914800943, 56.85231026484398598 ) ) ;
#4170=VECTOR ( 'NONE', #2539, 1000.000000000000114 ) ;
#4172=FACE_OUTER_BOUND ( 'NONE', #4379, .T. ) ;
#4175=CARTESIAN_POINT ( 'NONE',  ( -15.49969986081092088, -13.50737899243822504, 57.00231026484397745 ) ) ;
#4183=CARTESIAN_POINT ( 'NONE',  ( -23.96284084890188382, -10.23071992935364527, 57.00231026484397745 ) ) ;
#4185=CARTESIAN_POINT ( 'NONE',  ( -15.49969986081092088, -13.50737899243822504, 57.00231026484397745 ) ) ;
#4186=AXIS2_PLACEMENT_3D ( 'NONE', #10551, #2010, #8961 ) ;
#4187=DIRECTION ( 'NONE',  ( -0.4895147004624045839, 0.8719950447285823580, -9.135454576426008610E-16 ) ) ;
#4190=EDGE_CURVE ( 'NONE', #12810, #6704, #5684, .T. ) ;
#4192=FACE_OUTER_BOUND ( 'NONE', #5641, .T. ) ;
#4193=CARTESIAN_POINT ( 'NONE',  ( -14.07534335717186202, -5.558639560896826204, 56.85231026484398598 ) ) ;
#4194=EDGE_CURVE ( 'NONE', #13942, #12795, #12588, .T. ) ;
#4195=ORIENTED_EDGE ( 'NONE', *, *, #5778, .T. ) ;
#4196=CARTESIAN_POINT ( 'NONE',  ( -12.60362876103445373, -23.05271278361805543, 57.00231026484399166 ) ) ;
#4198=CARTESIAN_POINT ( 'NONE',  ( -15.49969986081091733, -13.50737899243822682, 54.00231026484399166 ) ) ;
#4199=VECTOR ( 'NONE', #10404, 1000.000000000000000 ) ;
#4200=ORIENTED_EDGE ( 'NONE', *, *, #5064, .T. ) ;
#4202=VERTEX_POINT ( 'NONE', #4399 ) ;
#4206=FACE_OUTER_BOUND ( 'NONE', #13027, .T. ) ;
#4207=AXIS2_PLACEMENT_3D ( 'NONE', #14258, #5984, #7046 ) ;
#4211=AXIS2_PLACEMENT_3D ( 'NONE', #10351, #15018, #3396 ) ;
#4214=DIRECTION ( 'NONE',  ( -0.8934395198752397294, 0.4491835085186243748, -9.848077530122081084E-16 ) ) ;
#4215=EDGE_CURVE ( 'NONE', #858, #6590, #12663, .T. ) ;
#4217=FACE_OUTER_BOUND ( 'NONE', #398, .T. ) ;
#4218=CARTESIAN_POINT ( 'NONE',  ( -16.32149003149046607, -5.473954385499126829, 56.85231026484398598 ) ) ;
#4220=CARTESIAN_POINT ( 'NONE',  ( -21.29301345516119071, -7.881655252552254964, 57.00231026484397745 ) ) ;
#4221=ORIENTED_EDGE ( 'NONE', *, *, #4113, .F. ) ;
#4225=DIRECTION ( 'NONE',  ( -8.018662683283438208E-16, 5.975035461963189015E-16, 1.000000000000000000 ) ) ;
#4229=ORIENTED_EDGE ( 'NONE', *, *, #11629, .T. ) ;
#4230=CARTESIAN_POINT ( 'NONE',  ( -15.49969986081091022, -13.50737899243823215, 46.00231026484398456 ) ) ;
#4231=DIRECTION ( 'NONE',  ( 0.8599296884906633132, -0.5104125104778985955, 9.945218953682734920E-16 ) ) ;
#4233=VECTOR ( 'NONE', #14774, 1000.000000000000227 ) ;
#4234=EDGE_CURVE ( 'NONE', #3406, #4445, #6128, .T. ) ;
#4235=FACE_OUTER_BOUND ( 'NONE', #12165, .T. ) ;
#4236=CARTESIAN_POINT ( 'NONE',  ( -15.49969986081092088, -13.50737899243822504, 57.00231026484397745 ) ) ;
#4237=ORIENTED_EDGE ( 'NONE', *, *, #788, .F. ) ;
#4238=DIRECTION ( 'NONE',  ( 8.018662683283438208E-16, -5.975035461963189015E-16, -1.000000000000000000 ) ) ;
#4239=CYLINDRICAL_SURFACE ( 'NONE', #11409, 5.000000000000000000 ) ;
#4240=ORIENTED_EDGE ( 'NONE', *, *, #4296, .F. ) ;
#4243=ORIENTED_EDGE ( 'NONE', *, *, #3986, .F. ) ;
#4249=VECTOR ( 'NONE', #8593, 1000.000000000000000 ) ;
#4252=DIRECTION ( 'NONE',  ( -0.5779813897169902015, 0.8160499452489514693, -9.510565162951533652E-16 ) ) ;
#4253=DIRECTION ( 'NONE',  ( -8.018662683283438208E-16, 5.975035461963189015E-16, 1.000000000000000000 ) ) ;
#4255=VERTEX_POINT ( 'NONE', #1332 ) ;
#4259=PLANE ( 'NONE',  #12025 ) ;
#4261=CIRCLE ( 'NONE', #12084, 5.000000000000000000 ) ;
#4264=ADVANCED_FACE ( 'NONE', ( #7204 ), #4856, .F. ) ;
#4266=PLANE ( 'NONE',  #1762 ) ;
#4268=PLANE ( 'NONE',  #2370 ) ;
#4269=CARTESIAN_POINT ( 'NONE',  ( -16.34789837066772122, -3.568506607309356315, 56.85231026484398598 ) ) ;
#4271=ORIENTED_EDGE ( 'NONE', *, *, #6544, .T. ) ;
#4275=VERTEX_POINT ( 'NONE', #11885 ) ;
#4278=ORIENTED_EDGE ( 'NONE', *, *, #193, .T. ) ;
#4279=EDGE_CURVE ( 'NONE', #7908, #4983, #1405, .T. ) ;
#4280=CARTESIAN_POINT ( 'NONE',  ( -21.11416342254291934, -20.63752968607602867, 56.85231026484398598 ) ) ;
#4282=ADVANCED_FACE ( 'NONE', ( #2629 ), #9509, .F. ) ;
#4283=DIRECTION ( 'NONE',  ( -8.018662683283438208E-16, 5.975035461963189015E-16, 1.000000000000000000 ) ) ;
#4284=CARTESIAN_POINT ( 'NONE',  ( -14.26755283655060680, -21.48817241857114269, 56.85231026484400019 ) ) ;
#4285=DIRECTION ( 'NONE',  ( 0.6061090314442014737, -0.7953815700667020705, 9.612616959383187437E-16 ) ) ;
#4290=DIRECTION ( 'NONE',  ( 0.1617534816134024167, -0.9868311969055004740, 7.193398003386505973E-16 ) ) ;
#4291=ORIENTED_EDGE ( 'NONE', *, *, #5624, .F. ) ;
#4293=CARTESIAN_POINT ( 'NONE',  ( -18.15085299098534222, -14.64962258016358554, 51.00231026484399166 ) ) ;
#4294=VERTEX_POINT ( 'NONE', #13199 ) ;
#4296=EDGE_CURVE ( 'NONE', #12810, #14910, #6965, .T. ) ;
#4298=FACE_OUTER_BOUND ( 'NONE', #12096, .T. ) ;
#4299=ADVANCED_FACE ( 'NONE', ( #8204 ), #8513, .F. ) ;
#4305=CARTESIAN_POINT ( 'NONE',  ( -18.50396719079564889, -6.011671700261853601, 56.85231026484398598 ) ) ;
#4307=DIRECTION ( 'NONE',  ( -8.018662683283438208E-16, 5.975035461963189015E-16, 1.000000000000000000 ) ) ;
#4310=ORIENTED_EDGE ( 'NONE', *, *, #3652, .F. ) ;
#4313=DIRECTION ( 'NONE',  ( -0.8415927028326188886, 0.5401126942952620968, -9.975640502598240034E-16 ) ) ;
#4315=VERTEX_POINT ( 'NONE', #3702 ) ;
#4317=EDGE_CURVE ( 'NONE', #2532, #8254, #4778, .T. ) ;
#4318=EDGE_CURVE ( 'NONE', #12566, #11022, #12047, .T. ) ;
#4319=ORIENTED_EDGE ( 'NONE', *, *, #10640, .F. ) ;
#4322=FACE_OUTER_BOUND ( 'NONE', #4674, .T. ) ;
#4324=VECTOR ( 'NONE', #7964, 1000.000000000000227 ) ;
#4325=DIRECTION ( 'NONE',  ( 0.5691548339926102429, 0.8222303661035903488, -3.489949670250048422E-17 ) ) ;
#4327=CIRCLE ( 'NONE', #6749, 9.974999999999999645 ) ;
#4328=EDGE_CURVE ( 'NONE', #4893, #6007, #14104, .T. ) ;
#4329=CARTESIAN_POINT ( 'NONE',  ( -7.528759897616733809, -14.80173833325270571, 56.85231026484400019 ) ) ;
#4335=DIRECTION ( 'NONE',  ( -8.018662683283438208E-16, 5.975035461963189015E-16, 1.000000000000000000 ) ) ;
#4337=ORIENTED_EDGE ( 'NONE', *, *, #13527, .T. ) ;
#4338=DIRECTION ( 'NONE',  ( 0.9957106782009873536, 0.09252159378507134047, 7.431448254773946593E-16 ) ) ;
#4339=DIRECTION ( 'NONE',  ( 0.5975035461963189576, 0.8018662683283437342, 0.000000000000000000 ) ) ;
#4342=VERTEX_POINT ( 'NONE', #3623 ) ;
#4344=LINE ( 'NONE', #5403, #12743 ) ;
#4346=CIRCLE ( 'NONE', #11674, 9.974999999999999645 ) ;
#4347=PRODUCT_CONTEXT ( 'NONE', #13971, 'mechanical' ) ;
#4348=FACE_OUTER_BOUND ( 'NONE', #6350, .T. ) ;
#4349=AXIS2_PLACEMENT_3D ( 'NONE', #11710, #13935, #2534 ) ;
#4351=PLANE ( 'NONE',  #9917 ) ;
#4352=CARTESIAN_POINT ( 'NONE',  ( -25.21423696146293736, -11.24278324042065869, 56.85231026484398598 ) ) ;
#4355=DIRECTION ( 'NONE',  ( -0.5975035461963188466, -0.8018662683283437342, 0.000000000000000000 ) ) ;
#4356=LINE ( 'NONE', #12540, #14756 ) ;
#4359=VERTEX_POINT ( 'NONE', #1175 ) ;
#4362=CARTESIAN_POINT ( 'NONE',  ( -8.663330333365388825, -17.80566954616001496, 56.85231026484400019 ) ) ;
#4365=CARTESIAN_POINT ( 'NONE',  ( -21.21771647519868154, -9.340181373223902739, 56.85231026484398598 ) ) ;
#4366=VECTOR ( 'NONE', #8585, 1000.000000000000000 ) ;
#4367=CARTESIAN_POINT ( 'NONE',  ( -18.36422177163696290, -5.957162821864243618, 56.85231026484398598 ) ) ;
#4368=ADVANCED_FACE ( 'NONE', ( #5832 ), #1703, .T. ) ;
#4369=CARTESIAN_POINT ( 'NONE',  ( -19.05456510292772876, -4.187316862259577555, 56.85231026484398598 ) ) ;
#4370=PLANE ( 'NONE',  #366 ) ;
#4371=CARTESIAN_POINT ( 'NONE',  ( -13.88982576282654691, -4.575998618238553917, 57.00231026484397745 ) ) ;
#4372=VERTEX_POINT ( 'NONE', #6356 ) ;
#4374=ORIENTED_EDGE ( 'NONE', *, *, #8588, .T. ) ;
#4375=DIRECTION ( 'NONE',  ( 0.9316361277244821215, 0.3633925226508276651, 5.299192642332029177E-16 ) ) ;
#4376=CARTESIAN_POINT ( 'NONE',  ( -18.15085299098534222, -14.64962258016358376, 51.25231026484399166 ) ) ;
#4378=CARTESIAN_POINT ( 'NONE',  ( -9.299228256956212135, -8.333850033420862502, 57.00231026484397745 ) ) ;
#4379=EDGE_LOOP ( 'NONE', ( #2311, #553, #4544, #14432 ) ) ;
#4380=LINE ( 'NONE', #2007, #9530 ) ;
#4381=CARTESIAN_POINT ( 'NONE',  ( 0.000000000000000000, 0.000000000000000000, 0.000000000000000000 ) ) ;
#4387=FACE_OUTER_BOUND ( 'NONE', #8436, .T. ) ;
#4389=ORIENTED_EDGE ( 'NONE', *, *, #3115, .T. ) ;
#4392=DIRECTION ( 'NONE',  ( -0.1165201156931293391, -0.9931883319083343320, 4.999999999999997430E-16 ) ) ;
#4393=ORIENTED_EDGE ( 'NONE', *, *, #8810, .F. ) ;
#4394=ORIENTED_EDGE ( 'NONE', *, *, #12628, .T. ) ;
#4395=DIRECTION ( 'NONE',  ( 0.2872152572324145892, 0.9578660637129379207, -3.420201433256678811E-16 ) ) ;
#4396=VERTEX_POINT ( 'NONE', #6286 ) ;
#4397=EDGE_CURVE ( 'NONE', #1781, #2885, #9956, .T. ) ;
#4399=CARTESIAN_POINT ( 'NONE',  ( -17.62015867087677634, -21.29935591968936137, 57.00231026484399166 ) ) ;
#4400=DIRECTION ( 'NONE',  ( -8.018662683283439195E-16, 5.975035461963190001E-16, 1.000000000000000000 ) ) ;
#4404=EDGE_CURVE ( 'NONE', #12600, #10731, #14631, .T. ) ;
#4406=PLANE ( 'NONE',  #11563 ) ;
#4408=ORIENTED_EDGE ( 'NONE', *, *, #5821, .F. ) ;
#4409=DIRECTION ( 'NONE',  ( 0.6859287159822015090, -0.7276687409742212953, 9.848077530122081084E-16 ) ) ;
#4411=ORIENTED_EDGE ( 'NONE', *, *, #5430, .T. ) ;
#4412=ORIENTED_EDGE ( 'NONE', *, *, #1632, .F. ) ;
#4414=AXIS2_PLACEMENT_3D ( 'NONE', #14482, #4231, #12190 ) ;
#4416=CARTESIAN_POINT ( 'NONE',  ( -7.734307812155741146, -7.246443652516329159, 54.00231026484399166 ) ) ;
#4418=VERTEX_POINT ( 'NONE', #13418 ) ;
#4422=EDGE_CURVE ( 'NONE', #15033, #5603, #3408, .T. ) ;
#4425=LINE ( 'NONE', #6620, #2315 ) ;
#4427=LINE ( 'NONE', #6084, #6029 ) ;
#4429=ORIENTED_EDGE ( 'NONE', *, *, #7290, .F. ) ;
#4433=CARTESIAN_POINT ( 'NONE',  ( -20.64795620320353109, -18.36032465801230273, 57.00231026484397745 ) ) ;
#4436=DIRECTION ( 'NONE',  ( -0.9731439732146149879, -0.2301973227387160703, -6.427876096865396850E-16 ) ) ;
#4439=CIRCLE ( 'NONE', #13723, 9.974999999999999645 ) ;
#4440=CARTESIAN_POINT ( 'NONE',  ( -15.83606446161809167, -16.37446674635458521, 51.25231026484399166 ) ) ;
#4442=LINE ( 'NONE', #8092, #3253 ) ;
#4443=ORIENTED_EDGE ( 'NONE', *, *, #14931, .F. ) ;
#4445=VERTEX_POINT ( 'NONE', #14481 ) ;
#4447=CARTESIAN_POINT ( 'NONE',  ( -5.524802968312267026, -13.55273297815671008, 56.85231026484400019 ) ) ;
#4448=VERTEX_POINT ( 'NONE', #12339 ) ;
#4451=ORIENTED_EDGE ( 'NONE', *, *, #4157, .T. ) ;
#4454=EDGE_CURVE ( 'NONE', #7254, #5023, #7509, .T. ) ;
#4457=AXIS2_PLACEMENT_3D ( 'NONE', #12985, #6071, #10523 ) ;
#4459=ORIENTED_EDGE ( 'NONE', *, *, #9627, .F. ) ;
#4463=ORIENTED_EDGE ( 'NONE', *, *, #12717, .T. ) ;
#4465=ORIENTED_EDGE ( 'NONE', *, *, #14166, .T. ) ;
#4466=CARTESIAN_POINT ( 'NONE',  ( -15.49969986081092088, -13.50737899243822504, 57.00231026484397745 ) ) ;
#4468=ORIENTED_EDGE ( 'NONE', *, *, #482, .F. ) ;
#4469=LINE ( 'NONE', #9124, #539 ) ;
#4470=ORIENTED_EDGE ( 'NONE', *, *, #15043, .T. ) ;
#4472=ADVANCED_FACE ( 'NONE', ( #5372 ), #710, .F. ) ;
#4473=VECTOR ( 'NONE', #13705, 1000.000000000000114 ) ;
#4474=ADVANCED_FACE ( 'NONE', ( #1558 ), #6210, .F. ) ;
#4475=DIRECTION ( 'NONE',  ( 0.5975035461963188466, 0.8018662683283437342, 0.000000000000000000 ) ) ;
#4476=LINE ( 'NONE', #4548, #12709 ) ;
#4478=CARTESIAN_POINT ( 'NONE',  ( -15.53979317422733786, -13.47750381512840967, 56.85231026484398598 ) ) ;
#4480=ORIENTED_EDGE ( 'NONE', *, *, #601, .F. ) ;
#4481=CARTESIAN_POINT ( 'NONE',  ( -9.425865349984700714, -18.82901260770113794, 57.00231026484399166 ) ) ;
#4486=CIRCLE ( 'NONE', #9115, 9.974999999999999645 ) ;
#4488=VECTOR ( 'NONE', #3560, 1000.000000000000114 ) ;
#4489=DIRECTION ( 'NONE',  ( 8.018662683283438208E-16, -5.975035461963189015E-16, -1.000000000000000000 ) ) ;
#4492=EDGE_CURVE ( 'NONE', #4102, #34, #9888, .T. ) ;
#4493=ADVANCED_FACE ( 'NONE', ( #7955 ), #5667, .T. ) ;
#4496=CARTESIAN_POINT ( 'NONE',  ( -6.468284635389320414, -17.74225372801456757, 57.00231026484399166 ) ) ;
#4497=EDGE_CURVE ( 'NONE', #13689, #15033, #15080, .T. ) ;
#4498=CARTESIAN_POINT ( 'NONE',  ( -5.898712304418586960, -10.80152183767200391, 54.00231026484399166 ) ) ;
#4499=CARTESIAN_POINT ( 'NONE',  ( -17.73437360760467030, -13.24520873212868644, 51.25231026484399166 ) ) ;
#4500=VERTEX_POINT ( 'NONE', #13790 ) ;
#4503=VECTOR ( 'NONE', #12133, 1000.000000000000000 ) ;
#4507=LINE ( 'NONE', #7780, #6189 ) ;
#4508=ORIENTED_EDGE ( 'NONE', *, *, #8527, .F. ) ;
#4509=VECTOR ( 'NONE', #14199, 1000.000000000000114 ) ;
#4510=DIRECTION ( 'NONE',  ( 0.5975035461963188466, 0.8018662683283437342, 0.000000000000000000 ) ) ;
#4511=DIRECTION ( 'NONE',  ( 0.8018662683283437342, -0.5975035461963188466, 9.999999999999996833E-16 ) ) ;
#4518=LINE ( 'NONE', #6564, #12379 ) ;
#4521=PLANE ( 'NONE',  #940 ) ;
#4524=EDGE_LOOP ( 'NONE', ( #2115, #5739, #1062, #14717 ) ) ;
#4526=ORIENTED_EDGE ( 'NONE', *, *, #12420, .F. ) ;
#4528=ORIENTED_EDGE ( 'NONE', *, *, #14088, .T. ) ;
#4530=CARTESIAN_POINT ( 'NONE',  ( -13.18491133144367922, -15.23222315862922471, 56.75231026484399166 ) ) ;
#4531=VERTEX_POINT ( 'NONE', #784 ) ;
#4534=LINE ( 'NONE', #6882, #7338 ) ;
#4543=ORIENTED_EDGE ( 'NONE', *, *, #13379, .F. ) ;
#4544=ORIENTED_EDGE ( 'NONE', *, *, #13083, .F. ) ;
#4546=VERTEX_POINT ( 'NONE', #1010 ) ;
#4547=DIRECTION ( 'NONE',  ( -0.5975035461963187355, -0.8018662683283438453, 0.000000000000000000 ) ) ;
#4548=CARTESIAN_POINT ( 'NONE',  ( -11.61446667642527331, -19.42012692406430574, 56.85231026484400019 ) ) ;
#4549=CIRCLE ( 'NONE', #3073, 9.974999999999999645 ) ;
#4550=FACE_OUTER_BOUND ( 'NONE', #12730, .T. ) ;
#4552=CARTESIAN_POINT ( 'NONE',  ( -14.11952815701478059, -21.46390939632912875, 56.85231026484400019 ) ) ;
#4556=PLANE ( 'NONE',  #12550 ) ;
#4557=ORIENTED_EDGE ( 'NONE', *, *, #13124, .T. ) ;
#4558=ORIENTED_EDGE ( 'NONE', *, *, #9314, .F. ) ;
#4562=AXIS2_PLACEMENT_3D ( 'NONE', #14151, #2518, #13923 ) ;
#4563=CARTESIAN_POINT ( 'NONE',  ( -24.03943920472178775, -16.57887731378902885, 57.00231026484397745 ) ) ;
#4565=DIRECTION ( 'NONE',  ( 8.018662683283438208E-16, -5.975035461963189015E-16, -1.000000000000000000 ) ) ;
#4566=VECTOR ( 'NONE', #15015, 1000.000000000000000 ) ;
#4567=CARTESIAN_POINT ( 'NONE',  ( -6.426265323245524463, -13.69186664111786023, 57.00231026484399166 ) ) ;
#4569=VECTOR ( 'NONE', #306, 1000.000000000000000 ) ;
#4572=DIRECTION ( 'NONE',  ( 0.7953815700667045130, 0.6061090314441981430, 2.756373558170028881E-16 ) ) ;
#4577=VECTOR ( 'NONE', #517, 1000.000000000000000 ) ;
#4578=EDGE_CURVE ( 'NONE', #9643, #5814, #11338, .T. ) ;
#4579=FACE_OUTER_BOUND ( 'NONE', #10615, .T. ) ;
#4583=DIRECTION ( 'NONE',  ( -0.01206535623792160013, -0.9999272109403024578, 5.877852522924710079E-16 ) ) ;
#4590=LINE ( 'NONE', #14225, #12138 ) ;
#4591=DIRECTION ( 'NONE',  ( -0.3956847857120157075, 0.9183863840214729901, -8.660254037844388394E-16 ) ) ;
#4595=AXIS2_PLACEMENT_3D ( 'NONE', #7520, #10973, #9751 ) ;
#4597=DIRECTION ( 'NONE',  ( -8.018662683283438208E-16, 5.975035461963189015E-16, 1.000000000000000000 ) ) ;
#4598=AXIS2_PLACEMENT_3D ( 'NONE', #10727, #12028, #252 ) ;
#4603=ORIENTED_EDGE ( 'NONE', *, *, #4755, .T. ) ;
#4613=ORIENTED_EDGE ( 'NONE', *, *, #11882, .T. ) ;
#4614=EDGE_CURVE ( 'NONE', #13499, #11960, #11947, .T. ) ;
#4616=ORIENTED_EDGE ( 'NONE', *, *, #1521, .T. ) ;
#4617=ORIENTED_EDGE ( 'NONE', *, *, #5399, .T. ) ;
#4620=ORIENTED_EDGE ( 'NONE', *, *, #1987, .F. ) ;
#4624=EDGE_CURVE ( 'NONE', #2831, #12009, #14013, .T. ) ;
#4626=EDGE_CURVE ( 'NONE', #1378, #6204, #12956, .T. ) ;
#4633=VERTEX_POINT ( 'NONE', #1313 ) ;
#4637=ORIENTED_EDGE ( 'NONE', *, *, #1880, .F. ) ;
#4638=AXIS2_PLACEMENT_3D ( 'NONE', #9072, #4724, #11376 ) ;
#4641=CARTESIAN_POINT ( 'NONE',  ( -18.36422177163696290, -5.957162821864243618, 57.00231026484397745 ) ) ;
#4643=ORIENTED_EDGE ( 'NONE', *, *, #12823, .T. ) ;
#4644=DIRECTION ( 'NONE',  ( -8.018662683283438208E-16, 5.975035461963189015E-16, 1.000000000000000000 ) ) ;
#4650=LINE ( 'NONE', #6772, #368 ) ;
#4651=VECTOR ( 'NONE', #1785, 1000.000000000000114 ) ;
#4654=PLANE ( 'NONE',  #9453 ) ;
#4655=CARTESIAN_POINT ( 'NONE',  ( -22.00391959472895209, -7.178368354675633611, 57.00231026484397745 ) ) ;
#4656=ORIENTED_EDGE ( 'NONE', *, *, #14021, .T. ) ;
#4657=PLANE ( 'NONE',  #2781 ) ;
#4658=ORIENTED_EDGE ( 'NONE', *, *, #13424, .T. ) ;
#4660=DIRECTION ( 'NONE',  ( -8.018662683283438208E-16, 5.975035461963189015E-16, 1.000000000000000000 ) ) ;
#4662=VECTOR ( 'NONE', #13941, 1000.000000000000000 ) ;
#4663=LINE ( 'NONE', #7085, #2748 ) ;
#4665=ADVANCED_FACE ( 'NONE', ( #1387 ), #2313, .F. ) ;
#4666=CARTESIAN_POINT ( 'NONE',  ( -17.81448839017816610, -11.78253482624722004, 51.10586365543726117 ) ) ;
#4667=DIRECTION ( 'NONE',  ( 8.018662683283438208E-16, -5.975035461963189015E-16, -1.000000000000000000 ) ) ;
#4670=CARTESIAN_POINT ( 'NONE',  ( -14.19354049678269192, -21.47604090745013750, 56.85231026484400019 ) ) ;
#4674=EDGE_LOOP ( 'NONE', ( #12620, #4278 ) ) ;
#4675=EDGE_CURVE ( 'NONE', #7160, #2925, #7049, .T. ) ;
#4676=DIRECTION ( 'NONE',  ( 0.5975035461963189576, 0.8018662683283437342, 0.000000000000000000 ) ) ;
#4678=ORIENTED_EDGE ( 'NONE', *, *, #918, .F. ) ;
#4679=CARTESIAN_POINT ( 'NONE',  ( -15.54961651457173488, -13.51026476396819831, 56.85231026484398598 ) ) ;
#4680=EDGE_LOOP ( 'NONE', ( #7542, #13737, #2036, #10008 ) ) ;
#4681=CARTESIAN_POINT ( 'NONE',  ( -15.49969986081092088, -13.50737899243822504, 57.00231026484397745 ) ) ;
#4682=EDGE_CURVE ( 'NONE', #4722, #14217, #9568, .T. ) ;
#4684=CARTESIAN_POINT ( 'NONE',  ( -20.00744539586189319, -5.630737564061013778, 56.85231026484398598 ) ) ;
#4686=EDGE_CURVE ( 'NONE', #3306, #5040, #6950, .T. ) ;
#4687=LINE ( 'NONE', #3609, #14186 ) ;
#4693=ORIENTED_EDGE ( 'NONE', *, *, #15084, .F. ) ;
#4695=ORIENTED_EDGE ( 'NONE', *, *, #9145, .F. ) ;
#4696=CARTESIAN_POINT ( 'NONE',  ( -11.67714598312096008, -19.46131314156662384, 57.00231026484399166 ) ) ;
#4697=ORIENTED_EDGE ( 'NONE', *, *, #6057, .T. ) ;
#4704=VECTOR ( 'NONE', #9987, 1000.000000000000000 ) ;
#4705=DIRECTION ( 'NONE',  ( 8.018662683283438208E-16, -5.975035461963189015E-16, -1.000000000000000000 ) ) ;
#4706=AXIS2_PLACEMENT_3D ( 'NONE', #11944, #6338, #13098 ) ;
#4710=DIRECTION ( 'NONE',  ( -8.018662683283438208E-16, 5.975035461963189015E-16, 1.000000000000000000 ) ) ;
#4711=CARTESIAN_POINT ( 'NONE',  ( -17.81448839017816610, -11.78253482624722537, 51.25231026484399166 ) ) ;
#4715=VERTEX_POINT ( 'NONE', #5968 ) ;
#4719=ORIENTED_EDGE ( 'NONE', *, *, #3707, .T. ) ;
#4720=AXIS2_PLACEMENT_3D ( 'NONE', #10817, #6055, #348 ) ;
#4722=VERTEX_POINT ( 'NONE', #1234 ) ;
#4724=DIRECTION ( 'NONE',  ( -0.4274949678123940999, 0.9040177279761056894, -8.829475928589322242E-16 ) ) ;
#4725=AXIS2_PLACEMENT_3D ( 'NONE', #6186, #14312, #12867 ) ;
#4726=CARTESIAN_POINT ( 'NONE',  ( -11.61446667642527331, -19.42012692406430574, 56.85231026484400019 ) ) ;
#4728=ORIENTED_EDGE ( 'NONE', *, *, #5985, .F. ) ;
#4729=AXIS2_PLACEMENT_3D ( 'NONE', #9841, #4253, #7534 ) ;
#4731=ORIENTED_EDGE ( 'NONE', *, *, #10381, .T. ) ;
#4732=EDGE_CURVE ( 'NONE', #337, #12833, #14086, .T. ) ;
#4733=DIRECTION ( 'NONE',  ( 0.5104125104779002609, 0.8599296884906623140, -1.045284632676510365E-16 ) ) ;
#4735=DIRECTION ( 'NONE',  ( 0.5975035461963188466, 0.8018662683283437342, 0.000000000000000000 ) ) ;
#4736=ORIENTED_EDGE ( 'NONE', *, *, #4279, .F. ) ;
#4738=CARTESIAN_POINT ( 'NONE',  ( -15.49969986081092088, -13.50737899243822504, 57.00231026484397745 ) ) ;
#4739=VECTOR ( 'NONE', #9918, 1000.000000000000114 ) ;
#4740=PLANE ( 'NONE',  #11538 ) ;
#4743=VECTOR ( 'NONE', #2937, 1000.000000000000000 ) ;
#4745=CARTESIAN_POINT ( 'NONE',  ( -10.85342163307452523, -20.71489927548028476, 56.85231026484400019 ) ) ;
#4746=DIRECTION ( 'NONE',  ( 0.09252159378507134047, -0.9957106782009873536, 6.691306063588577540E-16 ) ) ;
#4751=VERTEX_POINT ( 'NONE', #1550 ) ;
#4753=ORIENTED_EDGE ( 'NONE', *, *, #13475, .T. ) ;
#4755=EDGE_CURVE ( 'NONE', #14491, #5023, #1477, .T. ) ;
#4756=CARTESIAN_POINT ( 'NONE',  ( -25.45346213993001783, -14.15794911993139849, 57.00231026484397745 ) ) ;
#4759=DIRECTION ( 'NONE',  ( 8.018662683283438208E-16, -5.975035461963189015E-16, -1.000000000000000000 ) ) ;
#4765=DIRECTION ( 'NONE',  ( 8.018662683283438208E-16, -5.975035461963189015E-16, -1.000000000000000000 ) ) ;
#4766=DIRECTION ( 'NONE',  ( -0.9183863840214728791, -0.3956847857120156520, -4.999999999999998416E-16 ) ) ;
#4767=EDGE_CURVE ( 'NONE', #4359, #15022, #1772, .T. ) ;
#4768=ORIENTED_EDGE ( 'NONE', *, *, #729, .T. ) ;
#4770=EDGE_CURVE ( 'NONE', #5960, #12566, #341, .T. ) ;
#4772=ORIENTED_EDGE ( 'NONE', *, *, #14611, .T. ) ;
#4774=VECTOR ( 'NONE', #10568, 1000.000000000000114 ) ;
#4776=DIRECTION ( 'NONE',  ( -0.5491495666976170531, 0.8357240892757724637, -9.396926207859082113E-16 ) ) ;
#4778=LINE ( 'NONE', #5008, #10820 ) ;
#4779=EDGE_CURVE ( 'NONE', #5304, #13197, #1697, .T. ) ;
#4781=DIRECTION ( 'NONE',  ( 0.5975035461963189576, 0.8018662683283437342, 0.000000000000000000 ) ) ;
#4783=EDGE_CURVE ( 'NONE', #14533, #6892, #12181, .T. ) ;
#4784=DIRECTION ( 'NONE',  ( -0.5975035461963187355, -0.8018662683283439563, 0.000000000000000000 ) ) ;
#4786=LINE ( 'NONE', #14041, #8019 ) ;
#4787=ORIENTED_EDGE ( 'NONE', *, *, #8377, .T. ) ;
#4788=PLANE ( 'NONE',  #14842 ) ;
#4791=EDGE_LOOP ( 'NONE', ( #13318, #1713, #4411, #9861 ) ) ;
#4792=ORIENTED_EDGE ( 'NONE', *, *, #6824, .F. ) ;
#4796=AXIS2_PLACEMENT_3D ( 'NONE', #2940, #12277, #7810 ) ;
#4797=VECTOR ( 'NONE', #5711, 1000.000000000000000 ) ;
#4798=DIRECTION ( 'NONE',  ( 8.018662683283438208E-16, -5.975035461963189015E-16, -1.000000000000000000 ) ) ;
#4801=DIRECTION ( 'NONE',  ( -8.018662683283438208E-16, 5.975035461963189015E-16, 1.000000000000000000 ) ) ;
#4802=DIRECTION ( 'NONE',  ( -8.018662683283438208E-16, 5.975035461963189015E-16, 1.000000000000000000 ) ) ;
#4805=CARTESIAN_POINT ( 'NONE',  ( -9.884208147447518300, -5.263176313152190922, 57.00231026484397745 ) ) ;
#4807=CARTESIAN_POINT ( 'NONE',  ( -15.04562126104788966, -5.444807279564146896, 57.00231026484397745 ) ) ;
#4810=ORIENTED_EDGE ( 'NONE', *, *, #1987, .T. ) ;
#4811=CARTESIAN_POINT ( 'NONE',  ( -15.50552586659557797, -13.55703840903364288, 56.85231026484398598 ) ) ;
#4812=CARTESIAN_POINT ( 'NONE',  ( -10.72806301968316411, -20.63252684047564500, 57.00231026484399166 ) ) ;
#4814=CARTESIAN_POINT ( 'NONE',  ( -6.938526287600614850, -8.388108336439911383, 54.00231026484399166 ) ) ;
#4817=( NAMED_UNIT ( * ) SI_UNIT ( $, .STERADIAN. ) SOLID_ANGLE_UNIT ( ) );
#4820=CARTESIAN_POINT ( 'NONE',  ( -7.985436018829471294, -20.06759727486528178, 57.00231026484399166 ) ) ;
#4823=ORIENTED_EDGE ( 'NONE', *, *, #9988, .T. ) ;
#4827=DIRECTION ( 'NONE',  ( 0.8018662683283437342, -0.5975035461963188466, 1.000000000000000078E-15 ) ) ;
#4829=DIRECTION ( 'NONE',  ( -8.018662683283438208E-16, 5.975035461963189015E-16, 1.000000000000000000 ) ) ;
#4831=VERTEX_POINT ( 'NONE', #5288 ) ;
#4835=ORIENTED_EDGE ( 'NONE', *, *, #7290, .T. ) ;
#4837=EDGE_LOOP ( 'NONE', ( #6587, #860, #3926, #7742 ) ) ;
#4839=EDGE_CURVE ( 'NONE', #9919, #11420, #1623, .T. ) ;
#4843=AXIS2_PLACEMENT_3D ( 'NONE', #171, #1384, #3684 ) ;
#4845=DIRECTION ( 'NONE',  ( -8.018662683283438208E-16, 5.975035461963189015E-16, 1.000000000000000000 ) ) ;
#4847=VERTEX_POINT ( 'NONE', #8577 ) ;
#4850=ORIENTED_EDGE ( 'NONE', *, *, #4003, .F. ) ;
#4853=PLANE ( 'NONE',  #4207 ) ;
#4854=EDGE_LOOP ( 'NONE', ( #11500, #14234, #12965, #2157 ) ) ;
#4855=VECTOR ( 'NONE', #1073, 1000.000000000000000 ) ;
#4856=PLANE ( 'NONE',  #1540 ) ;
#4862=VECTOR ( 'NONE', #8762, 1000.000000000000227 ) ;
#4863=DIRECTION ( 'NONE',  ( -0.9183863840214728791, -0.3956847857120156520, -4.999999999999998416E-16 ) ) ;
#4865=PLANE ( 'NONE',  #13419 ) ;
#4866=ORIENTED_EDGE ( 'NONE', *, *, #11826, .T. ) ;
#4867=LINE ( 'NONE', #9372, #9220 ) ;
#4871=ORIENTED_EDGE ( 'NONE', *, *, #6384, .F. ) ;
#4874=AXIS2_PLACEMENT_3D ( 'NONE', #10493, #5886, #4759 ) ;
#4875=FACE_OUTER_BOUND ( 'NONE', #9143, .T. ) ;
#4876=ADVANCED_FACE ( 'NONE', ( #14696 ), #1850, .F. ) ;
#4878=PLANE ( 'NONE',  #4882 ) ;
#4880=CARTESIAN_POINT ( 'NONE',  ( -7.145558396657058609, -18.95797028117975103, 57.00231026484399166 ) ) ;
#4882=AXIS2_PLACEMENT_3D ( 'NONE', #436, #5025, #14280 ) ;
#4883=DIRECTION ( 'NONE',  ( 0.5975035461963189576, 0.8018662683283437342, 0.000000000000000000 ) ) ;
#4885=ORIENTED_EDGE ( 'NONE', *, *, #1824, .F. ) ;
#4886=CARTESIAN_POINT ( 'NONE',  ( -16.57334897777262483, -22.01522992987520766, 56.85231026484400019 ) ) ;
#4887=LINE ( 'NONE', #5033, #4082 ) ;
#4890=CARTESIAN_POINT ( 'NONE',  ( -18.04596724311489808, -11.61005040962811563, 57.00231026484397745 ) ) ;
#4891=ORIENTED_EDGE ( 'NONE', *, *, #4925, .T. ) ;
#4893=VERTEX_POINT ( 'NONE', #2208 ) ;
#4894=DIRECTION ( 'NONE',  ( -0.1165201156931293391, -0.9931883319083343320, 4.999999999999998416E-16 ) ) ;
#4895=DIRECTION ( 'NONE',  ( -0.8018662683283437342, 0.5975035461963188466, -1.000000000000000078E-15 ) ) ;
#4896=VECTOR ( 'NONE', #14652, 1000.000000000000000 ) ;
#4897=CARTESIAN_POINT ( 'NONE',  ( -14.51048789653087390, -15.80334495249191207, 51.25231026484399166 ) ) ;
#4901=VECTOR ( 'NONE', #3456, 1000.000000000000000 ) ;
#4903=LINE ( 'NONE', #2675, #2867 ) ;
#4904=DIRECTION ( 'NONE',  ( -8.018662683283438208E-16, 5.975035461963189015E-16, 1.000000000000000000 ) ) ;
#4906=VERTEX_POINT ( 'NONE', #2363 ) ;
#4910=ORIENTED_EDGE ( 'NONE', *, *, #5064, .F. ) ;
#4914=CARTESIAN_POINT ( 'NONE',  ( -25.29546517631143132, -15.38982603914036140, 57.00231026484397745 ) ) ;
#4920=CARTESIAN_POINT ( 'NONE',  ( -12.87131257180735844, -22.19373785326158099, 56.85231026484400019 ) ) ;
#4922=ORIENTED_EDGE ( 'NONE', *, *, #4318, .T. ) ;
#4923=ORIENTED_EDGE ( 'NONE', *, *, #8362, .F. ) ;
#4925=EDGE_CURVE ( 'NONE', #7427, #2588, #11539, .T. ) ;
#4926=LINE ( 'NONE', #35, #12269 ) ;
#4928=EDGE_CURVE ( 'NONE', #11333, #10194, #7721, .T. ) ;
#4929=DIRECTION ( 'NONE',  ( 8.018662683283438208E-16, -5.975035461963189015E-16, -1.000000000000000000 ) ) ;
#4930=CIRCLE ( 'NONE', #10284, 9.974999999999999645 ) ;
#4931=DIRECTION ( 'NONE',  ( -8.018662683283438208E-16, 5.975035461963189015E-16, 1.000000000000000000 ) ) ;
#4932=LINE ( 'NONE', #351, #7772 ) ;
#4933=VECTOR ( 'NONE', #2545, 1000.000000000000114 ) ;
#4934=CARTESIAN_POINT ( 'NONE',  ( -23.68291657637574232, -19.21137664199072148, 54.00231026484399166 ) ) ;
#4936=FACE_OUTER_BOUND ( 'NONE', #990, .T. ) ;
#4938=LINE ( 'NONE', #358, #1906 ) ;
#4940=ORIENTED_EDGE ( 'NONE', *, *, #13383, .F. ) ;
#4946=CARTESIAN_POINT ( 'NONE',  ( -16.73644428586259636, -23.40541355628490550, 57.00231026484399166 ) ) ;
#4947=EDGE_CURVE ( 'NONE', #10177, #9929, #3504, .T. ) ;
#4949=AXIS2_PLACEMENT_3D ( 'NONE', #7488, #1463, #14459 ) ;
#4952=CARTESIAN_POINT ( 'NONE',  ( -15.49969986081092088, -13.50737899243822504, 56.85231026484398598 ) ) ;
#4953=CARTESIAN_POINT ( 'NONE',  ( -15.16333526000374832, -10.64029123852186487, 51.25231026484399166 ) ) ;
#4957=DIRECTION ( 'NONE',  ( -0.7953815700667019595, -0.6061090314442014737, -2.756373558169989438E-16 ) ) ;
#4958=PLANE ( 'NONE',  #8753 ) ;
#4960=VECTOR ( 'NONE', #926, 1000.000000000000114 ) ;
#4961=EDGE_CURVE ( 'NONE', #6605, #14388, #8162, .T. ) ;
#4962=DIRECTION ( 'NONE',  ( -8.018662683283438208E-16, 5.975035461963189015E-16, 1.000000000000000000 ) ) ;
#4963=EDGE_CURVE ( 'NONE', #11221, #7892, #9233, .T. ) ;
#4965=ORIENTED_EDGE ( 'NONE', *, *, #10247, .F. ) ;
#4966=DIRECTION ( 'NONE',  ( -8.018662683283438208E-16, 5.975035461963189015E-16, 1.000000000000000000 ) ) ;
#4967=ORIENTED_EDGE ( 'NONE', *, *, #10174, .T. ) ;
#4968=DIRECTION ( 'NONE',  ( -0.5975035461963188466, -0.8018662683283439563, 0.000000000000000000 ) ) ;
#4970=CARTESIAN_POINT ( 'NONE',  ( -20.69940085690220144, -18.30574950243923027, 57.00231026484397745 ) ) ;
#4971=ADVANCED_FACE ( 'NONE', ( #4579 ), #5860, .T. ) ;
#4972=VECTOR ( 'NONE', #10553, 1000.000000000000227 ) ;
#4975=ORIENTED_EDGE ( 'NONE', *, *, #8399, .T. ) ;
#4976=CARTESIAN_POINT ( 'NONE',  ( -13.81224214977857123, -23.33861042463823665, 56.85231026484400019 ) ) ;
#4977=CARTESIAN_POINT ( 'NONE',  ( -9.002116193859002635, -10.70790913352571927, 56.85231026484400019 ) ) ;
#4978=DIRECTION ( 'NONE',  ( -8.018662683283438208E-16, 5.975035461963189015E-16, 1.000000000000000000 ) ) ;
#4979=ORIENTED_EDGE ( 'NONE', *, *, #3185, .T. ) ;
#4980=DIRECTION ( 'NONE',  ( 8.018662683283438208E-16, -5.975035461963189015E-16, -1.000000000000000000 ) ) ;
#4981=ADVANCED_FACE ( 'NONE', ( #701 ), #988, .T. ) ;
#4983=VERTEX_POINT ( 'NONE', #3428 ) ;
#4985=ORIENTED_EDGE ( 'NONE', *, *, #14035, .T. ) ;
#4987=AXIS2_PLACEMENT_3D ( 'NONE', #3506, #6090, #4735 ) ;
#4989=DIRECTION ( 'NONE',  ( -0.9931883319083343320, 0.1165201156931299220, 0.000000000000000000 ) ) ;
#4993=DIRECTION ( 'NONE',  ( -8.018662683283438208E-16, 5.975035461963189015E-16, 1.000000000000000000 ) ) ;
#4995=EDGE_CURVE ( 'NONE', #5453, #8707, #15119, .T. ) ;
#4996=VECTOR ( 'NONE', #5264, 1000.000000000000114 ) ;
#4998=FACE_OUTER_BOUND ( 'NONE', #5811, .T. ) ;
#4999=ORIENTED_EDGE ( 'NONE', *, *, #593, .F. ) ;
#5001=AXIS2_PLACEMENT_3D ( 'NONE', #5506, #13699, #999 ) ;
#5002=ORIENTED_EDGE ( 'NONE', *, *, #7037, .T. ) ;
#5007=FACE_OUTER_BOUND ( 'NONE', #12198, .T. ) ;
#5008=CARTESIAN_POINT ( 'NONE',  ( -24.85752488709640318, -10.05314452190415508, 54.00231026484397745 ) ) ;
#5009=VECTOR ( 'NONE', #7625, 1000.000000000000000 ) ;
#5012=EDGE_CURVE ( 'NONE', #4831, #14554, #10388, .T. ) ;
#5016=LINE ( 'NONE', #1790, #9623 ) ;
#5017=VERTEX_POINT ( 'NONE', #5939 ) ;
#5023=VERTEX_POINT ( 'NONE', #12999 ) ;
#5025=DIRECTION ( 'NONE',  ( -8.018662683283439195E-16, 5.975035461963190001E-16, 1.000000000000000000 ) ) ;
#5026=EDGE_CURVE ( 'NONE', #11857, #2792, #8238, .T. ) ;
#5028=LINE ( 'NONE', #14205, #883 ) ;
#5029=LINE ( 'NONE', #440, #5448 ) ;
#5030=EDGE_CURVE ( 'NONE', #14164, #17, #11839, .T. ) ;
#5031=ORIENTED_EDGE ( 'NONE', *, *, #8998, .F. ) ;
#5032=CARTESIAN_POINT ( 'NONE',  ( -16.32149003149045896, -5.473954385499117947, 57.00231026484397745 ) ) ;
#5033=CARTESIAN_POINT ( 'NONE',  ( -7.985436018829467741, -20.06759727486528533, 54.00231026484400587 ) ) ;
#5034=ORIENTED_EDGE ( 'NONE', *, *, #3225, .T. ) ;
#5036=LINE ( 'NONE', #12221, #1153 ) ;
#5039=DIRECTION ( 'NONE',  ( -8.018662683283439195E-16, 5.975035461963190001E-16, 1.000000000000000000 ) ) ;
#5040=VERTEX_POINT ( 'NONE', #4807 ) ;
#5049=EDGE_LOOP ( 'NONE', ( #14582, #12983, #7717, #3897 ) ) ;
#5051=DIRECTION ( 'NONE',  ( -8.018662683283438208E-16, 5.975035461963189015E-16, 1.000000000000000000 ) ) ;
#5053=DIRECTION ( 'NONE',  ( 0.8357240892757724637, 0.5491495666976171641, 3.420201433256690644E-16 ) ) ;
#5056=ORIENTED_EDGE ( 'NONE', *, *, #747, .F. ) ;
#5059=CYLINDRICAL_SURFACE ( 'NONE', #1770, 0.2500000000000014433 ) ;
#5061=ORIENTED_EDGE ( 'NONE', *, *, #13777, .F. ) ;
#5064=EDGE_CURVE ( 'NONE', #1451, #13944, #14368, .T. ) ;
#5068=PLANE ( 'NONE',  #456 ) ;
#5071=VERTEX_POINT ( 'NONE', #12927 ) ;
#5073=ORIENTED_EDGE ( 'NONE', *, *, #3030, .F. ) ;
#5074=VECTOR ( 'NONE', #3032, 1000.000000000000000 ) ;
#5075=EDGE_LOOP ( 'NONE', ( #5141, #14047, #7371, #207 ) ) ;
#5076=DIRECTION ( 'NONE',  ( 8.018662683283438208E-16, -5.975035461963189015E-16, -1.000000000000000000 ) ) ;
#5077=ORIENTED_EDGE ( 'NONE', *, *, #2819, .F. ) ;
#5078=ORIENTED_EDGE ( 'NONE', *, *, #3431, .T. ) ;
#5082=AXIS2_PLACEMENT_3D ( 'NONE', #9763, #14428, #3948 ) ;
#5083=FACE_OUTER_BOUND ( 'NONE', #5291, .T. ) ;
#5085=DIRECTION ( 'NONE',  ( 0.5975035461963189576, 0.8018662683283437342, 0.000000000000000000 ) ) ;
#5086=CARTESIAN_POINT ( 'NONE',  ( -15.49969986081092088, -13.50737899243822504, 56.85231026484398598 ) ) ;
#5088=ORIENTED_EDGE ( 'NONE', *, *, #8757, .F. ) ;
#5091=VECTOR ( 'NONE', #7980, 1000.000000000000000 ) ;
#5093=ORIENTED_EDGE ( 'NONE', *, *, #6985, .T. ) ;
#5099=ADVANCED_FACE ( 'NONE', ( #14139 ), #3660, .F. ) ;
#5100=EDGE_CURVE ( 'NONE', #8254, #12536, #12192, .T. ) ;
#5101=CARTESIAN_POINT ( 'NONE',  ( -8.194314379747492438, -16.94868586237404529, 57.00231026484399166 ) ) ;
#5105=ORIENTED_EDGE ( 'NONE', *, *, #14953, .F. ) ;
#5114=EDGE_CURVE ( 'NONE', #3941, #12614, #6011, .T. ) ;
#5115=DIRECTION ( 'NONE',  ( -8.018662683283438208E-16, 5.975035461963189015E-16, 1.000000000000000000 ) ) ;
#5116=VECTOR ( 'NONE', #3771, 1000.000000000000000 ) ;
#5120=ORIENTED_EDGE ( 'NONE', *, *, #3814, .F. ) ;
#5123=ORIENTED_EDGE ( 'NONE', *, *, #12518, .F. ) ;
#5125=ORIENTED_EDGE ( 'NONE', *, *, #10846, .F. ) ;
#5128=ORIENTED_EDGE ( 'NONE', *, *, #354, .F. ) ;
#5132=ORIENTED_EDGE ( 'NONE', *, *, #12664, .F. ) ;
#5136=CARTESIAN_POINT ( 'NONE',  ( -12.81093390292742740, -9.898980784960722090, -13.99768973515600301 ) ) ;
#5141=ORIENTED_EDGE ( 'NONE', *, *, #12469, .T. ) ;
#5142=ORIENTED_EDGE ( 'NONE', *, *, #4317, .F. ) ;
#5144=CARTESIAN_POINT ( 'NONE',  ( -15.34686821047329808, -23.48120812104550481, 56.85231026484400019 ) ) ;
#5148=DIRECTION ( 'NONE',  ( 0.5975035461963189576, 0.8018662683283437342, 0.000000000000000000 ) ) ;
#5149=CARTESIAN_POINT ( 'NONE',  ( -14.95642007119156425, -3.547184613301258782, 57.00231026484397745 ) ) ;
#5150=DIRECTION ( 'NONE',  ( -8.018662683283439195E-16, 5.975035461963190001E-16, 1.000000000000000000 ) ) ;
#5151=DIRECTION ( 'NONE',  ( 0.5975035461963189576, 0.8018662683283437342, 0.000000000000000000 ) ) ;
#5154=EDGE_LOOP ( 'NONE', ( #5783, #11649, #12121, #3903 ) ) ;
#5155=CARTESIAN_POINT ( 'NONE',  ( -15.19545581216392627, -5.437764035151672282, 56.85231026484398598 ) ) ;
#5158=VECTOR ( 'NONE', #15115, 999.9999999999998863 ) ;
#5159=DIRECTION ( 'NONE',  ( 0.5975035461963189576, 0.8018662683283437342, 0.000000000000000000 ) ) ;
#5160=EDGE_CURVE ( 'NONE', #118, #10152, #3957, .T. ) ;
#5166=VECTOR ( 'NONE', #12635, 1000.000000000000000 ) ;
#5167=LINE ( 'NONE', #8679, #14597 ) ;
#5169=CARTESIAN_POINT ( 'NONE',  ( -10.07958688850791162, -7.521259601090221736, 56.85231026484398598 ) ) ;
#5173=CARTESIAN_POINT ( 'NONE',  ( -15.49969986081092088, -13.50737899243822504, 56.85231026484398598 ) ) ;
#5177=ORIENTED_EDGE ( 'NONE', *, *, #2672, .T. ) ;
#5179=ORIENTED_EDGE ( 'NONE', *, *, #288, .F. ) ;
#5185=VECTOR ( 'NONE', #4107, 1000.000000000000000 ) ;
#5188=EDGE_CURVE ( 'NONE', #8489, #11739, #446, .T. ) ;
#5189=VECTOR ( 'NONE', #14299, 999.9999999999998863 ) ;
#5192=VERTEX_POINT ( 'NONE', #5329 ) ;
#5193=CARTESIAN_POINT ( 'NONE',  ( -13.96026682931439211, -23.36287344688023992, 57.00231026484399166 ) ) ;
#5195=ORIENTED_EDGE ( 'NONE', *, *, #2438, .F. ) ;
#5196=EDGE_LOOP ( 'NONE', ( #3635, #12276, #4408, #3198 ) ) ;
#5202=ORIENTED_EDGE ( 'NONE', *, *, #10459, .F. ) ;
#5203=CIRCLE ( 'NONE', #806, 9.974999999999999645 ) ;
#5204=LINE ( 'NONE', #5501, #2258 ) ;
#5208=EDGE_CURVE ( 'NONE', #13485, #1568, #13521, .T. ) ;
#5210=VECTOR ( 'NONE', #2924, 1000.000000000000114 ) ;
#5211=CARTESIAN_POINT ( 'NONE',  ( -16.38999062866295020, -11.44100962838991364, 51.00231026484399166 ) ) ;
#5212=EDGE_CURVE ( 'NONE', #11184, #9718, #3031, .T. ) ;
#5213=ORIENTED_EDGE ( 'NONE', *, *, #4624, .T. ) ;
#5214=CARTESIAN_POINT ( 'NONE',  ( -19.68577560955674954, -20.41303028871448788, 57.00231026484397745 ) ) ;
#5217=ORIENTED_EDGE ( 'NONE', *, *, #14933, .T. ) ;
#5220=ORIENTED_EDGE ( 'NONE', *, *, #14468, .T. ) ;
#5222=CARTESIAN_POINT ( 'NONE',  ( -18.54556661251663030, -20.98627902725976213, 56.85231026484398598 ) ) ;
#5223=ORIENTED_EDGE ( 'NONE', *, *, #11984, .F. ) ;
#5227=DIRECTION ( 'NONE',  ( -0.9183863840214729901, -0.3956847857120157075, -4.999999999999999402E-16 ) ) ;
#5228=EDGE_CURVE ( 'NONE', #2134, #572, #9334, .T. ) ;
#5229=EDGE_CURVE ( 'NONE', #8291, #14012, #550, .T. ) ;
#5234=ORIENTED_EDGE ( 'NONE', *, *, #12244, .F. ) ;
#5237=PLANE ( 'NONE',  #7149 ) ;
#5238=ORIENTED_EDGE ( 'NONE', *, *, #1315, .T. ) ;
#5240=VECTOR ( 'NONE', #14599, 999.9999999999998863 ) ;
#5243=ADVANCED_FACE ( 'NONE', ( #14814 ), #6608, .T. ) ;
#5249=EDGE_CURVE ( 'NONE', #12040, #8177, #3414, .T. ) ;
#5250=CARTESIAN_POINT ( 'NONE',  ( -23.43263029221230198, -15.01730109988151440, 56.85231026484398598 ) ) ;
#5254=CARTESIAN_POINT ( 'NONE',  ( -23.55378106252664239, -12.92169478045303066, 56.85231026484398598 ) ) ;
#5255=ORIENTED_EDGE ( 'NONE', *, *, #2531, .T. ) ;
#5257=CARTESIAN_POINT ( 'NONE',  ( -23.37741044072812713, -11.73331557219068877, 56.85231026484398598 ) ) ;
#5259=VECTOR ( 'NONE', #8646, 1000.000000000000000 ) ;
#5260=EDGE_CURVE ( 'NONE', #4893, #1960, #11519, .T. ) ;
#5262=CARTESIAN_POINT ( 'NONE',  ( -18.68395610307571530, -20.92841410781112899, 56.85231026484398598 ) ) ;
#5264=DIRECTION ( 'NONE',  ( -0.8934395198752397294, 0.4491835085186243748, -9.848077530122081084E-16 ) ) ;
#5265=ORIENTED_EDGE ( 'NONE', *, *, #6658, .F. ) ;
#5267=CARTESIAN_POINT ( 'NONE',  ( -21.89842656004739396, -7.071732433740530510, 57.00231026484397745 ) ) ;
#5275=EDGE_CURVE ( 'NONE', #12154, #8967, #10561, .T. ) ;
#5278=CARTESIAN_POINT ( 'NONE',  ( -23.41792317787242084, -15.09084496969942535, 56.85231026484398598 ) ) ;
#5279=AXIS2_PLACEMENT_3D ( 'NONE', #11304, #10071, #14822 ) ;
#5282=FACE_OUTER_BOUND ( 'NONE', #13096, .T. ) ;
#5286=CARTESIAN_POINT ( 'NONE',  ( -17.87376992080280758, -22.26666214519964271, 56.85231026484400019 ) ) ;
#5288=CARTESIAN_POINT ( 'NONE',  ( -8.194314379747492438, -16.94868586237404529, 56.85231026484400019 ) ) ;
#5291=EDGE_LOOP ( 'NONE', ( #4731, #9413, #6379, #9356 ) ) ;
#5293=DIRECTION ( 'NONE',  ( -8.018662683283438208E-16, 5.975035461963189015E-16, 1.000000000000000000 ) ) ;
#5294=EDGE_LOOP ( 'NONE', ( #4011, #2796, #14760, #3377 ) ) ;
#5295=CIRCLE ( 'NONE', #12885, 9.974999999999999645 ) ;
#5299=PLANE ( 'NONE',  #11448 ) ;
#5301=VECTOR ( 'NONE', #13930, 1000.000000000000114 ) ;
#5302=DIRECTION ( 'NONE',  ( -0.1617534816134003905, 0.9868311969055008070, -7.193398003386493154E-16 ) ) ;
#5304=VERTEX_POINT ( 'NONE', #13895 ) ;
#5305=CARTESIAN_POINT ( 'NONE',  ( -6.309378268457435546, -9.629413800598410234, 57.00231026484399166 ) ) ;
#5306=VERTEX_POINT ( 'NONE', #3189 ) ;
#5314=EDGE_CURVE ( 'NONE', #1146, #2196, #14469, .T. ) ;
#5317=CARTESIAN_POINT ( 'NONE',  ( -18.86735971344653962, -5.080035572537331845, 56.85231026484398598 ) ) ;
#5318=CARTESIAN_POINT ( 'NONE',  ( -22.58324314276470091, -9.630648466248954875, 56.85231026484398598 ) ) ;
#5319=LINE ( 'NONE', #14802, #5324 ) ;
#5321=EDGE_CURVE ( 'NONE', #13197, #6348, #6687, .T. ) ;
#5322=FACE_OUTER_BOUND ( 'NONE', #9581, .T. ) ;
#5324=VECTOR ( 'NONE', #4325, 1000.000000000000000 ) ;
#5325=VERTEX_POINT ( 'NONE', #4641 ) ;
#5327=CARTESIAN_POINT ( 'NONE',  ( -15.49969986081091378, -13.50737899243822859, 51.00031026484398922 ) ) ;
#5329=CARTESIAN_POINT ( 'NONE',  ( -12.95343247850694723, -15.40470757524832912, 57.00231026484399166 ) ) ;
#5330=LINE ( 'NONE', #4416, #5074 ) ;
#5332=EDGE_LOOP ( 'NONE', ( #11663, #12308, #6014, #8597 ) ) ;
#5333=PLANE ( 'NONE',  #6614 ) ;
#5336=AXIS2_PLACEMENT_3D ( 'NONE', #11316, #3209, #13692 ) ;
#5337=CARTESIAN_POINT ( 'NONE',  ( -24.06473463808513813, -13.92741382918746496, 56.85231026484398598 ) ) ;
#5340=FACE_OUTER_BOUND ( 'NONE', #3761, .T. ) ;
#5343=CARTESIAN_POINT ( 'NONE',  ( -18.18846581869434686, -17.11577719991577951, 46.00231026484398456 ) ) ;
#5345=ORIENTED_EDGE ( 'NONE', *, *, #4492, .F. ) ;
#5349=CARTESIAN_POINT ( 'NONE',  ( -6.468284635389317749, -17.74225372801457112, 54.00231026484400587 ) ) ;
#5351=EDGE_CURVE ( 'NONE', #1855, #9677, #2346, .T. ) ;
#5352=VECTOR ( 'NONE', #7271, 1000.000000000000114 ) ;
#5353=DIRECTION ( 'NONE',  ( -8.018662683283438208E-16, 5.975035461963189015E-16, 1.000000000000000000 ) ) ;
#5355=CARTESIAN_POINT ( 'NONE',  ( -13.18491133144367744, -15.23222315862922471, 56.75231026484399166 ) ) ;
#5358=DIRECTION ( 'NONE',  ( -0.5691548339926102429, -0.8222303661035904598, 3.489949670250058899E-17 ) ) ;
#5360=EDGE_CURVE ( 'NONE', #2549, #11181, #8452, .T. ) ;
#5362=ORIENTED_EDGE ( 'NONE', *, *, #5321, .F. ) ;
#5364=EDGE_LOOP ( 'NONE', ( #2458, #1604, #3129, #10667 ) ) ;
#5367=VERTEX_POINT ( 'NONE', #131 ) ;
#5370=CARTESIAN_POINT ( 'NONE',  ( -13.88982576282654691, -4.575998618238553917, 56.85231026484398598 ) ) ;
#5372=FACE_OUTER_BOUND ( 'NONE', #7952, .T. ) ;
#5374=CYLINDRICAL_SURFACE ( 'NONE', #13414, 0.2499999999999996947 ) ;
#5378=PLANE ( 'NONE',  #12989 ) ;
#5379=ORIENTED_EDGE ( 'NONE', *, *, #13881, .T. ) ;
#5384=ORIENTED_EDGE ( 'NONE', *, *, #15059, .T. ) ;
#5387=DIRECTION ( 'NONE',  ( 8.018662683283438208E-16, -5.975035461963189015E-16, -1.000000000000000000 ) ) ;
#5388=DIRECTION ( 'NONE',  ( -8.018662683283439195E-16, 5.975035461963190001E-16, 1.000000000000000000 ) ) ;
#5389=LINE ( 'NONE', #11213, #686 ) ;
#5391=EDGE_CURVE ( 'NONE', #8928, #572, #3716, .T. ) ;
#5392=CARTESIAN_POINT ( 'NONE',  ( -12.58343141761905670, -12.25091104594033098, 57.00231026484397745 ) ) ;
#5394=ORIENTED_EDGE ( 'NONE', *, *, #10848, .T. ) ;
#5396=DIRECTION ( 'NONE',  ( -0.9997391571607663341, -0.02283895005206026604, -7.880107536067206944E-16 ) ) ;
#5397=ORIENTED_EDGE ( 'NONE', *, *, #227, .T. ) ;
#5398=CARTESIAN_POINT ( 'NONE',  ( -10.72806301968316411, -20.63252684047564500, 56.85231026484400019 ) ) ;
#5399=EDGE_CURVE ( 'NONE', #13689, #13829, #11054, .T. ) ;
#5401=CARTESIAN_POINT ( 'NONE',  ( -5.526612771747951847, -13.70272205979775393, 54.00231026484399166 ) ) ;
#5402=ORIENTED_EDGE ( 'NONE', *, *, #3652, .T. ) ;
#5403=CARTESIAN_POINT ( 'NONE',  ( -17.40065610530428586, -5.145404622917534532, 56.85231026484398598 ) ) ;
#5404=VECTOR ( 'NONE', #8068, 1000.000000000000000 ) ;
#5408=EDGE_CURVE ( 'NONE', #6205, #9738, #14276, .T. ) ;
#5409=DIRECTION ( 'NONE',  ( 0.7276687409742212953, 0.6859287159822015090, 1.736481776669299976E-16 ) ) ;
#5410=VECTOR ( 'NONE', #8509, 1000.000000000000000 ) ;
#5413=EDGE_CURVE ( 'NONE', #10807, #6204, #3564, .T. ) ;
#5419=ORIENTED_EDGE ( 'NONE', *, *, #1134, .F. ) ;
#5424=PLANE ( 'NONE',  #6393 ) ;
#5427=AXIS2_PLACEMENT_3D ( 'NONE', #4811, #2366, #8316 ) ;
#5430=EDGE_CURVE ( 'NONE', #11463, #2715, #3868, .T. ) ;
#5432=LINE ( 'NONE', #852, #7917 ) ;
#5433=CARTESIAN_POINT ( 'NONE',  ( -15.83606446161809167, -16.37446674635458876, 56.89875687425071504 ) ) ;
#5434=CARTESIAN_POINT ( 'NONE',  ( -14.10579935493720782, -22.47500361547664127, 57.00231026484399166 ) ) ;
#5435=ORIENTED_EDGE ( 'NONE', *, *, #12415, .F. ) ;
#5437=ORIENTED_EDGE ( 'NONE', *, *, #4092, .F. ) ;
#5443=CARTESIAN_POINT ( 'NONE',  ( -9.969334273478565933, -7.622966832294271633, 57.00231026484397745 ) ) ;
#5446=CARTESIAN_POINT ( 'NONE',  ( -15.49969986081091378, -13.50737899243822859, 51.00031026484398922 ) ) ;
#5448=VECTOR ( 'NONE', #7308, 1000.000000000000114 ) ;
#5449=DIRECTION ( 'NONE',  ( -0.7511640317997414495, -0.6601155939154573771, -2.079116908177570050E-16 ) ) ;
#5450=PLANE ( 'NONE',  #13508 ) ;
#5451=VERTEX_POINT ( 'NONE', #7525 ) ;
#5453=VERTEX_POINT ( 'NONE', #1572 ) ;
#5458=DIRECTION ( 'NONE',  ( -0.6601155939154559338, 0.7511640317997426708, -9.781476007338054812E-16 ) ) ;
#5460=FACE_OUTER_BOUND ( 'NONE', #14290, .T. ) ;
#5462=EDGE_CURVE ( 'NONE', #13117, #14849, #10804, .T. ) ;
#5465=CIRCLE ( 'NONE', #596, 9.974999999999999645 ) ;
#5468=DIRECTION ( 'NONE',  ( 8.018662683283438208E-16, -5.975035461963189015E-16, -1.000000000000000000 ) ) ;
#5469=DIRECTION ( 'NONE',  ( 8.018662683283438208E-16, -5.975035461963189015E-16, -1.000000000000000000 ) ) ;
#5471=EDGE_LOOP ( 'NONE', ( #932, #7215, #928, #2379 ) ) ;
#5472=DIRECTION ( 'NONE',  ( 0.7032868978765922652, 0.7109061395677488404, 1.391731009600549485E-16 ) ) ;
#5473=FACE_OUTER_BOUND ( 'NONE', #2414, .T. ) ;
#5474=VERTEX_POINT ( 'NONE', #10904 ) ;
#5475=ORIENTED_EDGE ( 'NONE', *, *, #1882, .F. ) ;
#5480=VECTOR ( 'NONE', #1844, 1000.000000000000114 ) ;
#5481=ORIENTED_EDGE ( 'NONE', *, *, #11496, .T. ) ;
#5482=DIRECTION ( 'NONE',  ( 0.8018662683283437342, -0.5975035461963190686, 1.000000000000000078E-15 ) ) ;
#5484=ADVANCED_FACE ( 'NONE', ( #7450 ), #432, .F. ) ;
#5490=EDGE_LOOP ( 'NONE', ( #11349, #13780, #10097, #12093 ) ) ;
#5491=LINE ( 'NONE', #7479, #14360 ) ;
#5498=LINE ( 'NONE', #4433, #3969 ) ;
#5499=CARTESIAN_POINT ( 'NONE',  ( -8.561607448813433052, -9.375294326971793879, 57.00231026484399166 ) ) ;
#5501=CARTESIAN_POINT ( 'NONE',  ( -24.38380099443793725, -15.36048369738253427, 56.85231026484398598 ) ) ;
#5502=CARTESIAN_POINT ( 'NONE',  ( -19.38713143869018296, -6.429305403720261936, 56.85231026484398598 ) ) ;
#5505=CARTESIAN_POINT ( 'NONE',  ( -8.972439834930606040, -10.77678811232731348, 56.85231026484400019 ) ) ;
#5506=CARTESIAN_POINT ( 'NONE',  ( -20.94048570341206883, -6.243833066724571168, 56.85231026484398598 ) ) ;
#5508=FACE_OUTER_BOUND ( 'NONE', #968, .T. ) ;
#5510=LINE ( 'NONE', #2078, #2374 ) ;
#5511=DIRECTION ( 'NONE',  ( 8.018662683283438208E-16, -5.975035461963189015E-16, -1.000000000000000000 ) ) ;
#5512=ORIENTED_EDGE ( 'NONE', *, *, #8138, .T. ) ;
#5514=DIRECTION ( 'NONE',  ( 0.5975035461963189576, 0.8018662683283437342, 0.000000000000000000 ) ) ;
#5515=ORIENTED_EDGE ( 'NONE', *, *, #13342, .F. ) ;
#5516=AXIS2_PLACEMENT_3D ( 'NONE', #7151, #3654, #10609 ) ;
#5520=LINE ( 'NONE', #15081, #4774 ) ;
#5521=CARTESIAN_POINT ( 'NONE',  ( -9.299228256956212135, -8.333850033420862502, 56.85231026484398598 ) ) ;
#5527=VERTEX_POINT ( 'NONE', #8747 ) ;
#5531=DIRECTION ( 'NONE',  ( -0.7737441449604661736, -0.6334982226805353500, -2.419218955996689845E-16 ) ) ;
#5538=CARTESIAN_POINT ( 'NONE',  ( -23.36093307149983289, -11.66014798166512634, 56.85231026484398598 ) ) ;
#5540=CARTESIAN_POINT ( 'NONE',  ( -23.39388780995641781, -11.80648316271623877, 57.00231026484397745 ) ) ;
#5541=LINE ( 'NONE', #10363, #8500 ) ;
#5542=ORIENTED_EDGE ( 'NONE', *, *, #3646, .F. ) ;
#5545=FACE_OUTER_BOUND ( 'NONE', #1847, .T. ) ;
#5546=EDGE_LOOP ( 'NONE', ( #6723, #5877, #4678, #5962 ) ) ;
#5547=ORIENTED_EDGE ( 'NONE', *, *, #3271, .T. ) ;
#5549=EDGE_CURVE ( 'NONE', #5733, #8391, #13503, .T. ) ;
#5552=CARTESIAN_POINT ( 'NONE',  ( -6.368730986314239395, -9.491655842995189829, 57.00231026484399166 ) ) ;
#5553=VECTOR ( 'NONE', #11238, 1000.000000000000227 ) ;
#5556=DIRECTION ( 'NONE',  ( -0.1617534816134024167, 0.9868311969055004740, -7.193398003386505973E-16 ) ) ;
#5558=FACE_OUTER_BOUND ( 'NONE', #10411, .T. ) ;
#5559=CARTESIAN_POINT ( 'NONE',  ( -23.05384319539488658, -10.65421522557165623, 56.85231026484398598 ) ) ;
#5560=EDGE_LOOP ( 'NONE', ( #13557, #3905, #6494, #2824 ) ) ;
#5564=EDGE_CURVE ( 'NONE', #9069, #11272, #12058, .T. ) ;
#5567=ORIENTED_EDGE ( 'NONE', *, *, #662, .F. ) ;
#5568=DIRECTION ( 'NONE',  ( 0.5975035461963189576, 0.8018662683283437342, 0.000000000000000000 ) ) ;
#5572=( BOUNDED_CURVE ( )  B_SPLINE_CURVE ( 3, ( #15113, #10604, #12911, #2423 ),
 .UNSPECIFIED., .F., .T. ) 
 B_SPLINE_CURVE_WITH_KNOTS ( ( 4, 4 ),
 ( 1.570796326794895670, 3.141592653589792228 ),
 .UNSPECIFIED. ) 
 CURVE ( )  GEOMETRIC_REPRESENTATION_ITEM ( )  RATIONAL_B_SPLINE_CURVE ( ( 1.000000000000000000, 0.8047378541243649375, 0.8047378541243649375, 1.000000000000000000 ) ) 
 REPRESENTATION_ITEM ( '' )  );
#5577=CARTESIAN_POINT ( 'NONE',  ( -25.44713467170207366, -12.76632185356751847, 57.00231026484397745 ) ) ;
#5578=DIRECTION ( 'NONE',  ( -0.9885168150181794511, 0.1511109077013120805, -8.829475928589259133E-16 ) ) ;
#5582=AXIS2_PLACEMENT_3D ( 'NONE', #3579, #4962, #7159 ) ;
#5584=DIRECTION ( 'NONE',  ( -8.018662683283438208E-16, 5.975035461963189015E-16, 1.000000000000000000 ) ) ;
#5585=ORIENTED_EDGE ( 'NONE', *, *, #8034, .F. ) ;
#5595=VECTOR ( 'NONE', #2390, 1000.000000000000000 ) ;
#5597=ORIENTED_EDGE ( 'NONE', *, *, #5351, .T. ) ;
#5598=DIRECTION ( 'NONE',  ( 0.5975035461963189576, 0.8018662683283437342, 0.000000000000000000 ) ) ;
#5599=EDGE_CURVE ( 'NONE', #4546, #6222, #15021, .T. ) ;
#5602=EDGE_CURVE ( 'NONE', #2901, #5814, #10276, .T. ) ;
#5603=VERTEX_POINT ( 'NONE', #1946 ) ;
#5604=CARTESIAN_POINT ( 'NONE',  ( -23.45327702811275827, -7.487309620431346069, 56.85231026484398598 ) ) ;
#5605=ORIENTED_EDGE ( 'NONE', *, *, #10527, .F. ) ;
#5609=VECTOR ( 'NONE', #6452, 1000.000000000000000 ) ;
#5614=DIRECTION ( 'NONE',  ( -0.6251242923673536733, -0.7805252200231682647, -3.489949670250128540E-17 ) ) ;
#5617=CARTESIAN_POINT ( 'NONE',  ( -23.96284084890188382, -10.23071992935364527, 56.85231026484398598 ) ) ;
#5622=ORIENTED_EDGE ( 'NONE', *, *, #1535, .T. ) ;
#5624=EDGE_CURVE ( 'NONE', #11420, #6835, #4469, .T. ) ;
#5630=LINE ( 'NONE', #2046, #14649 ) ;
#5632=EDGE_CURVE ( 'NONE', #14564, #8987, #6894, .T. ) ;
#5636=ORIENTED_EDGE ( 'NONE', *, *, #14166, .F. ) ;
#5640=CARTESIAN_POINT ( 'NONE',  ( -15.47724068538499154, -13.46270701644446177, 56.85231026484398598 ) ) ;
#5641=EDGE_LOOP ( 'NONE', ( #678, #10792, #5842, #14157 ) ) ;
#5645=LINE ( 'NONE', #10316, #3729 ) ;
#5646=DIRECTION ( 'NONE',  ( 8.018662683283438208E-16, -5.975035461963189015E-16, -1.000000000000000000 ) ) ;
#5647=CARTESIAN_POINT ( 'NONE',  ( -17.20133171717847631, -6.639650181150215325, 57.00231026484397745 ) ) ;
#5652=CARTESIAN_POINT ( 'NONE',  ( -9.401538680480957311, -6.786242167561306715, 56.85231026484398598 ) ) ;
#5654=DIRECTION ( 'NONE',  ( -8.018662683283438208E-16, 5.975035461963189015E-16, 1.000000000000000000 ) ) ;
#5657=ORIENTED_EDGE ( 'NONE', *, *, #13777, .T. ) ;
#5659=ORIENTED_EDGE ( 'NONE', *, *, #7037, .F. ) ;
#5663=FACE_OUTER_BOUND ( 'NONE', #7874, .T. ) ;
#5666=VECTOR ( 'NONE', #451, 1000.000000000000114 ) ;
#5667=PLANE ( 'NONE',  #13436 ) ;
#5668=AXIS2_PLACEMENT_3D ( 'NONE', #3210, #7708, #1837 ) ;
#5669=ADVANCED_FACE ( 'NONE', ( #14795 ), #12586, .F. ) ;
#5672=AXIS2_PLACEMENT_3D ( 'NONE', #1950, #4894, #6301 ) ;
#5674=VECTOR ( 'NONE', #7644, 1000.000000000000000 ) ;
#5677=LINE ( 'NONE', #15013, #12507 ) ;
#5679=DIRECTION ( 'NONE',  ( 8.018662683283438208E-16, -5.975035461963189015E-16, -1.000000000000000000 ) ) ;
#5680=ORIENTED_EDGE ( 'NONE', *, *, #5742, .F. ) ;
#5681=ORIENTED_EDGE ( 'NONE', *, *, #474, .F. ) ;
#5682=CARTESIAN_POINT ( 'NONE',  ( -8.525484111995742964, -7.700351810740323266, 56.85231026484400019 ) ) ;
#5684=LINE ( 'NONE', #10201, #13507 ) ;
#5685=VECTOR ( 'NONE', #3824, 1000.000000000000000 ) ;
#5688=DIRECTION ( 'NONE',  ( 8.018662683283438208E-16, -5.975035461963189015E-16, -1.000000000000000000 ) ) ;
#5692=CARTESIAN_POINT ( 'NONE',  ( -21.23124220554638697, -20.54376104222092181, 57.00231026484397745 ) ) ;
#5695=LINE ( 'NONE', #889, #12903 ) ;
#5696=FACE_OUTER_BOUND ( 'NONE', #4122, .T. ) ;
#5699=ORIENTED_EDGE ( 'NONE', *, *, #10032, .F. ) ;
#5705=ORIENTED_EDGE ( 'NONE', *, *, #6357, .F. ) ;
#5707=EDGE_CURVE ( 'NONE', #10582, #13608, #4926, .T. ) ;
#5709=ADVANCED_FACE ( 'NONE', ( #13044 ), #7123, .T. ) ;
#5710=AXIS2_PLACEMENT_3D ( 'NONE', #4151, #11111, #13141 ) ;
#5711=DIRECTION ( 'NONE',  ( 0.9931883319083343320, -0.1165201156931293391, 8.660254037844386422E-16 ) ) ;
#5713=ORIENTED_EDGE ( 'NONE', *, *, #13693, .F. ) ;
#5716=AXIS2_PLACEMENT_3D ( 'NONE', #13280, #12273, #5151 ) ;
#5718=DIRECTION ( 'NONE',  ( 0.5975035461963189576, 0.8018662683283437342, 0.000000000000000000 ) ) ;
#5719=ORIENTED_EDGE ( 'NONE', *, *, #13379, .T. ) ;
#5720=DIRECTION ( 'NONE',  ( -8.018662683283438208E-16, 5.975035461963189015E-16, 1.000000000000000000 ) ) ;
#5721=ORIENTED_EDGE ( 'NONE', *, *, #117, .F. ) ;
#5722=EDGE_CURVE ( 'NONE', #10422, #1909, #1171, .T. ) ;
#5726=CARTESIAN_POINT ( 'NONE',  ( -23.09568838840838012, -16.24821979201191979, 56.85231026484398598 ) ) ;
#5727=PLANE ( 'NONE',  #6215 ) ;
#5728=DIRECTION ( 'NONE',  ( -8.018662683283438208E-16, 5.975035461963189015E-16, 1.000000000000000000 ) ) ;
#5729=VECTOR ( 'NONE', #12247, 1000.000000000000000 ) ;
#5731=CARTESIAN_POINT ( 'NONE',  ( -17.95685260396765770, -23.17500669507538191, 54.00231026484399166 ) ) ;
#5733=VERTEX_POINT ( 'NONE', #13949 ) ;
#5734=CARTESIAN_POINT ( 'NONE',  ( -8.600581100527527667, -9.311215824554304632, 56.85231026484400019 ) ) ;
#5739=ORIENTED_EDGE ( 'NONE', *, *, #7835, .F. ) ;
#5740=EDGE_CURVE ( 'NONE', #4983, #13470, #9277, .T. ) ;
#5741=EDGE_LOOP ( 'NONE', ( #14458, #7918, #10873, #14995 ) ) ;
#5742=EDGE_CURVE ( 'NONE', #13944, #2941, #13119, .T. ) ;
#5747=LINE ( 'NONE', #9264, #4662 ) ;
#5748=CARTESIAN_POINT ( 'NONE',  ( -14.99866629829804765, -4.445910272123860807, 56.85231026484398598 ) ) ;
#5749=ORIENTED_EDGE ( 'NONE', *, *, #14302, .F. ) ;
#5750=DIRECTION ( 'NONE',  ( 0.5975035461963189576, 0.8018662683283437342, 0.000000000000000000 ) ) ;
#5753=DIRECTION ( 'NONE',  ( 0.5975035461963189576, 0.8018662683283437342, 0.000000000000000000 ) ) ;
#5754=ORIENTED_EDGE ( 'NONE', *, *, #2725, .F. ) ;
#5755=ORIENTED_EDGE ( 'NONE', *, *, #9933, .F. ) ;
#5756=ADVANCED_FACE ( 'NONE', ( #3468 ), #4853, .F. ) ;
#5759=ORIENTED_EDGE ( 'NONE', *, *, #12846, .T. ) ;
#5762=CARTESIAN_POINT ( 'NONE',  ( -19.27841348868324545, -22.73895244004356897, 57.00231026484399166 ) ) ;
#5763=DIRECTION ( 'NONE',  ( -8.018662683283439195E-16, 5.975035461963190001E-16, 1.000000000000000000 ) ) ;
#5765=ORIENTED_EDGE ( 'NONE', *, *, #13391, .T. ) ;
#5767=DIRECTION ( 'NONE',  ( -8.018662683283438208E-16, 5.975035461963189015E-16, 1.000000000000000000 ) ) ;
#5771=EDGE_CURVE ( 'NONE', #5474, #2398, #3776, .T. ) ;
#5773=VECTOR ( 'NONE', #14917, 1000.000000000000000 ) ;
#5774=ORIENTED_EDGE ( 'NONE', *, *, #6613, .F. ) ;
#5776=ORIENTED_EDGE ( 'NONE', *, *, #2574, .T. ) ;
#5777=CARTESIAN_POINT ( 'NONE',  ( -17.81448839017816610, -11.78253482624722537, 51.00231026484399166 ) ) ;
#5778=EDGE_CURVE ( 'NONE', #5017, #2405, #9507, .T. ) ;
#5781=VECTOR ( 'NONE', #235, 1000.000000000000000 ) ;
#5783=ORIENTED_EDGE ( 'NONE', *, *, #14809, .T. ) ;
#5785=CARTESIAN_POINT ( 'NONE',  ( -22.58324314276470091, -9.630648466248954875, 56.85231026484398598 ) ) ;
#5786=DIRECTION ( 'NONE',  ( -0.6061090314442014737, 0.7953815700667020705, -9.612616959383187437E-16 ) ) ;
#5787=VECTOR ( 'NONE', #1470, 1000.000000000000114 ) ;
#5788=EDGE_CURVE ( 'NONE', #3714, #7506, #3698, .T. ) ;
#5789=DIRECTION ( 'NONE',  ( 0.5104125104778984845, 0.8599296884906632021, -1.045284632676530333E-16 ) ) ;
#5790=EDGE_CURVE ( 'NONE', #11735, #10731, #11881, .T. ) ;
#5794=LINE ( 'NONE', #3508, #2256 ) ;
#5798=CARTESIAN_POINT ( 'NONE',  ( -23.68291657637574588, -19.21137664199072148, 57.00231026484397745 ) ) ;
#5799=( LENGTH_UNIT ( ) NAMED_UNIT ( * ) SI_UNIT ( .MILLI., .METRE. ) );
#5802=CARTESIAN_POINT ( 'NONE',  ( -13.57551609484869637, -3.719726473329906025, 54.00231026484399166 ) ) ;
#5807=VECTOR ( 'NONE', #11589, 1000.000000000000000 ) ;
#5811=EDGE_LOOP ( 'NONE', ( #6441, #4693, #9842, #11479 ) ) ;
#5814=VERTEX_POINT ( 'NONE', #14333 ) ;
#5815=FACE_OUTER_BOUND ( 'NONE', #13045, .T. ) ;
#5816=VERTEX_POINT ( 'NONE', #1853 ) ;
#5817=CARTESIAN_POINT ( 'NONE',  ( -15.12053853660593283, -5.441285657357897598, 57.00231026484397745 ) ) ;
#5818=DIRECTION ( 'NONE',  ( 0.8885476655824650072, 0.4587843131450243805, 4.383711467890778149E-16 ) ) ;
#5821=EDGE_CURVE ( 'NONE', #13135, #6106, #9661, .T. ) ;
#5822=DIRECTION ( 'NONE',  ( -0.3956847857120158740, 0.9183863840214728791, 0.000000000000000000 ) ) ;
#5823=DIRECTION ( 'NONE',  ( -8.018662683283438208E-16, 5.975035461963189015E-16, 1.000000000000000000 ) ) ;
#5824=ORIENTED_EDGE ( 'NONE', *, *, #2384, .T. ) ;
#5826=ORIENTED_EDGE ( 'NONE', *, *, #2712, .T. ) ;
#5830=CARTESIAN_POINT ( 'NONE',  ( -20.48903913017556633, -19.85700446605285308, 56.85231026484398598 ) ) ;
#5831=ORIENTED_EDGE ( 'NONE', *, *, #10247, .T. ) ;
#5832=FACE_OUTER_BOUND ( 'NONE', #12140, .T. ) ;
#5834=ADVANCED_FACE ( 'NONE', ( #3925 ), #9953, .T. ) ;
#5840=FACE_OUTER_BOUND ( 'NONE', #10239, .T. ) ;
#5842=ORIENTED_EDGE ( 'NONE', *, *, #7991, .T. ) ;
#5844=VERTEX_POINT ( 'NONE', #14555 ) ;
#5845=DIRECTION ( 'NONE',  ( -8.018662683283438208E-16, 5.975035461963189015E-16, 1.000000000000000000 ) ) ;
#5847=VERTEX_POINT ( 'NONE', #414 ) ;
#5850=EDGE_CURVE ( 'NONE', #13612, #3714, #8580, .T. ) ;
#5855=AXIS2_PLACEMENT_3D ( 'NONE', #4074, #8584, #8811 ) ;
#5856=VERTEX_POINT ( 'NONE', #7585 ) ;
#5858=FACE_OUTER_BOUND ( 'NONE', #13373, .T. ) ;
#5859=ORIENTED_EDGE ( 'NONE', *, *, #14030, .F. ) ;
#5860=PLANE ( 'NONE',  #9983 ) ;
#5861=VERTEX_POINT ( 'NONE', #12111 ) ;
#5863=ORIENTED_EDGE ( 'NONE', *, *, #9359, .F. ) ;
#5864=LINE ( 'NONE', #8010, #12285 ) ;
#5866=DIRECTION ( 'NONE',  ( 0.9826409426582659590, -0.1855175943453191700, 8.987940462991681405E-16 ) ) ;
#5869=DIRECTION ( 'NONE',  ( -8.018662683283439195E-16, 5.975035461963190001E-16, 1.000000000000000000 ) ) ;
#5871=CARTESIAN_POINT ( 'NONE',  ( -7.594860258898399330, -10.18326093375929631, 56.85231026484400019 ) ) ;
#5872=ADVANCED_FACE ( 'NONE', ( #14407 ), #489, .F. ) ;
#5875=AXIS2_PLACEMENT_3D ( 'NONE', #6360, #640, #11267 ) ;
#5876=DIRECTION ( 'NONE',  ( 0.5975035461963189576, 0.8018662683283437342, 0.000000000000000000 ) ) ;
#5877=ORIENTED_EDGE ( 'NONE', *, *, #8872, .T. ) ;
#5881=EDGE_LOOP ( 'NONE', ( #2602, #485, #4528, #11008, #11483, #11337 ) ) ;
#5883=VERTEX_POINT ( 'NONE', #14628 ) ;
#5886=DIRECTION ( 'NONE',  ( 0.3857661296576204712, 0.9225966037272086417, -2.419218955996629202E-16 ) ) ;
#5890=( NAMED_UNIT ( * ) PLANE_ANGLE_UNIT ( ) SI_UNIT ( $, .RADIAN. ) );
#5893=CARTESIAN_POINT ( 'NONE',  ( -24.32830346761242879, -18.15026423267100597, 54.00231026484399166 ) ) ;
#5894=DIRECTION ( 'NONE',  ( -8.018662683283438208E-16, 5.975035461963189015E-16, 1.000000000000000000 ) ) ;
#5895=AXIS2_PLACEMENT_3D ( 'NONE', #12336, #1778, #5076 ) ;
#5896=ORIENTED_EDGE ( 'NONE', *, *, #10858, .F. ) ;
#5897=FACE_OUTER_BOUND ( 'NONE', #14025, .T. ) ;
#5898=ORIENTED_EDGE ( 'NONE', *, *, #6711, .F. ) ;
#5901=AXIS2_PLACEMENT_3D ( 'NONE', #13337, #7347, #13262 ) ;
#5905=EDGE_CURVE ( 'NONE', #9600, #1021, #12039, .T. ) ;
#5906=FACE_OUTER_BOUND ( 'NONE', #2237, .T. ) ;
#5907=VECTOR ( 'NONE', #14665, 1000.000000000000227 ) ;
#5916=DIRECTION ( 'NONE',  ( 0.5975035461963189576, 0.8018662683283437342, 0.000000000000000000 ) ) ;
#5922=ORIENTED_EDGE ( 'NONE', *, *, #8588, .F. ) ;
#5925=VERTEX_POINT ( 'NONE', #5144 ) ;
#5928=DIRECTION ( 'NONE',  ( 0.5975035461963189576, 0.8018662683283437342, 0.000000000000000000 ) ) ;
#5930=AXIS2_PLACEMENT_3D ( 'NONE', #10488, #14998, #931 ) ;
#5933=ORIENTED_EDGE ( 'NONE', *, *, #12891, .T. ) ;
#5935=CARTESIAN_POINT ( 'NONE',  ( -23.12048770254168062, -16.17743848078839619, 56.85231026484398598 ) ) ;
#5937=CARTESIAN_POINT ( 'NONE',  ( -20.52642601085533869, -22.12321610861327770, 54.00231026484399166 ) ) ;
#5938=ORIENTED_EDGE ( 'NONE', *, *, #14024, .T. ) ;
#5939=CARTESIAN_POINT ( 'NONE',  ( -10.08476707729037614, -21.88467736064467672, 57.00231026484399166 ) ) ;
#5940=ORIENTED_EDGE ( 'NONE', *, *, #3387, .T. ) ;
#5941=CARTESIAN_POINT ( 'NONE',  ( -13.41639018438039699, -15.05973874201012741, 51.00231026484399166 ) ) ;
#5945=DIRECTION ( 'NONE',  ( -0.4491835085186243748, -0.8934395198752397294, 1.736481776669299976E-16 ) ) ;
#5946=DIRECTION ( 'NONE',  ( 0.8222303661035966771, -0.5691548339926011391, 9.993908270190953088E-16 ) ) ;
#5947=AXIS2_PLACEMENT_3D ( 'NONE', #2510, #3808, #11758 ) ;
#5953=ORIENTED_EDGE ( 'NONE', *, *, #3986, .T. ) ;
#5955=DIRECTION ( 'NONE',  ( -0.5401126942952620968, -0.8415927028326188886, 6.975647374412522208E-17 ) ) ;
#5959=DIRECTION ( 'NONE',  ( -0.4177292884839868270, -0.9085715390340278752, 2.079116908177700458E-16 ) ) ;
#5960=VERTEX_POINT ( 'NONE', #1701 ) ;
#5961=DIRECTION ( 'NONE',  ( -8.018662683283438208E-16, 5.975035461963189015E-16, 1.000000000000000000 ) ) ;
#5962=ORIENTED_EDGE ( 'NONE', *, *, #2963, .F. ) ;
#5965=CARTESIAN_POINT ( 'NONE',  ( -12.04767799572592502, -20.80732214584531548, 56.85231026484400019 ) ) ;
#5966=ORIENTED_EDGE ( 'NONE', *, *, #13391, .F. ) ;
#5968=CARTESIAN_POINT ( 'NONE',  ( -16.32149003149046607, -5.473954385499126829, 56.85231026484398598 ) ) ;
#5969=ADVANCED_FACE ( 'NONE', ( #5663 ), #10334, .F. ) ;
#5970=CARTESIAN_POINT ( 'NONE',  ( -14.00164528647249007, -5.572553380472728968, 56.85231026484398598 ) ) ;
#5975=CARTESIAN_POINT ( 'NONE',  ( -18.26066734922995494, -14.69693585872053632, 57.00231026484398456 ) ) ;
#5979=ORIENTED_EDGE ( 'NONE', *, *, #5228, .T. ) ;
#5981=VERTEX_POINT ( 'NONE', #2160 ) ;
#5982=AXIS2_PLACEMENT_3D ( 'NONE', #14170, #2538, #14087 ) ;
#5983=EDGE_CURVE ( 'NONE', #5192, #5306, #2634, .T. ) ;
#5984=DIRECTION ( 'NONE',  ( -0.1272150336605082366, 0.9918751611018171710, -6.946583704589972670E-16 ) ) ;
#5985=EDGE_CURVE ( 'NONE', #1451, #9234, #1409, .T. ) ;
#5988=DIRECTION ( 'NONE',  ( -0.09252159378507134047, 0.9957106782009873536, -6.691306063588577540E-16 ) ) ;
#5991=CARTESIAN_POINT ( 'NONE',  ( -22.64031343690345111, -17.27870339600297811, 57.00231026484397745 ) ) ;
#5996=ORIENTED_EDGE ( 'NONE', *, *, #4675, .T. ) ;
#5997=CARTESIAN_POINT ( 'NONE',  ( -21.68801466096620700, -19.44379288755867208, 57.00231026484397745 ) ) ;
#6000=CARTESIAN_POINT ( 'NONE',  ( -24.55043086433169819, -12.83990741858047357, 56.85231026484398598 ) ) ;
#6002=AXIS2_PLACEMENT_3D ( 'NONE', #10302, #4801, #4883 ) ;
#6004=EDGE_CURVE ( 'NONE', #11664, #10889, #9719, .T. ) ;
#6005=CARTESIAN_POINT ( 'NONE',  ( -23.02734322232803521, -10.58405290357860373, 57.00231026484397745 ) ) ;
#6007=VERTEX_POINT ( 'NONE', #11486 ) ;
#6009=LINE ( 'NONE', #8465, #8229 ) ;
#6010=VERTEX_POINT ( 'NONE', #13787 ) ;
#6011=LINE ( 'NONE', #9619, #7375 ) ;
#6012=ORIENTED_EDGE ( 'NONE', *, *, #936, .T. ) ;
#6014=ORIENTED_EDGE ( 'NONE', *, *, #11526, .F. ) ;
#6017=CARTESIAN_POINT ( 'NONE',  ( -15.10625462230756177, -3.540141368888813922, 56.85231026484398598 ) ) ;
#6022=VERTEX_POINT ( 'NONE', #4378 ) ;
#6023=DIRECTION ( 'NONE',  ( 8.018662683283438208E-16, -5.975035461963189015E-16, -1.000000000000000000 ) ) ;
#6027=CARTESIAN_POINT ( 'NONE',  ( -13.57551609484869815, -3.719726473329904248, 56.85231026484398598 ) ) ;
#6028=ORIENTED_EDGE ( 'NONE', *, *, #15077, .F. ) ;
#6029=VECTOR ( 'NONE', #1580, 1000.000000000000000 ) ;
#6031=ORIENTED_EDGE ( 'NONE', *, *, #9382, .T. ) ;
#6032=EDGE_LOOP ( 'NONE', ( #4463, #8968, #14331, #3146 ) ) ;
#6033=FACE_OUTER_BOUND ( 'NONE', #3777, .T. ) ;
#6035=CARTESIAN_POINT ( 'NONE',  ( -14.00594099532011860, -11.50271332161736915, 51.25231026484399166 ) ) ;
#6038=DIRECTION ( 'NONE',  ( 0.3204693369899919708, 0.9472588896649083434, -3.090169943749469383E-16 ) ) ;
#6040=( NAMED_UNIT ( * ) SI_UNIT ( $, .STERADIAN. ) SOLID_ANGLE_UNIT ( ) );
#6044=AXIS2_PLACEMENT_3D ( 'NONE', #3765, #3535, #7193 ) ;
#6045=FACE_OUTER_BOUND ( 'NONE', #10448, .T. ) ;
#6049=EDGE_LOOP ( 'NONE', ( #11044, #5093, #7776, #13991 ) ) ;
#6051=CARTESIAN_POINT ( 'NONE',  ( -20.39403028972282428, -7.084672814149619136, 57.00231026484397745 ) ) ;
#6054=LINE ( 'NONE', #1482, #10040 ) ;
#6055=DIRECTION ( 'NONE',  ( -0.7805252200231683757, 0.6251242923673537843, -9.993908270190959005E-16 ) ) ;
#6057=EDGE_CURVE ( 'NONE', #4202, #6280, #11186, .T. ) ;
#6058=CYLINDRICAL_SURFACE ( 'NONE', #11985, 9.974999999999997868 ) ;
#6059=CARTESIAN_POINT ( 'NONE',  ( -6.507973901336479017, -12.27851192488648024, 56.85231026484400019 ) ) ;
#6062=DIRECTION ( 'NONE',  ( 0.5975035461963188466, 0.8018662683283437342, 0.000000000000000000 ) ) ;
#6064=DIRECTION ( 'NONE',  ( 0.7582332219680881780, -0.6519834208811539078, 9.975640502598240034E-16 ) ) ;
#6065=ORIENTED_EDGE ( 'NONE', *, *, #8421, .F. ) ;
#6069=ORIENTED_EDGE ( 'NONE', *, *, #5012, .T. ) ;
#6071=DIRECTION ( 'NONE',  ( 8.018662683283438208E-16, -5.975035461963189015E-16, -1.000000000000000000 ) ) ;
#6075=ADVANCED_FACE ( 'NONE', ( #4298 ), #13632, .T. ) ;
#6078=EDGE_CURVE ( 'NONE', #2929, #11933, #6653, .T. ) ;
#6079=VECTOR ( 'NONE', #10413, 1000.000000000000000 ) ;
#6084=CARTESIAN_POINT ( 'NONE',  ( -9.401538680480957311, -6.786242167561306715, 57.00231026484397745 ) ) ;
#6085=PLANE ( 'NONE',  #10679 ) ;
#6086=ORIENTED_EDGE ( 'NONE', *, *, #1688, .F. ) ;
#6089=ORIENTED_EDGE ( 'NONE', *, *, #8226, .F. ) ;
#6090=DIRECTION ( 'NONE',  ( -8.018662683283439195E-16, 5.975035461963190001E-16, 1.000000000000000000 ) ) ;
#6095=DIRECTION ( 'NONE',  ( -8.018662683283438208E-16, 5.975035461963189015E-16, 1.000000000000000000 ) ) ;
#6097=DIRECTION ( 'NONE',  ( -0.3204693369899910826, -0.9472588896649086765, 3.090169943749478258E-16 ) ) ;
#6099=LINE ( 'NONE', #13089, #8476 ) ;
#6101=FACE_OUTER_BOUND ( 'NONE', #10524, .T. ) ;
#6104=ORIENTED_EDGE ( 'NONE', *, *, #4578, .T. ) ;
#6105=CARTESIAN_POINT ( 'NONE',  ( -24.88854884048805616, -16.87637585156647546, 54.00231026484397745 ) ) ;
#6106=VERTEX_POINT ( 'NONE', #8261 ) ;
#6107=ORIENTED_EDGE ( 'NONE', *, *, #9731, .F. ) ;
#6108=VECTOR ( 'NONE', #9726, 999.9999999999998863 ) ;
#6109=PLANE ( 'NONE',  #4706 ) ;
#6111=DIRECTION ( 'NONE',  ( 0.5975035461963189576, 0.8018662683283437342, 0.000000000000000000 ) ) ;
#6113=PLANE ( 'NONE',  #13087 ) ;
#6114=CARTESIAN_POINT ( 'NONE',  ( -15.49969986081092088, -13.50737899243822504, 56.85231026484398598 ) ) ;
#6116=CARTESIAN_POINT ( 'NONE',  ( -7.499849062438288527, -12.40572695854698360, 57.00231026484399166 ) ) ;
#6123=EDGE_LOOP ( 'NONE', ( #10353, #15079, #5863, #14811 ) ) ;
#6127=VECTOR ( 'NONE', #1404, 1000.000000000000000 ) ;
#6128=LINE ( 'NONE', #8438, #323 ) ;
#6130=ADVANCED_FACE ( 'NONE', ( #5815 ), #11562, .F. ) ;
#6131=DIRECTION ( 'NONE',  ( 8.018662683283438208E-16, -5.975035461963189015E-16, -1.000000000000000000 ) ) ;
#6132=PLANE ( 'NONE',  #7286 ) ;
#6134=AXIS2_PLACEMENT_3D ( 'NONE', #395, #10788, #6256 ) ;
#6137=CARTESIAN_POINT ( 'NONE',  ( -7.887638505697306179, -19.95386229157006497, 56.85231026484400019 ) ) ;
#6138=ORIENTED_EDGE ( 'NONE', *, *, #12527, .F. ) ;
#6139=DIRECTION ( 'NONE',  ( -0.04695496274984587576, -0.9988970074402868660, 5.591929034707467802E-16 ) ) ;
#6140=CYLINDRICAL_SURFACE ( 'NONE', #8687, 0.2499999999999996947 ) ;
#6142=EDGE_LOOP ( 'NONE', ( #14512, #2401, #14405, #204 ) ) ;
#6144=CARTESIAN_POINT ( 'NONE',  ( -6.424455519809837867, -13.54187755947681993, 57.00231026484399166 ) ) ;
#6146=LINE ( 'NONE', #5370, #10856 ) ;
#6149=ADVANCED_FACE ( 'NONE', ( #8104 ), #2310, .T. ) ;
#6153=CIRCLE ( 'NONE', #8608, 9.974999999999999645 ) ;
#6154=EDGE_CURVE ( 'NONE', #3452, #13092, #12652, .T. ) ;
#6157=EDGE_CURVE ( 'NONE', #6428, #4722, #9335, .T. ) ;
#6159=LINE ( 'NONE', #13301, #3500 ) ;
#6160=ORIENTED_EDGE ( 'NONE', *, *, #3386, .F. ) ;
#6161=LINE ( 'NONE', #1275, #10925 ) ;
#6162=AXIS2_PLACEMENT_3D ( 'NONE', #119, #9435, #9666 ) ;
#6164=ORIENTED_EDGE ( 'NONE', *, *, #11866, .T. ) ;
#6165=AXIS2_PLACEMENT_3D ( 'NONE', #6716, #5578, #14994 ) ;
#6168=EDGE_LOOP ( 'NONE', ( #3601, #825, #4166, #1830 ) ) ;
#6171=DIRECTION ( 'NONE',  ( 8.018662683283438208E-16, -5.975035461963189015E-16, -1.000000000000000000 ) ) ;
#6172=EDGE_CURVE ( 'NONE', #186, #11757, #14242, .T. ) ;
#6174=PLANE ( 'NONE',  #14543 ) ;
#6176=VECTOR ( 'NONE', #3066, 1000.000000000000227 ) ;
#6183=ORIENTED_EDGE ( 'NONE', *, *, #6592, .F. ) ;
#6185=EDGE_LOOP ( 'NONE', ( #9951, #2552, #14626, #14096 ) ) ;
#6186=CARTESIAN_POINT ( 'NONE',  ( -15.45378054160984682, -13.48759475315262613, 56.85231026484398598 ) ) ;
#6187=ORIENTED_EDGE ( 'NONE', *, *, #10998, .F. ) ;
#6188=ORIENTED_EDGE ( 'NONE', *, *, #7905, .F. ) ;
#6189=VECTOR ( 'NONE', #9161, 1000.000000000000114 ) ;
#6190=DIRECTION ( 'NONE',  ( -8.018662683283438208E-16, 5.975035461963189015E-16, 1.000000000000000000 ) ) ;
#6191=ORIENTED_EDGE ( 'NONE', *, *, #11136, .T. ) ;
#6193=AXIS2_PLACEMENT_3D ( 'NONE', #8681, #4252, #9979 ) ;
#6194=CARTESIAN_POINT ( 'NONE',  ( -23.41792317787242084, -15.09084496969942535, 57.00231026484397745 ) ) ;
#6196=DIRECTION ( 'NONE',  ( 0.4274949678123838859, -0.9040177279761104634, 8.829475928589268008E-16 ) ) ;
#6197=AXIS2_PLACEMENT_3D ( 'NONE', #11825, #12987, #1350 ) ;
#6199=ADVANCED_FACE ( 'NONE', ( #9492 ), #8184, .F. ) ;
#6200=CARTESIAN_POINT ( 'NONE',  ( -8.744338604334316756, -15.61126689213601360, 57.00231026484399166 ) ) ;
#6202=ORIENTED_EDGE ( 'NONE', *, *, #7898, .F. ) ;
#6203=DIRECTION ( 'NONE',  ( -8.018662683283438208E-16, 5.975035461963189015E-16, 1.000000000000000000 ) ) ;
#6204=VERTEX_POINT ( 'NONE', #7026 ) ;
#6205=VERTEX_POINT ( 'NONE', #8339 ) ;
#6206=DIRECTION ( 'NONE',  ( 8.018662683283438208E-16, -5.975035461963189015E-16, -1.000000000000000000 ) ) ;
#6210=CYLINDRICAL_SURFACE ( 'NONE', #966, 0.2500000000000004441 ) ;
#6211=AXIS2_PLACEMENT_3D ( 'NONE', #11081, #604, #9152 ) ;
#6214=CARTESIAN_POINT ( 'NONE',  ( -15.45180655762527699, -13.52173975529984418, 56.85231026484398598 ) ) ;
#6215=AXIS2_PLACEMENT_3D ( 'NONE', #8086, #78, #1069 ) ;
#6221=LINE ( 'NONE', #8448, #9363 ) ;
#6222=VERTEX_POINT ( 'NONE', #4914 ) ;
#6225=ORIENTED_EDGE ( 'NONE', *, *, #14828, .F. ) ;
#6227=DIRECTION ( 'NONE',  ( -0.3306575217771102193, 0.9437508163134058492, -8.290375725550400094E-16 ) ) ;
#6229=EDGE_CURVE ( 'NONE', #1960, #11221, #94, .T. ) ;
#6232=CARTESIAN_POINT ( 'NONE',  ( -21.67659902633306146, -21.33978230808610022, 57.00231026484397745 ) ) ;
#6233=VERTEX_POINT ( 'NONE', #4756 ) ;
#6234=ADVANCED_FACE ( 'NONE', ( #2231 ), #6876, .F. ) ;
#6236=DIRECTION ( 'NONE',  ( 0.9183863840214729901, 0.3956847857120157075, 4.999999999999999402E-16 ) ) ;
#6242=FACE_OUTER_BOUND ( 'NONE', #12330, .T. ) ;
#6244=LINE ( 'NONE', #602, #8221 ) ;
#6245=AXIS2_PLACEMENT_3D ( 'NONE', #13551, #13774, #11396 ) ;
#6249=DIRECTION ( 'NONE',  ( -8.018662683283438208E-16, 5.975035461963189015E-16, 1.000000000000000000 ) ) ;
#6250=VERTEX_POINT ( 'NONE', #15044 ) ;
#6252=EDGE_CURVE ( 'NONE', #9932, #9450, #9454, .T. ) ;
#6253=LINE ( 'NONE', #464, #6526 ) ;
#6256=DIRECTION ( 'NONE',  ( 8.018662683283438208E-16, -5.975035461963189015E-16, -1.000000000000000000 ) ) ;
#6257=ORIENTED_EDGE ( 'NONE', *, *, #8260, .T. ) ;
#6260=ORIENTED_EDGE ( 'NONE', *, *, #8377, .F. ) ;
#6265=LINE ( 'NONE', #3985, #5729 ) ;
#6268=LINE ( 'NONE', #11096, #10417 ) ;
#6272=EDGE_CURVE ( 'NONE', #12486, #7429, #7067, .T. ) ;
#6273=EDGE_CURVE ( 'NONE', #10559, #7319, #3420, .T. ) ;
#6277=ORIENTED_EDGE ( 'NONE', *, *, #4317, .T. ) ;
#6279=CARTESIAN_POINT ( 'NONE',  ( -23.54151295824578227, -12.77219731018227300, 56.85231026484398598 ) ) ;
#6280=VERTEX_POINT ( 'NONE', #6990 ) ;
#6283=DIRECTION ( 'NONE',  ( 0.5975035461963189576, 0.8018662683283437342, 0.000000000000000000 ) ) ;
#6286=CARTESIAN_POINT ( 'NONE',  ( -21.48581293389291247, -5.528213918555015205, 57.00231026484397745 ) ) ;
#6287=CIRCLE ( 'NONE', #14841, 9.974999999999999645 ) ;
#6288=VECTOR ( 'NONE', #10825, 1000.000000000000000 ) ;
#6290=CARTESIAN_POINT ( 'NONE',  ( -22.61924992783766797, -9.696439889920343447, 57.00231026484397745 ) ) ;
#6291=CARTESIAN_POINT ( 'NONE',  ( -12.52039621090187893, -4.935039769003430443, 56.85231026484398598 ) ) ;
#6292=DIRECTION ( 'NONE',  ( -0.9755678736739584744, 0.2196982563774038943, -9.135454576426008610E-16 ) ) ;
#6294=EDGE_LOOP ( 'NONE', ( #14572, #8163, #10345, #2664 ) ) ;
#6295=LINE ( 'NONE', #4163, #12662 ) ;
#6297=ORIENTED_EDGE ( 'NONE', *, *, #7383, .F. ) ;
#6298=ORIENTED_EDGE ( 'NONE', *, *, #15072, .F. ) ;
#6300=VERTEX_POINT ( 'NONE', #4880 ) ;
#6301=DIRECTION ( 'NONE',  ( 0.9931883319083342210, -0.1165201156931306992, 0.000000000000000000 ) ) ;
#6302=CIRCLE ( 'NONE', #9494, 9.974999999999999645 ) ;
#6303=ADVANCED_FACE ( 'NONE', ( #14203 ), #12684, .F. ) ;
#6304=CARTESIAN_POINT ( 'NONE',  ( -7.490307934913750465, -12.48011759562962020, 57.00231026484399166 ) ) ;
#6308=DIRECTION ( 'NONE',  ( 8.018662683283438208E-16, -5.975035461963189015E-16, -1.000000000000000000 ) ) ;
#6309=EDGE_LOOP ( 'NONE', ( #9981, #10442, #5061, #13266 ) ) ;
#6310=CARTESIAN_POINT ( 'NONE',  ( -18.18846581869429713, -17.11577719991581148, -13.99768973515600301 ) ) ;
#6311=DIRECTION ( 'NONE',  ( -8.018662683283438208E-16, 5.975035461963189015E-16, 1.000000000000000000 ) ) ;
#6312=ORIENTED_EDGE ( 'NONE', *, *, #12158, .F. ) ;
#6314=CARTESIAN_POINT ( 'NONE',  ( -15.45378054160984682, -13.48759475315262613, 56.85231026484398598 ) ) ;
#6316=FACE_OUTER_BOUND ( 'NONE', #10947, .T. ) ;
#6317=EDGE_LOOP ( 'NONE', ( #4616, #3145, #9353, #3499 ) ) ;
#6318=CARTESIAN_POINT ( 'NONE',  ( -15.49969986081091733, -13.50737899243822682, 54.00231026484399166 ) ) ;
#6320=EDGE_CURVE ( 'NONE', #9709, #6890, #12990, .T. ) ;
#6321=DIRECTION ( 'NONE',  ( 0.5975035461963189576, 0.8018662683283437342, 0.000000000000000000 ) ) ;
#6324=ADVANCED_FACE ( 'NONE', ( #3723 ), #2279, .F. ) ;
#6327=DIRECTION ( 'NONE',  ( -8.018662683283438208E-16, 5.975035461963189015E-16, 1.000000000000000000 ) ) ;
#6328=ORIENTED_EDGE ( 'NONE', *, *, #11666, .T. ) ;
#6332=ORIENTED_EDGE ( 'NONE', *, *, #9174, .T. ) ;
#6335=ORIENTED_EDGE ( 'NONE', *, *, #2986, .F. ) ;
#6336=ORIENTED_EDGE ( 'NONE', *, *, #1315, .F. ) ;
#6337=CIRCLE ( 'NONE', #8786, 9.974999999999999645 ) ;
#6338=DIRECTION ( 'NONE',  ( 0.5779813897169902015, -0.8160499452489515804, 9.510565162951535624E-16 ) ) ;
#6344=LINE ( 'NONE', #2766, #8064 ) ;
#6345=CARTESIAN_POINT ( 'NONE',  ( -21.24026693782044717, -7.828337292084670551, 56.85231026484398598 ) ) ;
#6347=PLANE ( 'NONE',  #14245 ) ;
#6348=VERTEX_POINT ( 'NONE', #12210 ) ;
#6350=EDGE_LOOP ( 'NONE', ( #4105, #6365, #1381, #10719 ) ) ;
#6352=ORIENTED_EDGE ( 'NONE', *, *, #13124, .F. ) ;
#6356=CARTESIAN_POINT ( 'NONE',  ( -8.663330333365388825, -17.80566954616001496, 57.00231026484399166 ) ) ;
#6357=EDGE_CURVE ( 'NONE', #11198, #12259, #369, .T. ) ;
#6358=DIRECTION ( 'NONE',  ( -0.5779813897169993053, 0.8160499452489450301, -9.510565162951571123E-16 ) ) ;
#6360=CARTESIAN_POINT ( 'NONE',  ( -24.33650094517379614, -11.44044972528773130, 56.85231026484398598 ) ) ;
#6361=DIRECTION ( 'NONE',  ( -8.018662683283438208E-16, 5.975035461963189015E-16, 1.000000000000000000 ) ) ;
#6364=DIRECTION ( 'NONE',  ( 0.5975035461963189576, 0.8018662683283437342, 0.000000000000000000 ) ) ;
#6365=ORIENTED_EDGE ( 'NONE', *, *, #12435, .F. ) ;
#6367=VECTOR ( 'NONE', #13425, 1000.000000000000000 ) ;
#6371=LINE ( 'NONE', #1646, #12785 ) ;
#6374=CIRCLE ( 'NONE', #12760, 9.974999999999999645 ) ;
#6375=DIRECTION ( 'NONE',  ( -8.018662683283438208E-16, 5.975035461963189015E-16, 1.000000000000000000 ) ) ;
#6378=LINE ( 'NONE', #10128, #11811 ) ;
#6379=ORIENTED_EDGE ( 'NONE', *, *, #9908, .T. ) ;
#6381=CARTESIAN_POINT ( 'NONE',  ( -19.62128088291994388, -20.45131122700032833, 56.85231026484398598 ) ) ;
#6383=ORIENTED_EDGE ( 'NONE', *, *, #4928, .T. ) ;
#6384=EDGE_CURVE ( 'NONE', #4372, #5367, #5167, .T. ) ;
#6386=CARTESIAN_POINT ( 'NONE',  ( -23.54764701038621411, -12.84694604531765272, 57.00231026484397745 ) ) ;
#6389=LINE ( 'NONE', #12373, #4739 ) ;
#6391=AXIS2_PLACEMENT_3D ( 'NONE', #13172, #4338, #7249 ) ;
#6393=AXIS2_PLACEMENT_3D ( 'NONE', #11169, #1988, #5353 ) ;
#6397=CIRCLE ( 'NONE', #9800, 9.974999999999999645 ) ;
#6398=AXIS2_PLACEMENT_3D ( 'NONE', #11719, #4766, #14253 ) ;
#6399=CARTESIAN_POINT ( 'NONE',  ( -9.565488148413143321, -20.37370125056455095, 56.85231026484400019 ) ) ;
#6400=PLANE ( 'NONE',  #6211 ) ;
#6402=CARTESIAN_POINT ( 'NONE',  ( -15.49969986081092088, -13.50737899243822504, 56.85231026484398598 ) ) ;
#6405=ORIENTED_EDGE ( 'NONE', *, *, #7655, .F. ) ;
#6412=CONICAL_SURFACE ( 'NONE', #7881, 4.499999999999999112, 0.7853981633974476129 ) ;
#6417=LINE ( 'NONE', #1841, #1177 ) ;
#6420=CARTESIAN_POINT ( 'NONE',  ( -7.480766807389218620, -12.55450823271226746, 56.85231026484400019 ) ) ;
#6422=ORIENTED_EDGE ( 'NONE', *, *, #13277, .F. ) ;
#6424=ORIENTED_EDGE ( 'NONE', *, *, #10546, .F. ) ;
#6427=VERTEX_POINT ( 'NONE', #13220 ) ;
#6428=VERTEX_POINT ( 'NONE', #4953 ) ;
#6431=LINE ( 'NONE', #14629, #13541 ) ;
#6435=CIRCLE ( 'NONE', #8649, 9.974999999999999645 ) ;
#6436=PLANE ( 'NONE',  #4414 ) ;
#6438=CARTESIAN_POINT ( 'NONE',  ( -23.14528701667493849, -16.10665716956490812, 56.85231026484398598 ) ) ;
#6440=EDGE_CURVE ( 'NONE', #2941, #9718, #2724, .T. ) ;
#6441=ORIENTED_EDGE ( 'NONE', *, *, #4767, .T. ) ;
#6443=EDGE_CURVE ( 'NONE', #8706, #2715, #9213, .T. ) ;
#6445=ORIENTED_EDGE ( 'NONE', *, *, #11168, .T. ) ;
#6446=VERTEX_POINT ( 'NONE', #7819 ) ;
#6447=VECTOR ( 'NONE', #3573, 999.9999999999998863 ) ;
#6449=ORIENTED_EDGE ( 'NONE', *, *, #3300, .T. ) ;
#6452=DIRECTION ( 'NONE',  ( 0.1165201156931293391, 0.9931883319083343320, -4.999999999999998416E-16 ) ) ;
#6454=CARTESIAN_POINT ( 'NONE',  ( -15.50552586659557797, -13.55703840903364288, 56.85231026484398598 ) ) ;
#6457=VERTEX_POINT ( 'NONE', #1807 ) ;
#6460=CARTESIAN_POINT ( 'NONE',  ( -15.31527533914055539, -21.58027268651140673, 56.85231026484400019 ) ) ;
#6461=ORIENTED_EDGE ( 'NONE', *, *, #10640, .T. ) ;
#6463=PLANE ( 'NONE',  #2293 ) ;
#6465=LINE ( 'NONE', #12452, #2960 ) ;
#6466=VECTOR ( 'NONE', #13102, 1000.000000000000000 ) ;
#6467=CARTESIAN_POINT ( 'NONE',  ( -19.87664613915258371, -5.557310358991672139, 56.85231026484398598 ) ) ;
#6468=ADVANCED_FACE ( 'NONE', ( #7680 ), #13442, .T. ) ;
#6469=CARTESIAN_POINT ( 'NONE',  ( -7.821737630532772378, -18.34578224045527151, 57.00231026484399166 ) ) ;
#6470=CARTESIAN_POINT ( 'NONE',  ( -9.204203523554131294, -8.449911655164932256, 57.00231026484397745 ) ) ;
#6471=LINE ( 'NONE', #13607, #10360 ) ;
#6474=VECTOR ( 'NONE', #2124, 1000.000000000000000 ) ;
#6478=VERTEX_POINT ( 'NONE', #5538 ) ;
#6480=DIRECTION ( 'NONE',  ( -8.018662683283438208E-16, 5.975035461963189015E-16, 1.000000000000000000 ) ) ;
#6481=CARTESIAN_POINT ( 'NONE',  ( -17.54761070396351741, -21.31837676343380750, 57.00231026484399166 ) ) ;
#6482=CARTESIAN_POINT ( 'NONE',  ( -18.36422177163696290, -5.957162821864243618, 56.85231026484398598 ) ) ;
#6483=CYLINDRICAL_SURFACE ( 'NONE', #12090, 9.974999999999997868 ) ;
#6485=EDGE_CURVE ( 'NONE', #6873, #9624, #12436, .T. ) ;
#6492=FACE_OUTER_BOUND ( 'NONE', #12601, .T. ) ;
#6494=ORIENTED_EDGE ( 'NONE', *, *, #5114, .F. ) ;
#6499=CARTESIAN_POINT ( 'NONE',  ( -13.08902965115471417, -15.30366854329086834, 57.00231026484398456 ) ) ;
#6506=CARTESIAN_POINT ( 'NONE',  ( -10.07958688850791162, -7.521259601090221736, 56.85231026484398598 ) ) ;
#6511=CARTESIAN_POINT ( 'NONE',  ( -12.98295438134161195, -5.834228258119843247, 56.85231026484398598 ) ) ;
#6514=LINE ( 'NONE', #14719, #157 ) ;
#6516=ORIENTED_EDGE ( 'NONE', *, *, #11975, .T. ) ;
#6518=ORIENTED_EDGE ( 'NONE', *, *, #5564, .F. ) ;
#6519=LINE ( 'NONE', #1719, #1291 ) ;
#6524=EDGE_CURVE ( 'NONE', #10845, #13725, #5389, .T. ) ;
#6526=VECTOR ( 'NONE', #9787, 1000.000000000000000 ) ;
#6532=EDGE_LOOP ( 'NONE', ( #7430, #13504, #9116, #1329 ) ) ;
#6533=LINE ( 'NONE', #8760, #1158 ) ;
#6535=ORIENTED_EDGE ( 'NONE', *, *, #4328, .T. ) ;
#6536=EDGE_CURVE ( 'NONE', #11708, #11163, #8754, .T. ) ;
#6539=DIRECTION ( 'NONE',  ( -0.9437508163134049610, -0.3306575217771128283, -5.591929034707468788E-16 ) ) ;
#6544=EDGE_CURVE ( 'NONE', #2885, #6427, #13587, .T. ) ;
#6555=DIRECTION ( 'NONE',  ( -0.7737441449604661736, -0.6334982226805353500, -2.419218955996689845E-16 ) ) ;
#6557=ORIENTED_EDGE ( 'NONE', *, *, #2517, .F. ) ;
#6558=EDGE_CURVE ( 'NONE', #2908, #14123, #5319, .T. ) ;
#6564=CARTESIAN_POINT ( 'NONE',  ( -16.49725497239786165, -3.582384846377125509, 54.00231026484397745 ) ) ;
#6566=DIRECTION ( 'NONE',  ( -8.018662683283438208E-16, 5.975035461963189015E-16, 1.000000000000000000 ) ) ;
#6569=ORIENTED_EDGE ( 'NONE', *, *, #12893, .F. ) ;
#6570=LINE ( 'NONE', #7868, #11032 ) ;
#6572=ORIENTED_EDGE ( 'NONE', *, *, #14931, .T. ) ;
#6575=DIRECTION ( 'NONE',  ( -8.018662683283438208E-16, 5.975035461963189015E-16, 1.000000000000000000 ) ) ;
#6584=VERTEX_POINT ( 'NONE', #6116 ) ;
#6587=ORIENTED_EDGE ( 'NONE', *, *, #4770, .T. ) ;
#6589=DIRECTION ( 'NONE',  ( 0.2872152572324145892, 0.9578660637129379207, -3.420201433256678811E-16 ) ) ;
#6590=VERTEX_POINT ( 'NONE', #3689 ) ;
#6591=LINE ( 'NONE', #13081, #3984 ) ;
#6592=EDGE_CURVE ( 'NONE', #10291, #12780, #7317, .T. ) ;
#6598=CARTESIAN_POINT ( 'NONE',  ( -15.14850084941412511, -4.438867027711355107, 56.85231026484398598 ) ) ;
#6599=CARTESIAN_POINT ( 'NONE',  ( -15.53979317422733786, -13.47750381512840967, 56.85231026484398598 ) ) ;
#6601=ADVANCED_BREP_SHAPE_REPRESENTATION ( '', ( #7285, #6789 ), #8995 ) ;
#6602=ORIENTED_EDGE ( 'NONE', *, *, #9017, .T. ) ;
#6604=DIRECTION ( 'NONE',  ( 0.6334982226805353500, -0.7737441449604661736, 9.702957262759961121E-16 ) ) ;
#6605=VERTEX_POINT ( 'NONE', #12959 ) ;
#6606=DIRECTION ( 'NONE',  ( -0.6519834208811540188, -0.7582332219680881780, -6.975647374412566582E-17 ) ) ;
#6608=PLANE ( 'NONE',  #13742 ) ;
#6611=ORIENTED_EDGE ( 'NONE', *, *, #6967, .F. ) ;
#6613=EDGE_CURVE ( 'NONE', #12009, #6962, #9573, .T. ) ;
#6614=AXIS2_PLACEMENT_3D ( 'NONE', #826, #14896, #5482 ) ;
#6616=ADVANCED_FACE ( 'NONE', ( #14250 ), #7111, .T. ) ;
#6620=CARTESIAN_POINT ( 'NONE',  ( -5.628190034013323739, -14.94052892857136428, 54.00231026484399166 ) ) ;
#6621=VECTOR ( 'NONE', #7201, 1000.000000000000114 ) ;
#6622=ORIENTED_EDGE ( 'NONE', *, *, #3624, .F. ) ;
#6625=AXIS2_PLACEMENT_3D ( 'NONE', #11858, #13023, #8178 ) ;
#6626=EDGE_CURVE ( 'NONE', #6250, #560, #9225, .T. ) ;
#6627=EDGE_CURVE ( 'NONE', #12770, #11960, #2542, .T. ) ;
#6628=VERTEX_POINT ( 'NONE', #2394 ) ;
#6630=ORIENTED_EDGE ( 'NONE', *, *, #8604, .F. ) ;
#6635=DIRECTION ( 'NONE',  ( 8.018662683283438208E-16, -5.975035461963189015E-16, -1.000000000000000000 ) ) ;
#6638=CIRCLE ( 'NONE', #9583, 9.974999999999999645 ) ;
#6639=VECTOR ( 'NONE', #2911, 1000.000000000000000 ) ;
#6640=CARTESIAN_POINT ( 'NONE',  ( -23.45327702811275827, -7.487309620431347845, 54.00231026484397745 ) ) ;
#6645=CYLINDRICAL_SURFACE ( 'NONE', #13972, 0.2500000000000007216 ) ;
#6652=CONICAL_SURFACE ( 'NONE', #7133, 5.000000000000000000, 0.7853981633974476129 ) ;
#6653=LINE ( 'NONE', #11336, #7007 ) ;
#6658=EDGE_CURVE ( 'NONE', #11757, #9677, #1390, .T. ) ;
#6659=EDGE_CURVE ( 'NONE', #3870, #6300, #11194, .T. ) ;
#6661=AXIS2_PLACEMENT_3D ( 'NONE', #6599, #8758, #2109 ) ;
#6662=LINE ( 'NONE', #715, #2235 ) ;
#6668=EDGE_LOOP ( 'NONE', ( #555, #8336, #6260, #12263 ) ) ;
#6669=VERTEX_POINT ( 'NONE', #1544 ) ;
#6671=ORIENTED_EDGE ( 'NONE', *, *, #9548, .F. ) ;
#6674=DIRECTION ( 'NONE',  ( 0.8018662683283437342, -0.5975035461963188466, 9.999999999999996833E-16 ) ) ;
#6677=AXIS2_PLACEMENT_3D ( 'NONE', #10646, #4765, #14019 ) ;
#6682=CARTESIAN_POINT ( 'NONE',  ( -11.67714598312096008, -19.46131314156662384, 56.85231026484400019 ) ) ;
#6687=LINE ( 'NONE', #15111, #7856 ) ;
#6689=LINE ( 'NONE', #5401, #14034 ) ;
#6692=FACE_OUTER_BOUND ( 'NONE', #9846, .T. ) ;
#6694=DIRECTION ( 'NONE',  ( 0.8018662683283437342, -0.5975035461963188466, 9.999999999999996833E-16 ) ) ;
#6697=LINE ( 'NONE', #11377, #11640 ) ;
#6698=DIRECTION ( 'NONE',  ( 0.2536112499260065323, 0.9673062255102924389, -3.746065934159220994E-16 ) ) ;
#6699=LINE ( 'NONE', #10000, #1087 ) ;
#6704=VERTEX_POINT ( 'NONE', #12324 ) ;
#6706=ORIENTED_EDGE ( 'NONE', *, *, #1617, .T. ) ;
#6707=VERTEX_POINT ( 'NONE', #2767 ) ;
#6708=PLANE ( 'NONE',  #7376 ) ;
#6710=FACE_OUTER_BOUND ( 'NONE', #12204, .T. ) ;
#6711=EDGE_CURVE ( 'NONE', #8638, #9434, #3988, .T. ) ;
#6712=DIRECTION ( 'NONE',  ( -0.9040177279761056894, -0.4274949678123940444, -4.694715627858810513E-16 ) ) ;
#6713=ADVANCED_FACE ( 'NONE', ( #11097 ), #14397, .F. ) ;
#6715=PLANE ( 'NONE',  #692 ) ;
#6716=CARTESIAN_POINT ( 'NONE',  ( -7.517426579539127296, -14.72759957212633530, 56.85231026484400019 ) ) ;
#6719=ORIENTED_EDGE ( 'NONE', *, *, #14864, .F. ) ;
#6723=ORIENTED_EDGE ( 'NONE', *, *, #10794, .T. ) ;
#6724=DIRECTION ( 'NONE',  ( 0.5975035461963189576, 0.8018662683283437342, 0.000000000000000000 ) ) ;
#6727=CARTESIAN_POINT ( 'NONE',  ( -10.11292913755864475, -19.52351987967748315, 56.85231026484400019 ) ) ;
#6732=VERTEX_POINT ( 'NONE', #2837 ) ;
#6738=DIRECTION ( 'NONE',  ( 0.5691548339926102429, 0.8222303661035903488, -3.489949670250048422E-17 ) ) ;
#6743=DIRECTION ( 'NONE',  ( -0.9578660637129379207, 0.2872152572324145892, -9.396926207859088029E-16 ) ) ;
#6746=FACE_OUTER_BOUND ( 'NONE', #7182, .T. ) ;
#6747=DIRECTION ( 'NONE',  ( -8.018662683283438208E-16, 5.975035461963189015E-16, 1.000000000000000000 ) ) ;
#6748=CIRCLE ( 'NONE', #185, 9.974999999999999645 ) ;
#6749=AXIS2_PLACEMENT_3D ( 'NONE', #7228, #12139, #14366 ) ;
#6755=AXIS2_PLACEMENT_3D ( 'NONE', #9690, #4957, #9615 ) ;
#6759=DIRECTION ( 'NONE',  ( -0.8885476655824650072, -0.4587843131450243805, -4.383711467890778149E-16 ) ) ;
#6762=VERTEX_POINT ( 'NONE', #13476 ) ;
#6765=ADVANCED_FACE ( 'NONE', ( #7496 ), #4062, .F. ) ;
#6770=EDGE_CURVE ( 'NONE', #6628, #12018, #6417, .T. ) ;
#6771=LINE ( 'NONE', #14055, #12116 ) ;
#6772=CARTESIAN_POINT ( 'NONE',  ( -25.26605094763165127, -15.53691377877616731, 54.00231026484397745 ) ) ;
#6773=ORIENTED_EDGE ( 'NONE', *, *, #12625, .F. ) ;
#6775=LINE ( 'NONE', #8236, #3125 ) ;
#6776=CARTESIAN_POINT ( 'NONE',  ( -20.94048570341206883, -6.243833066724571168, 57.00231026484397745 ) ) ;
#6777=DIRECTION ( 'NONE',  ( -8.018662683283439195E-16, 5.975035461963190001E-16, 1.000000000000000000 ) ) ;
#6779=VECTOR ( 'NONE', #8091, 999.9999999999998863 ) ;
#6781=ORIENTED_EDGE ( 'NONE', *, *, #14691, .F. ) ;
#6782=EDGE_CURVE ( 'NONE', #5603, #10638, #4137, .T. ) ;
#6783=VECTOR ( 'NONE', #7937, 1000.000000000000000 ) ;
#6786=ADVANCED_FACE ( 'NONE', ( #5282 ), #5068, .F. ) ;
#6787=FACE_BOUND ( 'NONE', #5881, .T. ) ;
#6788=CARTESIAN_POINT ( 'NONE',  ( -7.691420491076302213, -11.44776172600821340, 56.85231026484400019 ) ) ;
#6789=AXIS2_PLACEMENT_3D ( 'NONE', #4381, #12419, #6809 ) ;
#6791=DIRECTION ( 'NONE',  ( -0.6780482080269577549, -0.7350174335289139105, -1.045284632676540317E-16 ) ) ;
#6793=DIRECTION ( 'NONE',  ( 8.018662683283438208E-16, -5.975035461963189015E-16, -1.000000000000000000 ) ) ;
#6796=AXIS2_PLACEMENT_3D ( 'NONE', #4146, #8877, #13483 ) ;
#6798=CARTESIAN_POINT ( 'NONE',  ( -5.859109405273535742, -10.94619944609606677, 54.00231026484399166 ) ) ;
#6800=ORIENTED_EDGE ( 'NONE', *, *, #11375, .F. ) ;
#6805=ORIENTED_EDGE ( 'NONE', *, *, #6154, .T. ) ;
#6807=ADVANCED_FACE ( 'NONE', ( #6242 ), #14298, .T. ) ;
#6808=DIRECTION ( 'NONE',  ( -8.018662683283438208E-16, 5.975035461963189015E-16, 1.000000000000000000 ) ) ;
#6809=DIRECTION ( 'NONE',  ( 1.000000000000000000, 0.000000000000000000, 0.000000000000000000 ) ) ;
#6812=AXIS2_PLACEMENT_3D ( 'NONE', #8825, #5388, #2870 ) ;
#6817=VERTEX_POINT ( 'NONE', #1287 ) ;
#6819=FACE_OUTER_BOUND ( 'NONE', #10189, .T. ) ;
#6820=ORIENTED_EDGE ( 'NONE', *, *, #1882, .T. ) ;
#6821=VERTEX_POINT ( 'NONE', #8474 ) ;
#6824=EDGE_CURVE ( 'NONE', #10152, #11272, #13234, .T. ) ;
#6830=DIRECTION ( 'NONE',  ( 8.018662683283438208E-16, -5.975035461963189015E-16, -1.000000000000000000 ) ) ;
#6832=CARTESIAN_POINT ( 'NONE',  ( -13.02562488396841900, -21.19439421350821817, 57.00231026484399166 ) ) ;
#6833=CARTESIAN_POINT ( 'NONE',  ( -10.08476707729037258, -21.88467736064467672, 54.00231026484400587 ) ) ;
#6835=VERTEX_POINT ( 'NONE', #7165 ) ;
#6836=CARTESIAN_POINT ( 'NONE',  ( -15.45378054160984682, -13.48759475315262613, 56.85231026484398598 ) ) ;
#6837=ORIENTED_EDGE ( 'NONE', *, *, #9266, .T. ) ;
#6840=CARTESIAN_POINT ( 'NONE',  ( -15.49969986081092088, -13.50737899243822504, 57.00231026484397745 ) ) ;
#6841=PLANE ( 'NONE',  #9130 ) ;
#6843=DIRECTION ( 'NONE',  ( -0.9645173894937556502, -0.2640193276336997297, -6.156614753256502225E-16 ) ) ;
#6844=EDGE_CURVE ( 'NONE', #13647, #4255, #7083, .T. ) ;
#6846=CARTESIAN_POINT ( 'NONE',  ( -6.488891646287396675, -12.42729319905174634, 56.85231026484400019 ) ) ;
#6848=EDGE_CURVE ( 'NONE', #2925, #8256, #2741, .T. ) ;
#6849=DIRECTION ( 'NONE',  ( -0.5975035461963188466, -0.8018662683283437342, 0.000000000000000000 ) ) ;
#6850=LINE ( 'NONE', #3498, #8901 ) ;
#6851=ORIENTED_EDGE ( 'NONE', *, *, #2242, .F. ) ;
#6855=ORIENTED_EDGE ( 'NONE', *, *, #13693, .T. ) ;
#6858=AXIS2_PLACEMENT_3D ( 'NONE', #5086, #12050, #1563 ) ;
#6859=CARTESIAN_POINT ( 'NONE',  ( -7.517426579539127296, -14.72759957212633530, 57.00231026484399166 ) ) ;
#6860=CARTESIAN_POINT ( 'NONE',  ( -18.93133274217424855, -21.90887563098697655, 56.85231026484400019 ) ) ;
#6861=LINE ( 'NONE', #1216, #309 ) ;
#6866=CARTESIAN_POINT ( 'NONE',  ( -8.858895634567669930, -20.95051974273373929, 57.00231026484399166 ) ) ;
#6867=DIRECTION ( 'NONE',  ( -8.018662683283438208E-16, 5.975035461963189015E-16, 1.000000000000000000 ) ) ;
#6869=ORIENTED_EDGE ( 'NONE', *, *, #11984, .T. ) ;
#6871=ORIENTED_EDGE ( 'NONE', *, *, #12653, .F. ) ;
#6872=CARTESIAN_POINT ( 'NONE',  ( -15.49969986081086226, -13.50737899243826767, -13.99768973515600301 ) ) ;
#6873=VERTEX_POINT ( 'NONE', #7237 ) ;
#6875=AXIS2_PLACEMENT_3D ( 'NONE', #9886, #13416, #13269 ) ;
#6876=PLANE ( 'NONE',  #11178 ) ;
#6877=VERTEX_POINT ( 'NONE', #12003 ) ;
#6881=AXIS2_PLACEMENT_3D ( 'NONE', #616, #13399, #6635 ) ;
#6882=CARTESIAN_POINT ( 'NONE',  ( -7.223083447440863836, -17.23012942000294245, 56.85231026484400019 ) ) ;
#6883=ADVANCED_FACE ( 'NONE', ( #1519 ), #6174, .F. ) ;
#6889=CARTESIAN_POINT ( 'NONE',  ( -10.11292913755864475, -19.52351987967748315, 56.85231026484400019 ) ) ;
#6890=VERTEX_POINT ( 'NONE', #5443 ) ;
#6892=VERTEX_POINT ( 'NONE', #2234 ) ;
#6893=ORIENTED_EDGE ( 'NONE', *, *, #12945, .T. ) ;
#6894=LINE ( 'NONE', #5682, #2734 ) ;
#6898=VECTOR ( 'NONE', #3376, 1000.000000000000114 ) ;
#6901=EDGE_CURVE ( 'NONE', #9153, #7447, #5520, .T. ) ;
#6904=CARTESIAN_POINT ( 'NONE',  ( -9.959408463899002584, -21.80230492564002276, 56.85231026484400019 ) ) ;
#6906=ORIENTED_EDGE ( 'NONE', *, *, #4003, .T. ) ;
#6907=LINE ( 'NONE', #3261, #11192 ) ;
#6908=DIRECTION ( 'NONE',  ( 0.5975035461963188466, 0.8018662683283437342, 0.000000000000000000 ) ) ;
#6910=ORIENTED_EDGE ( 'NONE', *, *, #8399, .F. ) ;
#6915=ORIENTED_EDGE ( 'NONE', *, *, #3938, .F. ) ;
#6916=CARTESIAN_POINT ( 'NONE',  ( -7.264457220180047692, -15.89840986842768977, 57.00231026484399166 ) ) ;
#6917=CARTESIAN_POINT ( 'NONE',  ( -20.06719866676104402, -21.34952185377683165, 57.00231026484397745 ) ) ;
#6921=EDGE_CURVE ( 'NONE', #1753, #3679, #9496, .T. ) ;
#6923=DIRECTION ( 'NONE',  ( 0.3204693369899919708, 0.9472588896649083434, -3.090169943749469383E-16 ) ) ;
#6924=EDGE_LOOP ( 'NONE', ( #11999, #4965, #3301, #11440 ) ) ;
#6926=VECTOR ( 'NONE', #5358, 999.9999999999998863 ) ;
#6927=LINE ( 'NONE', #3201, #7172 ) ;
#6928=DIRECTION ( 'NONE',  ( -8.018662683283438208E-16, 5.975035461963189015E-16, 1.000000000000000000 ) ) ;
#6929=ORIENTED_EDGE ( 'NONE', *, *, #8116, .T. ) ;
#6931=EDGE_LOOP ( 'NONE', ( #9546, #2308 ) ) ;
#6933=DIRECTION ( 'NONE',  ( -8.018662683283438208E-16, 5.975035461963189015E-16, 1.000000000000000000 ) ) ;
#6935=ADVANCED_FACE ( 'NONE', ( #173 ), #10494, .T. ) ;
#6936=DIRECTION ( 'NONE',  ( -8.018662683283439195E-16, 5.975035461963190001E-16, 1.000000000000000000 ) ) ;
#6940=CARTESIAN_POINT ( 'NONE',  ( -8.600581100527527667, -9.311215824554304632, 57.00231026484399166 ) ) ;
#6943=DIRECTION ( 'NONE',  ( 0.9578660637129379207, -0.2872152572324145892, 9.396926207859088029E-16 ) ) ;
#6946=VERTEX_POINT ( 'NONE', #1086 ) ;
#6947=ORIENTED_EDGE ( 'NONE', *, *, #9826, .F. ) ;
#6948=CARTESIAN_POINT ( 'NONE',  ( -24.55043086433169819, -12.83990741858047357, 56.85231026484398598 ) ) ;
#6949=ORIENTED_EDGE ( 'NONE', *, *, #13922, .T. ) ;
#6950=LINE ( 'NONE', #5817, #13184 ) ;
#6952=LINE ( 'NONE', #3454, #13332 ) ;
#6953=DIRECTION ( 'NONE',  ( 0.9957106782009863544, 0.09252159378508258147, 7.431448254773871651E-16 ) ) ;
#6956=ORIENTED_EDGE ( 'NONE', *, *, #7802, .F. ) ;
#6959=AXIS2_PLACEMENT_3D ( 'NONE', #11378, #6698, #14598 ) ;
#6962=VERTEX_POINT ( 'NONE', #14014 ) ;
#6964=ORIENTED_EDGE ( 'NONE', *, *, #2961, .F. ) ;
#6965=LINE ( 'NONE', #7281, #12532 ) ;
#6966=EDGE_CURVE ( 'NONE', #3490, #505, #6952, .T. ) ;
#6967=EDGE_CURVE ( 'NONE', #12833, #7723, #12804, .T. ) ;
#6972=DIRECTION ( 'NONE',  ( 0.5975035461963189576, 0.8018662683283437342, 0.000000000000000000 ) ) ;
#6973=DIRECTION ( 'NONE',  ( -8.018662683283438208E-16, 5.975035461963189015E-16, 1.000000000000000000 ) ) ;
#6975=DIRECTION ( 'NONE',  ( 0.9183863840214728791, 0.3956847857120156520, 4.999999999999998416E-16 ) ) ;
#6977=EDGE_LOOP ( 'NONE', ( #8744, #6518, #8710, #12368 ) ) ;
#6980=DIRECTION ( 'NONE',  ( -0.9999272109403024578, 0.01206535623791937274, -8.090169943749475688E-16 ) ) ;
#6984=ORIENTED_EDGE ( 'NONE', *, *, #10180, .T. ) ;
#6985=EDGE_CURVE ( 'NONE', #13132, #10963, #2391, .T. ) ;
#6990=CARTESIAN_POINT ( 'NONE',  ( -18.10194853779420399, -23.13696500758646835, 57.00231026484399166 ) ) ;
#6994=ORIENTED_EDGE ( 'NONE', *, *, #4157, .F. ) ;
#6995=DIRECTION ( 'NONE',  ( -0.6780482080269607525, -0.7350174335289111349, -1.045284632676580746E-16 ) ) ;
#6998=VECTOR ( 'NONE', #8942, 1000.000000000000000 ) ;
#6999=DIRECTION ( 'NONE',  ( -8.018662683283438208E-16, 5.975035461963189015E-16, 1.000000000000000000 ) ) ;
#7001=CARTESIAN_POINT ( 'NONE',  ( -12.95836108888110516, -12.41244868326982953, 51.00231026484399166 ) ) ;
#7002=ORIENTED_EDGE ( 'NONE', *, *, #11138, .F. ) ;
#7003=PLANE ( 'NONE',  #552 ) ;
#7005=ADVANCED_FACE ( 'NONE', ( #13033 ), #13940, .F. ) ;
#7007=VECTOR ( 'NONE', #2461, 1000.000000000000000 ) ;
#7011=DIRECTION ( 'NONE',  ( -0.9225966037272086417, 0.3857661296576204712, -9.702957262759976898E-16 ) ) ;
#7014=CIRCLE ( 'NONE', #452, 9.974999999999999645 ) ;
#7017=EDGE_CURVE ( 'NONE', #12259, #11477, #8264, .T. ) ;
#7018=CARTESIAN_POINT ( 'NONE',  ( -24.33650094517379614, -11.44044972528773130, 57.00231026484397745 ) ) ;
#7020=EDGE_LOOP ( 'NONE', ( #4291, #13042, #13719, #14334 ) ) ;
#7023=DIRECTION ( 'NONE',  ( 0.4800904676395372217, 0.8772189822852960450, -1.391731009600650064E-16 ) ) ;
#7024=VERTEX_POINT ( 'NONE', #14246 ) ;
#7025=ORIENTED_EDGE ( 'NONE', *, *, #11311, .T. ) ;
#7026=CARTESIAN_POINT ( 'NONE',  ( -7.424382730750141768, -13.52981220323889566, 57.00231026484399166 ) ) ;
#7027=ORIENTED_EDGE ( 'NONE', *, *, #503, .T. ) ;
#7036=VECTOR ( 'NONE', #8207, 1000.000000000000114 ) ;
#7037=EDGE_CURVE ( 'NONE', #10921, #33, #7107, .T. ) ;
#7038=PLANE ( 'NONE',  #10821 ) ;
#7045=ORIENTED_EDGE ( 'NONE', *, *, #788, .T. ) ;
#7046=DIRECTION ( 'NONE',  ( 8.018662683283438208E-16, -5.975035461963189015E-16, -1.000000000000000000 ) ) ;
#7047=ORIENTED_EDGE ( 'NONE', *, *, #743, .T. ) ;
#7048=DIRECTION ( 'NONE',  ( 0.9931883319083343320, -0.1165201156931293391, 8.660254037844387408E-16 ) ) ;
#7049=CIRCLE ( 'NONE', #7537, 9.974999999999999645 ) ;
#7061=VECTOR ( 'NONE', #12528, 1000.000000000000114 ) ;
#7064=ORIENTED_EDGE ( 'NONE', *, *, #12664, .T. ) ;
#7067=LINE ( 'NONE', #13902, #9475 ) ;
#7068=DIRECTION ( 'NONE',  ( 8.018662683283438208E-16, -5.975035461963189015E-16, -1.000000000000000000 ) ) ;
#7069=EDGE_CURVE ( 'NONE', #15017, #9709, #1316, .T. ) ;
#7070=DIRECTION ( 'NONE',  ( -0.1165201156931293391, -0.9931883319083343320, 4.999999999999998416E-16 ) ) ;
#7071=VECTOR ( 'NONE', #2236, 1000.000000000000000 ) ;
#7072=ORIENTED_EDGE ( 'NONE', *, *, #10463, .T. ) ;
#7073=CARTESIAN_POINT ( 'NONE',  ( -15.49969986081092088, -13.50737899243822504, 56.85231026484398598 ) ) ;
#7076=EDGE_CURVE ( 'NONE', #11595, #9643, #9873, .T. ) ;
#7080=ORIENTED_EDGE ( 'NONE', *, *, #5740, .F. ) ;
#7081=CARTESIAN_POINT ( 'NONE',  ( -15.49969986081091200, -13.50737899243823215, 48.00231026484398456 ) ) ;
#7082=CARTESIAN_POINT ( 'NONE',  ( -19.05456510292772521, -4.187316862259579331, 54.00231026484397745 ) ) ;
#7083=LINE ( 'NONE', #8395, #137 ) ;
#7084=ADVANCED_FACE ( 'NONE', ( #7341 ), #6113, .F. ) ;
#7085=CARTESIAN_POINT ( 'NONE',  ( -23.08034316846174150, -10.72437754756471762, 56.85231026484398598 ) ) ;
#7089=LINE ( 'NONE', #5652, #10412 ) ;
#7091=ORIENTED_EDGE ( 'NONE', *, *, #9245, .F. ) ;
#7093=EDGE_CURVE ( 'NONE', #7312, #4342, #3308, .T. ) ;
#7094=FACE_OUTER_BOUND ( 'NONE', #7798, .T. ) ;
#7095=VECTOR ( 'NONE', #5449, 1000.000000000000000 ) ;
#7096=CARTESIAN_POINT ( 'NONE',  ( -20.45368390747784204, -7.130130991507916072, 57.00231026484397745 ) ) ;
#7097=ORIENTED_EDGE ( 'NONE', *, *, #7069, .F. ) ;
#7100=ORIENTED_EDGE ( 'NONE', *, *, #10931, .F. ) ;
#7101=DIRECTION ( 'NONE',  ( 0.8719950447285833572, 0.4895147004624025300, 4.067366430758019417E-16 ) ) ;
#7105=ORIENTED_EDGE ( 'NONE', *, *, #10701, .T. ) ;
#7107=LINE ( 'NONE', #7188, #12100 ) ;
#7108=VECTOR ( 'NONE', #9880, 1000.000000000000227 ) ;
#7109=CARTESIAN_POINT ( 'NONE',  ( -10.22560374232860347, -19.62253721876480483, 56.85231026484400019 ) ) ;
#7111=PLANE ( 'NONE',  #6044 ) ;
#7112=LINE ( 'NONE', #5893, #13791 ) ;
#7113=EDGE_CURVE ( 'NONE', #2114, #9929, #14318, .T. ) ;
#7114=DIRECTION ( 'NONE',  ( 0.2975196656470014966, -0.9547156899063178326, 8.090169943749475688E-16 ) ) ;
#7115=AXIS2_PLACEMENT_3D ( 'NONE', #14031, #3547, #11804 ) ;
#7120=ORIENTED_EDGE ( 'NONE', *, *, #10381, .F. ) ;
#7123=PLANE ( 'NONE',  #7115 ) ;
#7124=VERTEX_POINT ( 'NONE', #1541 ) ;
#7126=EDGE_CURVE ( 'NONE', #8808, #9099, #6265, .T. ) ;
#7127=DIRECTION ( 'NONE',  ( -8.018662683283438208E-16, 5.975035461963189015E-16, 1.000000000000000000 ) ) ;
#7130=AXIS2_PLACEMENT_3D ( 'NONE', #4280, #8861, #14762 ) ;
#7133=AXIS2_PLACEMENT_3D ( 'NONE', #7266, #336, #14325 ) ;
#7135=FACE_OUTER_BOUND ( 'NONE', #14625, .T. ) ;
#7137=ORIENTED_EDGE ( 'NONE', *, *, #11650, .T. ) ;
#7139=CARTESIAN_POINT ( 'NONE',  ( -14.99866629829804765, -4.445910272123860807, 57.00231026484397745 ) ) ;
#7140=ORIENTED_EDGE ( 'NONE', *, *, #8228, .F. ) ;
#7143=ORIENTED_EDGE ( 'NONE', *, *, #3539, .T. ) ;
#7145=CIRCLE ( 'NONE', #7623, 4.500000000000000000 ) ;
#7149=AXIS2_PLACEMENT_3D ( 'NONE', #9899, #3011, #14792 ) ;
#7150=AXIS2_PLACEMENT_3D ( 'NONE', #2601, #2677, #10632 ) ;
#7151=CARTESIAN_POINT ( 'NONE',  ( -15.49969986081092088, -13.50737899243822504, 56.85231026484398598 ) ) ;
#7153=ORIENTED_EDGE ( 'NONE', *, *, #10510, .T. ) ;
#7155=LINE ( 'NONE', #4886, #13382 ) ;
#7157=DIRECTION ( 'NONE',  ( 0.5975035461963188466, 0.8018662683283437342, 0.000000000000000000 ) ) ;
#7158=ORIENTED_EDGE ( 'NONE', *, *, #9159, .T. ) ;
#7159=DIRECTION ( 'NONE',  ( 0.5975035461963189576, 0.8018662683283437342, 0.000000000000000000 ) ) ;
#7160=VERTEX_POINT ( 'NONE', #11016 ) ;
#7161=CARTESIAN_POINT ( 'NONE',  ( -17.62015867087677634, -21.29935591968936137, 56.85231026484400019 ) ) ;
#7163=CARTESIAN_POINT ( 'NONE',  ( -7.707227416580196611, -8.855645637450560770, 56.85231026484400019 ) ) ;
#7165=CARTESIAN_POINT ( 'NONE',  ( -8.701256315749452241, -15.46758698257906950, 57.00231026484399166 ) ) ;
#7166=AXIS2_PLACEMENT_3D ( 'NONE', #13231, #5039, #2737 ) ;
#7171=CARTESIAN_POINT ( 'NONE',  ( -18.61476135779618346, -20.95734656753543845, 56.85231026484398598 ) ) ;
#7172=VECTOR ( 'NONE', #12692, 1000.000000000000227 ) ;
#7177=PLANE ( 'NONE',  #12800 ) ;
#7179=DIRECTION ( 'NONE',  ( 8.018662683283438208E-16, -5.975035461963189015E-16, -1.000000000000000000 ) ) ;
#7182=EDGE_LOOP ( 'NONE', ( #430, #15076, #13786, #10578 ) ) ;
#7185=ORIENTED_EDGE ( 'NONE', *, *, #5208, .F. ) ;
#7186=EDGE_CURVE ( 'NONE', #6669, #13555, #617, .T. ) ;
#7187=EDGE_CURVE ( 'NONE', #4342, #1606, #4059, .T. ) ;
#7188=CARTESIAN_POINT ( 'NONE',  ( -16.17213342976032209, -5.460076146431361188, 56.85231026484398598 ) ) ;
#7191=CARTESIAN_POINT ( 'NONE',  ( -16.24681173062539230, -5.467015265965240012, 57.00231026484397745 ) ) ;
#7193=DIRECTION ( 'NONE',  ( -8.018662683283438208E-16, 5.975035461963189015E-16, 1.000000000000000000 ) ) ;
#7195=DIRECTION ( 'NONE',  ( 8.018662683283438208E-16, -5.975035461963189015E-16, -1.000000000000000000 ) ) ;
#7198=EDGE_LOOP ( 'NONE', ( #12562, #3697, #6187, #12752 ) ) ;
#7201=DIRECTION ( 'NONE',  ( -0.9966498018049937402, 0.08178736187251965661, -8.480480961564258050E-16 ) ) ;
#7203=PLANE ( 'NONE',  #3455 ) ;
#7204=FACE_OUTER_BOUND ( 'NONE', #2268, .T. ) ;
#7207=ADVANCED_FACE ( 'NONE', ( #3135 ), #6483, .T. ) ;
#7213=LINE ( 'NONE', #11893, #4098 ) ;
#7215=ORIENTED_EDGE ( 'NONE', *, *, #13526, .F. ) ;
#7216=ORIENTED_EDGE ( 'NONE', *, *, #6536, .F. ) ;
#7217=EDGE_CURVE ( 'NONE', #6762, #5844, #10087, .T. ) ;
#7220=CARTESIAN_POINT ( 'NONE',  ( -18.41596830400278506, -14.76384693893611910, 57.00231026484397745 ) ) ;
#7222=AXIS2_PLACEMENT_3D ( 'NONE', #903, #14526, #8701 ) ;
#7224=CARTESIAN_POINT ( 'NONE',  ( -7.016473591028805856, -8.259951331604915126, 54.00231026484399166 ) ) ;
#7226=DIRECTION ( 'NONE',  ( 8.018662683283438208E-16, -5.975035461963189015E-16, -1.000000000000000000 ) ) ;
#7228=CARTESIAN_POINT ( 'NONE',  ( -15.49969986081092088, -13.50737899243822504, 56.85231026484398598 ) ) ;
#7232=ORIENTED_EDGE ( 'NONE', *, *, #11063, .T. ) ;
#7233=DIRECTION ( 'NONE',  ( 8.018662683283438208E-16, -5.975035461963189015E-16, -1.000000000000000000 ) ) ;
#7234=ORIENTED_EDGE ( 'NONE', *, *, #7732, .F. ) ;
#7237=CARTESIAN_POINT ( 'NONE',  ( -17.05536012119625866, -6.605120582739408164, 56.85231026484398598 ) ) ;
#7240=DIRECTION ( 'NONE',  ( 0.3633925226508256667, -0.9316361277244830097, 8.480480961564259036E-16 ) ) ;
#7242=CARTESIAN_POINT ( 'NONE',  ( -7.506093261461533217, -14.65346081099997910, 57.00231026484399166 ) ) ;
#7246=DIRECTION ( 'NONE',  ( -0.9997391571607663341, -0.02283895005206026604, -7.880107536067206944E-16 ) ) ;
#7247=EDGE_CURVE ( 'NONE', #6704, #951, #13547, .T. ) ;
#7249=DIRECTION ( 'NONE',  ( 8.018662683283438208E-16, -5.975035461963189015E-16, -1.000000000000000000 ) ) ;
#7250=VERTEX_POINT ( 'NONE', #4365 ) ;
#7253=ORIENTED_EDGE ( 'NONE', *, *, #8116, .F. ) ;
#7254=VERTEX_POINT ( 'NONE', #6788 ) ;
#7255=EDGE_CURVE ( 'NONE', #11739, #5451, #12474, .T. ) ;
#7257=LINE ( 'NONE', #9934, #12521 ) ;
#7259=DIRECTION ( 'NONE',  ( -8.018662683283438208E-16, 5.975035461963189015E-16, 1.000000000000000000 ) ) ;
#7260=DIRECTION ( 'NONE',  ( 0.9826409426582659590, -0.1855175943453191700, 8.987940462991681405E-16 ) ) ;
#7261=DIRECTION ( 'NONE',  ( -8.018662683283438208E-16, 5.975035461963189015E-16, 1.000000000000000000 ) ) ;
#7263=CARTESIAN_POINT ( 'NONE',  ( -15.49969986081092088, -13.50737899243822504, 56.85231026484398598 ) ) ;
#7264=CIRCLE ( 'NONE', #3866, 9.974999999999999645 ) ;
#7265=VECTOR ( 'NONE', #3256, 1000.000000000000114 ) ;
#7266=CARTESIAN_POINT ( 'NONE',  ( -15.49969986081091022, -13.50737899243823215, 45.50231026484398456 ) ) ;
#7269=EDGE_CURVE ( 'NONE', #1866, #5883, #2069, .T. ) ;
#7271=DIRECTION ( 'NONE',  ( 0.9472588896649092316, -0.3204693369899889732, 9.510565162951523791E-16 ) ) ;
#7274=ORIENTED_EDGE ( 'NONE', *, *, #11266, .F. ) ;
#7279=VECTOR ( 'NONE', #1993, 1000.000000000000000 ) ;
#7280=LINE ( 'NONE', #6916, #5158 ) ;
#7281=CARTESIAN_POINT ( 'NONE',  ( -16.58746603607633929, -23.42289157363887142, 54.00231026484399166 ) ) ;
#7282=EDGE_CURVE ( 'NONE', #5816, #2807, #13009, .T. ) ;
#7283=CARTESIAN_POINT ( 'NONE',  ( -17.98267069058175593, -13.21607870320540457, 51.00231026484399166 ) ) ;
#7284=CARTESIAN_POINT ( 'NONE',  ( -9.376966593418606166, -18.77214511605354019, 56.85231026484400019 ) ) ;
#7285=MANIFOLD_SOLID_BREP ( 'Stock-MAS-672-1', #8277 ) ;
#7286=AXIS2_PLACEMENT_3D ( 'NONE', #10663, #8361, #9590 ) ;
#7290=EDGE_CURVE ( 'NONE', #4715, #10921, #12704, .T. ) ;
#7292=ORIENTED_EDGE ( 'NONE', *, *, #15055, .F. ) ;
#7293=DIRECTION ( 'NONE',  ( -8.018662683283438208E-16, 5.975035461963189015E-16, 1.000000000000000000 ) ) ;
#7296=EDGE_LOOP ( 'NONE', ( #13285, #8429, #9258, #7523 ) ) ;
#7302=CARTESIAN_POINT ( 'NONE',  ( -12.84086554789186607, -5.882298658668338120, 57.00231026484397745 ) ) ;
#7308=DIRECTION ( 'NONE',  ( 0.9918751611018171710, 0.1272150336605075427, 7.193398003386516820E-16 ) ) ;
#7309=ORIENTED_EDGE ( 'NONE', *, *, #2384, .F. ) ;
#7311=CARTESIAN_POINT ( 'NONE',  ( -11.55238169831532957, -21.67927775123549594, 56.85231026484400019 ) ) ;
#7312=VERTEX_POINT ( 'NONE', #3362 ) ;
#7313=ADVANCED_FACE ( 'NONE', ( #13921 ), #5727, .F. ) ;
#7315=CARTESIAN_POINT ( 'NONE',  ( -15.49969986081092088, -13.50737899243822504, 57.00231026484397745 ) ) ;
#7317=( BOUNDED_CURVE ( )  B_SPLINE_CURVE ( 3, ( #13183, #1320, #5975, #176 ),
 .UNSPECIFIED., .F., .F. ) 
 B_SPLINE_CURVE_WITH_KNOTS ( ( 4, 4 ),
 ( -8.881784197001252323E-16, 1.570796326794907216 ),
 .UNSPECIFIED. ) 
 CURVE ( )  GEOMETRIC_REPRESENTATION_ITEM ( )  RATIONAL_B_SPLINE_CURVE ( ( 1.000000000000000000, 0.8047378541243622729, 0.8047378541243622729, 1.000000000000000000 ) ) 
 REPRESENTATION_ITEM ( '' )  );
#7319=VERTEX_POINT ( 'NONE', #9551 ) ;
#7321=DIRECTION ( 'NONE',  ( -0.8018662683283436232, 0.5975035461963189576, -9.999999999999996833E-16 ) ) ;
#7330=PRODUCT ( 'Dial Adjustment Screw', 'Dial Adjustment Screw', '', ( #4347 ) ) ;
#7331=LINE ( 'NONE', #11936, #9108 ) ;
#7332=ORIENTED_EDGE ( 'NONE', *, *, #6320, .F. ) ;
#7334=ORIENTED_EDGE ( 'NONE', *, *, #8594, .T. ) ;
#7335=DIRECTION ( 'NONE',  ( -8.018662683283438208E-16, 5.975035461963189015E-16, 1.000000000000000000 ) ) ;
#7336=ORIENTED_EDGE ( 'NONE', *, *, #4675, .F. ) ;
#7337=ORIENTED_EDGE ( 'NONE', *, *, #3740, .F. ) ;
#7338=VECTOR ( 'NONE', #1088, 999.9999999999998863 ) ;
#7341=FACE_OUTER_BOUND ( 'NONE', #8224, .T. ) ;
#7345=DIRECTION ( 'NONE',  ( 8.018662683283438208E-16, -5.975035461963189015E-16, -1.000000000000000000 ) ) ;
#7346=LINE ( 'NONE', #4920, #13276 ) ;
#7347=DIRECTION ( 'NONE',  ( -0.1511109077013150781, -0.9885168150181790070, 4.694715627858902218E-16 ) ) ;
#7354=EDGE_LOOP ( 'NONE', ( #12001, #8657, #7412, #14515, #4271, #5177 ) ) ;
#7355=VERTEX_POINT ( 'NONE', #8169 ) ;
#7359=FACE_OUTER_BOUND ( 'NONE', #592, .T. ) ;
#7362=AXIS2_PLACEMENT_3D ( 'NONE', #12793, #13928, #1226 ) ;
#7364=PLANE ( 'NONE',  #9313 ) ;
#7365=FACE_OUTER_BOUND ( 'NONE', #14140, .T. ) ;
#7366=ORIENTED_EDGE ( 'NONE', *, *, #14320, .T. ) ;
#7368=ORIENTED_EDGE ( 'NONE', *, *, #2626, .T. ) ;
#7371=ORIENTED_EDGE ( 'NONE', *, *, #9357, .T. ) ;
#7375=VECTOR ( 'NONE', #10690, 1000.000000000000227 ) ;
#7376=AXIS2_PLACEMENT_3D ( 'NONE', #13763, #10010, #915 ) ;
#7377=VECTOR ( 'NONE', #7687, 1000.000000000000227 ) ;
#7378=VECTOR ( 'NONE', #4283, 1000.000000000000000 ) ;
#7382=CARTESIAN_POINT ( 'NONE',  ( -23.12048770254168062, -16.17743848078839619, 57.00231026484397745 ) ) ;
#7383=EDGE_CURVE ( 'NONE', #6584, #1349, #1805, .T. ) ;
#7388=AXIS2_PLACEMENT_3D ( 'NONE', #2177, #3322, #4547 ) ;
#7389=FACE_OUTER_BOUND ( 'NONE', #12425, .T. ) ;
#7391=AXIS2_PLACEMENT_3D ( 'NONE', #2150, #7945, #4597 ) ;
#7394=VERTEX_POINT ( 'NONE', #13584 ) ;
#7395=LINE ( 'NONE', #11073, #8144 ) ;
#7397=CARTESIAN_POINT ( 'NONE',  ( -22.56723502526082470, -13.84084068328822248, 56.85231026484398598 ) ) ;
#7400=CIRCLE ( 'NONE', #819, 4.500000000000000000 ) ;
#7405=LINE ( 'NONE', #105, #13060 ) ;
#7407=LINE ( 'NONE', #2449, #5781 ) ;
#7410=ORIENTED_EDGE ( 'NONE', *, *, #11266, .T. ) ;
#7412=ORIENTED_EDGE ( 'NONE', *, *, #11504, .T. ) ;
#7414=ADVANCED_FACE ( 'NONE', ( #14223 ), #10983, .F. ) ;
#7416=DIRECTION ( 'NONE',  ( 0.4274949678123838859, -0.9040177279761104634, 8.829475928589268008E-16 ) ) ;
#7417=DIRECTION ( 'NONE',  ( -0.4274949678123838859, 0.9040177279761104634, -8.829475928589268008E-16 ) ) ;
#7420=VECTOR ( 'NONE', #13809, 1000.000000000000000 ) ;
#7424=AXIS2_PLACEMENT_3D ( 'NONE', #896, #8920, #3337 ) ;
#7425=FACE_OUTER_BOUND ( 'NONE', #15124, .T. ) ;
#7426=DIRECTION ( 'NONE',  ( -8.018662683283438208E-16, 5.975035461963189015E-16, 1.000000000000000000 ) ) ;
#7427=VERTEX_POINT ( 'NONE', #14728 ) ;
#7428=DIRECTION ( 'NONE',  ( -8.018662683283438208E-16, 5.975035461963189015E-16, 1.000000000000000000 ) ) ;
#7429=VERTEX_POINT ( 'NONE', #8677 ) ;
#7430=ORIENTED_EDGE ( 'NONE', *, *, #4732, .T. ) ;
#7438=CARTESIAN_POINT ( 'NONE',  ( -9.959408463899002584, -21.80230492564002276, 57.00231026484399166 ) ) ;
#7439=FACE_OUTER_BOUND ( 'NONE', #13029, .T. ) ;
#7440=VECTOR ( 'NONE', #7260, 1000.000000000000114 ) ;
#7443=ORIENTED_EDGE ( 'NONE', *, *, #7753, .T. ) ;
#7444=LINE ( 'NONE', #1792, #10200 ) ;
#7447=VERTEX_POINT ( 'NONE', #1954 ) ;
#7448=ORIENTED_EDGE ( 'NONE', *, *, #10846, .T. ) ;
#7449=EDGE_CURVE ( 'NONE', #4500, #4715, #807, .T. ) ;
#7450=FACE_OUTER_BOUND ( 'NONE', #3580, .T. ) ;
#7454=DIRECTION ( 'NONE',  ( 0.8415927028326188886, -0.5401126942952620968, 9.975640502598240034E-16 ) ) ;
#7456=EDGE_CURVE ( 'NONE', #5960, #12040, #4093, .T. ) ;
#7458=CARTESIAN_POINT ( 'NONE',  ( -23.05384319539488658, -10.65421522557165623, 57.00231026484397745 ) ) ;
#7460=DIRECTION ( 'NONE',  ( -0.1165201156931293391, -0.9931883319083343320, 4.999999999999998416E-16 ) ) ;
#7462=DIRECTION ( 'NONE',  ( -8.018662683283439195E-16, 5.975035461963190001E-16, 1.000000000000000000 ) ) ;
#7463=EDGE_LOOP ( 'NONE', ( #7216, #13097, #13343, #13893 ) ) ;
#7466=ADVANCED_FACE ( 'NONE', ( #4322, #12504 ), #3323, .T. ) ;
#7467=EDGE_LOOP ( 'NONE', ( #9617, #14796, #14287, #2321 ) ) ;
#7469=FACE_OUTER_BOUND ( 'NONE', #3844, .T. ) ;
#7473=DIRECTION ( 'NONE',  ( -8.018662683283438208E-16, 5.975035461963189015E-16, 1.000000000000000000 ) ) ;
#7478=VERTEX_POINT ( 'NONE', #3254 ) ;
#7479=CARTESIAN_POINT ( 'NONE',  ( -18.48721759179245439, -17.51671033407998479, -13.99768973515600301 ) ) ;
#7486=ORIENTED_EDGE ( 'NONE', *, *, #4492, .T. ) ;
#7487=ORIENTED_EDGE ( 'NONE', *, *, #601, .T. ) ;
#7488=CARTESIAN_POINT ( 'NONE',  ( -24.01584079503567182, -10.37104457333969876, 56.85231026484398598 ) ) ;
#7491=AXIS2_PLACEMENT_3D ( 'NONE', #14026, #4392, #14870 ) ;
#7496=FACE_OUTER_BOUND ( 'NONE', #5490, .T. ) ;
#7497=ADVANCED_FACE ( 'NONE', ( #10203 ), #10280, .T. ) ;
#7502=ORIENTED_EDGE ( 'NONE', *, *, #7247, .F. ) ;
#7503=CARTESIAN_POINT ( 'NONE',  ( -19.19431052208641120, -4.241825740657187538, 54.00231026484397745 ) ) ;
#7506=VERTEX_POINT ( 'NONE', #13729 ) ;
#7509=LINE ( 'NONE', #11189, #9511 ) ;
#7510=AXIS2_PLACEMENT_3D ( 'NONE', #10785, #13320, #8558 ) ;
#7511=AXIS2_PLACEMENT_3D ( 'NONE', #8368, #6975, #9675 ) ;
#7512=FACE_OUTER_BOUND ( 'NONE', #9831, .T. ) ;
#7513=VECTOR ( 'NONE', #3527, 1000.000000000000000 ) ;
#7514=LINE ( 'NONE', #1859, #7528 ) ;
#7515=ADVANCED_FACE ( 'NONE', ( #7973 ), #2180, .F. ) ;
#7516=ADVANCED_FACE ( 'NONE', ( #6746 ), #9127, .F. ) ;
#7517=DIRECTION ( 'NONE',  ( 8.018662683283438208E-16, -5.975035461963189015E-16, -1.000000000000000000 ) ) ;
#7518=CARTESIAN_POINT ( 'NONE',  ( -9.539601987502638991, -5.508762965862997518, 57.00231026484397745 ) ) ;
#7519=ORIENTED_EDGE ( 'NONE', *, *, #3916, .T. ) ;
#7520=CARTESIAN_POINT ( 'NONE',  ( -15.49969986081092088, -13.50737899243822504, 57.00231026484397745 ) ) ;
#7521=LINE ( 'NONE', #5155, #14827 ) ;
#7522=ORIENTED_EDGE ( 'NONE', *, *, #6844, .T. ) ;
#7523=ORIENTED_EDGE ( 'NONE', *, *, #2517, .T. ) ;
#7525=CARTESIAN_POINT ( 'NONE',  ( -25.43486656742121355, -12.61682438329676081, 57.00231026484397745 ) ) ;
#7526=ORIENTED_EDGE ( 'NONE', *, *, #5026, .F. ) ;
#7527=DIRECTION ( 'NONE',  ( 0.4800904676395346127, 0.8772189822852974883, -1.391731009600680140E-16 ) ) ;
#7528=VECTOR ( 'NONE', #637, 1000.000000000000227 ) ;
#7534=DIRECTION ( 'NONE',  ( -0.5975035461963187355, -0.8018662683283439563, 0.000000000000000000 ) ) ;
#7535=ORIENTED_EDGE ( 'NONE', *, *, #8914, .F. ) ;
#7536=CARTESIAN_POINT ( 'NONE',  ( -18.06278547315525529, -11.75340479732393817, 57.00231026484397745 ) ) ;
#7537=AXIS2_PLACEMENT_3D ( 'NONE', #4681, #10565, #6111 ) ;
#7538=CARTESIAN_POINT ( 'NONE',  ( -15.12053853660593283, -5.441285657357897598, 56.85231026484398598 ) ) ;
#7539=ORIENTED_EDGE ( 'NONE', *, *, #4961, .F. ) ;
#7542=ORIENTED_EDGE ( 'NONE', *, *, #9704, .T. ) ;
#7543=CARTESIAN_POINT ( 'NONE',  ( -20.33437667196779586, -7.039214636791314206, 56.85231026484398598 ) ) ;
#7544=ORIENTED_EDGE ( 'NONE', *, *, #10660, .F. ) ;
#7545=CARTESIAN_POINT ( 'NONE',  ( -8.858895634567668154, -20.95051974273374285, 54.00231026484400587 ) ) ;
#7548=AXIS2_PLACEMENT_3D ( 'NONE', #12917, #8300, #3797 ) ;
#7549=EDGE_CURVE ( 'NONE', #5960, #2827, #13450, .T. ) ;
#7550=DIRECTION ( 'NONE',  ( -0.8222303661035904598, 0.5691548339926102429, -9.993908270190959005E-16 ) ) ;
#7551=DIRECTION ( 'NONE',  ( -0.7511640317997426708, -0.6601155939154560448, -2.079116908177589032E-16 ) ) ;
#7555=CARTESIAN_POINT ( 'NONE',  ( -14.11952815701477881, -21.46390939632912875, 57.00231026484399166 ) ) ;
#7556=LINE ( 'NONE', #236, #11924 ) ;
#7557=ORIENTED_EDGE ( 'NONE', *, *, #12500, .T. ) ;
#7558=VERTEX_POINT ( 'NONE', #2409 ) ;
#7559=FACE_OUTER_BOUND ( 'NONE', #4837, .T. ) ;
#7568=DIRECTION ( 'NONE',  ( 0.6061090314441981430, -0.7953815700667045130, 9.612616959383179548E-16 ) ) ;
#7576=ORIENTED_EDGE ( 'NONE', *, *, #13065, .T. ) ;
#7577=CARTESIAN_POINT ( 'NONE',  ( -15.49969986081092088, -13.50737899243822504, 56.85231026484398598 ) ) ;
#7578=CIRCLE ( 'NONE', #993, 9.974999999999999645 ) ;
#7581=LINE ( 'NONE', #11107, #6176 ) ;
#7582=EDGE_LOOP ( 'NONE', ( #5774, #14518, #11334, #1227 ) ) ;
#7584=CARTESIAN_POINT ( 'NONE',  ( -15.49969986081092088, -13.50737899243822504, 56.85231026484398598 ) ) ;
#7585=CARTESIAN_POINT ( 'NONE',  ( -22.13265177292497299, -18.11337496850924822, 56.85231026484398598 ) ) ;
#7587=ORIENTED_EDGE ( 'NONE', *, *, #7093, .F. ) ;
#7590=CARTESIAN_POINT ( 'NONE',  ( -7.711221940648826489, -11.37542292179617753, 56.85231026484400019 ) ) ;
#7591=EDGE_CURVE ( 'NONE', #13132, #7744, #12894, .T. ) ;
#7593=CARTESIAN_POINT ( 'NONE',  ( -20.59651154950486784, -18.41489981358536809, 57.00231026484397745 ) ) ;
#7594=PLANE ( 'NONE',  #8402 ) ;
#7597=DIRECTION ( 'NONE',  ( -0.8772189822852959340, 0.4800904676395371662, -9.902680687415702019E-16 ) ) ;
#7598=ORIENTED_EDGE ( 'NONE', *, *, #14088, .F. ) ;
#7599=ORIENTED_EDGE ( 'NONE', *, *, #12253, .T. ) ;
#7600=FACE_OUTER_BOUND ( 'NONE', #383, .T. ) ;
#7601=AXIS2_PLACEMENT_3D ( 'NONE', #4745, #11418, #12576 ) ;
#7604=ADVANCED_FACE ( 'NONE', ( #5906 ), #6058, .T. ) ;
#7609=DIRECTION ( 'NONE',  ( 0.5975035461963189576, 0.8018662683283437342, 0.000000000000000000 ) ) ;
#7610=CARTESIAN_POINT ( 'NONE',  ( -7.731023390221355207, -11.30308411758414877, 56.85231026484400019 ) ) ;
#7612=DIRECTION ( 'NONE',  ( 8.018662683283438208E-16, -5.975035461963189015E-16, -1.000000000000000000 ) ) ;
#7616=CARTESIAN_POINT ( 'NONE',  ( -15.49969986081091378, -13.50737899243822859, 51.00231026484399166 ) ) ;
#7619=AXIS2_PLACEMENT_3D ( 'NONE', #11921, #1517, #4968 ) ;
#7623=AXIS2_PLACEMENT_3D ( 'NONE', #3538, #7195, #1240 ) ;
#7625=DIRECTION ( 'NONE',  ( -0.3633925226508256667, 0.9316361277244830097, -8.480480961564259036E-16 ) ) ;
#7631=ORIENTED_EDGE ( 'NONE', *, *, #14302, .T. ) ;
#7633=ADVANCED_FACE ( 'NONE', ( #191 ), #2631, .F. ) ;
#7637=EDGE_CURVE ( 'NONE', #964, #12427, #2460, .T. ) ;
#7638=CARTESIAN_POINT ( 'NONE',  ( -15.49969986081091200, -13.50737899243823037, 48.00231026484398456 ) ) ;
#7640=DIRECTION ( 'NONE',  ( -0.1960948578651675878, 0.9805849309054466278, -7.431448254773955467E-16 ) ) ;
#7643=AXIS2_PLACEMENT_3D ( 'NONE', #5257, #3887, #10851 ) ;
#7644=DIRECTION ( 'NONE',  ( -8.018662683283438208E-16, 5.975035461963189015E-16, 1.000000000000000000 ) ) ;
#7645=VERTEX_POINT ( 'NONE', #6290 ) ;
#7649=CARTESIAN_POINT ( 'NONE',  ( -6.368730986314236731, -9.491655842995191605, 54.00231026484399166 ) ) ;
#7650=DIRECTION ( 'NONE',  ( 0.5975035461963189576, 0.8018662683283437342, 0.000000000000000000 ) ) ;
#7651=VERTEX_POINT ( 'NONE', #13345 ) ;
#7655=EDGE_CURVE ( 'NONE', #6300, #2715, #11034, .T. ) ;
#7656=LINE ( 'NONE', #10832, #362 ) ;
#7657=VERTEX_POINT ( 'NONE', #13420 ) ;
#7661=LINE ( 'NONE', #8664, #14138 ) ;
#7663=VECTOR ( 'NONE', #7930, 1000.000000000000000 ) ;
#7664=DIRECTION ( 'NONE',  ( 0.1855175943453168941, 0.9826409426582662920, -4.383711467890769768E-16 ) ) ;
#7665=ORIENTED_EDGE ( 'NONE', *, *, #6524, .F. ) ;
#7666=DIRECTION ( 'NONE',  ( 8.018662683283438208E-16, -5.975035461963189015E-16, -1.000000000000000000 ) ) ;
#7671=VECTOR ( 'NONE', #14902, 1000.000000000000227 ) ;
#7672=CARTESIAN_POINT ( 'NONE',  ( -7.707227416580196611, -8.855645637450560770, 56.85231026484400019 ) ) ;
#7673=EDGE_CURVE ( 'NONE', #4906, #4831, #636, .T. ) ;
#7674=VERTEX_POINT ( 'NONE', #9890 ) ;
#7675=CARTESIAN_POINT ( 'NONE',  ( -25.44713467170207366, -12.76632185356751847, 54.00231026484397745 ) ) ;
#7676=EDGE_CURVE ( 'NONE', #3314, #10056, #3918, .T. ) ;
#7679=VECTOR ( 'NONE', #11849, 999.9999999999998863 ) ;
#7680=FACE_OUTER_BOUND ( 'NONE', #13501, .T. ) ;
#7684=VERTEX_POINT ( 'NONE', #2933 ) ;
#7685=DIRECTION ( 'NONE',  ( 0.5975035461963187355, 0.8018662683283439563, 0.000000000000000000 ) ) ;
#7687=DIRECTION ( 'NONE',  ( -0.9755678736739583634, 0.2196982563774038943, -9.135454576426008610E-16 ) ) ;
#7688=CARTESIAN_POINT ( 'NONE',  ( -23.14528701667493849, -16.10665716956490812, 56.85231026484398598 ) ) ;
#7690=ORIENTED_EDGE ( 'NONE', *, *, #3781, .T. ) ;
#7691=DIRECTION ( 'NONE',  ( -8.018662683283439195E-16, 5.975035461963190001E-16, 1.000000000000000000 ) ) ;
#7692=LINE ( 'NONE', #6467, #727 ) ;
#7695=ADVANCED_FACE ( 'NONE', ( #9744 ), #6436, .F. ) ;
#7696=CARTESIAN_POINT ( 'NONE',  ( -15.49969986081091022, -13.50737899243823215, 45.50231026484398456 ) ) ;
#7697=DIRECTION ( 'NONE',  ( -8.018662683283438208E-16, 5.975035461963189015E-16, 1.000000000000000000 ) ) ;
#7702=ORIENTED_EDGE ( 'NONE', *, *, #2573, .T. ) ;
#7704=ORIENTED_EDGE ( 'NONE', *, *, #10855, .T. ) ;
#7708=DIRECTION ( 'NONE',  ( -0.1960948578651647567, 0.9805849309054472940, -7.431448254773936732E-16 ) ) ;
#7713=CARTESIAN_POINT ( 'NONE',  ( -23.40321606353253614, -15.16438883951732741, 57.00231026484397745 ) ) ;
#7714=LINE ( 'NONE', #696, #6926 ) ;
#7717=ORIENTED_EDGE ( 'NONE', *, *, #7113, .F. ) ;
#7719=VECTOR ( 'NONE', #11767, 1000.000000000000000 ) ;
#7720=ORIENTED_EDGE ( 'NONE', *, *, #2990, .F. ) ;
#7721=LINE ( 'NONE', #8078, #14398 ) ;
#7722=CARTESIAN_POINT ( 'NONE',  ( -16.39856880423293006, -20.52544743201270450, 57.00231026484399166 ) ) ;
#7723=VERTEX_POINT ( 'NONE', #9958 ) ;
#7726=DIRECTION ( 'NONE',  ( -0.1855175943453168941, -0.9826409426582662920, 4.383711467890769768E-16 ) ) ;
#7727=ORIENTED_EDGE ( 'NONE', *, *, #5788, .F. ) ;
#7729=CARTESIAN_POINT ( 'NONE',  ( -15.49969986081092088, -13.50737899243822504, 56.85231026484398598 ) ) ;
#7731=ADVANCED_FACE ( 'NONE', ( #7512 ), #4155, .T. ) ;
#7732=EDGE_CURVE ( 'NONE', #6817, #5856, #13569, .T. ) ;
#7733=PLANE ( 'NONE',  #7601 ) ;
#7735=DIRECTION ( 'NONE',  ( -0.5975035461963189576, -0.8018662683283438453, 9.860761315262649757E-32 ) ) ;
#7738=DIRECTION ( 'NONE',  ( -0.3956847857120157075, 0.9183863840214729901, -8.660254037844388394E-16 ) ) ;
#7741=ORIENTED_EDGE ( 'NONE', *, *, #5599, .T. ) ;
#7742=ORIENTED_EDGE ( 'NONE', *, *, #7456, .F. ) ;
#7744=VERTEX_POINT ( 'NONE', #12267 ) ;
#7745=CIRCLE ( 'NONE', #12149, 9.974999999999999645 ) ;
#7752=DIRECTION ( 'NONE',  ( 0.5975035461963188466, 0.8018662683283437342, 0.000000000000000000 ) ) ;
#7753=EDGE_CURVE ( 'NONE', #12040, #2877, #7879, .T. ) ;
#7754=AXIS2_PLACEMENT_3D ( 'NONE', #4198, #12310, #4355 ) ;
#7755=VECTOR ( 'NONE', #11199, 1000.000000000000000 ) ;
#7756=DIRECTION ( 'NONE',  ( -8.018662683283438208E-16, 5.975035461963189015E-16, 1.000000000000000000 ) ) ;
#7759=VECTOR ( 'NONE', #4511, 1000.000000000000227 ) ;
#7771=CARTESIAN_POINT ( 'NONE',  ( -23.59767874945767119, -17.60420555931063902, 56.85231026484398598 ) ) ;
#7772=VECTOR ( 'NONE', #5988, 1000.000000000000114 ) ;
#7773=DIRECTION ( 'NONE',  ( -8.018662683283438208E-16, 5.975035461963189015E-16, 1.000000000000000000 ) ) ;
#7774=CARTESIAN_POINT ( 'NONE',  ( -22.56290636796585503, -13.91571566392944526, 56.85231026484398598 ) ) ;
#7775=ADVANCED_FACE ( 'NONE', ( #13713 ), #3233, .T. ) ;
#7776=ORIENTED_EDGE ( 'NONE', *, *, #11151, .T. ) ;
#7780=CARTESIAN_POINT ( 'NONE',  ( -20.54757852167729837, -19.81012014412530320, 56.85231026484398598 ) ) ;
#7781=ORIENTED_EDGE ( 'NONE', *, *, #117, .T. ) ;
#7783=CARTESIAN_POINT ( 'NONE',  ( -24.28571865450477318, -8.784403367172064492, 54.00231026484397745 ) ) ;
#7786=ADVANCED_FACE ( 'NONE', ( #8958 ), #15082, .F. ) ;
#7788=DIRECTION ( 'NONE',  ( -8.018662683283438208E-16, 5.975035461963189015E-16, 1.000000000000000000 ) ) ;
#7789=LINE ( 'NONE', #11395, #2851 ) ;
#7790=CARTESIAN_POINT ( 'NONE',  ( -15.80242800153736837, -16.08775797096295435, 51.00231026484399166 ) ) ;
#7793=LINE ( 'NONE', #1142, #1292 ) ;
#7798=EDGE_LOOP ( 'NONE', ( #10023, #8279, #13417, #8818 ) ) ;
#7799=CARTESIAN_POINT ( 'NONE',  ( -15.49969986081091733, -13.50737899243822682, 54.00231026484399166 ) ) ;
#7802=EDGE_CURVE ( 'NONE', #13942, #3312, #4380, .T. ) ;
#7803=DIRECTION ( 'NONE',  ( 8.018662683283438208E-16, -5.975035461963189015E-16, -1.000000000000000000 ) ) ;
#7807=ORIENTED_EDGE ( 'NONE', *, *, #1803, .F. ) ;
#7810=DIRECTION ( 'NONE',  ( 0.5975035461963189576, 0.8018662683283437342, 0.000000000000000000 ) ) ;
#7814=ORIENTED_EDGE ( 'NONE', *, *, #13728, .T. ) ;
#7816=EDGE_CURVE ( 'NONE', #8987, #6022, #864, .T. ) ;
#7819=CARTESIAN_POINT ( 'NONE',  ( -23.08034316846174150, -10.72437754756471762, 56.85231026484398598 ) ) ;
#7820=VECTOR ( 'NONE', #14000, 1000.000000000000114 ) ;
#7822=CARTESIAN_POINT ( 'NONE',  ( -12.73873237239188683, -12.31782212615591021, 57.00231026484397745 ) ) ;
#7825=CARTESIAN_POINT ( 'NONE',  ( -12.37415300023346454, -4.034703455804748984, 54.00231026484399166 ) ) ;
#7826=CYLINDRICAL_SURFACE ( 'NONE', #8265, 5.000000000000000000 ) ;
#7829=VERTEX_POINT ( 'NONE', #8036 ) ;
#7831=CARTESIAN_POINT ( 'NONE',  ( -15.49969986081092088, -13.50737899243822504, 56.85231026484398598 ) ) ;
#7833=DIRECTION ( 'NONE',  ( -0.4224988092984270360, -0.5670050759397227136, 0.7071067811865480168 ) ) ;
#7834=EDGE_CURVE ( 'NONE', #505, #7429, #10338, .T. ) ;
#7835=EDGE_CURVE ( 'NONE', #11757, #6457, #11489, .T. ) ;
#7840=LINE ( 'NONE', #2965, #14561 ) ;
#7841=CARTESIAN_POINT ( 'NONE',  ( -18.93133274217424855, -21.90887563098697655, 56.85231026484400019 ) ) ;
#7844=DIRECTION ( 'NONE',  ( -0.9918751611018171710, -0.1272150336605075427, -7.193398003386516820E-16 ) ) ;
#7846=CARTESIAN_POINT ( 'NONE',  ( -22.33089034576175180, -8.323646113680169378, 56.85231026484398598 ) ) ;
#7847=AXIS2_PLACEMENT_3D ( 'NONE', #255, #3616, #8350 ) ;
#7851=ORIENTED_EDGE ( 'NONE', *, *, #7835, .T. ) ;
#7855=EDGE_CURVE ( 'NONE', #8000, #4906, #4534, .T. ) ;
#7856=VECTOR ( 'NONE', #13966, 1000.000000000000114 ) ;
#7861=VECTOR ( 'NONE', #5115, 1000.000000000000000 ) ;
#7862=CARTESIAN_POINT ( 'NONE',  ( -24.80452494096261873, -9.912819877918101596, 56.85231026484398598 ) ) ;
#7863=CARTESIAN_POINT ( 'NONE',  ( -9.376966593418606166, -18.77214511605354019, 57.00231026484399166 ) ) ;
#7864=DIRECTION ( 'NONE',  ( -0.3306575217771128283, 0.9437508163134049610, -8.290375725550417844E-16 ) ) ;
#7865=EDGE_CURVE ( 'NONE', #11873, #12154, #5747, .T. ) ;
#7866=CARTESIAN_POINT ( 'NONE',  ( -16.48891182509095543, -11.21141303238454334, 51.25231026484399166 ) ) ;
#7868=CARTESIAN_POINT ( 'NONE',  ( -12.84086554789186607, -5.882298658668338120, 56.85231026484398598 ) ) ;
#7869=AXIS2_PLACEMENT_3D ( 'NONE', #7969, #12503, #3252 ) ;
#7874=EDGE_LOOP ( 'NONE', ( #87, #1110, #1331, #9796 ) ) ;
#7875=AXIS2_PLACEMENT_3D ( 'NONE', #3241, #869, #9350 ) ;
#7876=CARTESIAN_POINT ( 'NONE',  ( -17.87376992080280758, -22.26666214519964271, 57.00231026484399166 ) ) ;
#7879=LINE ( 'NONE', #4305, #7071 ) ;
#7880=AXIS2_PLACEMENT_3D ( 'NONE', #9676, #14116, #2642 ) ;
#7881=AXIS2_PLACEMENT_3D ( 'NONE', #6872, #5584, #4676 ) ;
#7882=AXIS2_PLACEMENT_3D ( 'NONE', #12993, #14285, #9911 ) ;
#7883=VECTOR ( 'NONE', #14888, 1000.000000000000114 ) ;
#7884=EDGE_LOOP ( 'NONE', ( #7368, #8784, #1639, #8333 ) ) ;
#7885=FACE_OUTER_BOUND ( 'NONE', #4680, .T. ) ;
#7888=ORIENTED_EDGE ( 'NONE', *, *, #3707, .F. ) ;
#7890=ORIENTED_EDGE ( 'NONE', *, *, #5408, .T. ) ;
#7892=VERTEX_POINT ( 'NONE', #8344 ) ;
#7893=ORIENTED_EDGE ( 'NONE', *, *, #669, .F. ) ;
#7895=ORIENTED_EDGE ( 'NONE', *, *, #9933, .T. ) ;
#7897=VECTOR ( 'NONE', #10137, 1000.000000000000000 ) ;
#7898=EDGE_CURVE ( 'NONE', #8100, #13349, #13034, .T. ) ;
#7899=CARTESIAN_POINT ( 'NONE',  ( -24.38380099443793725, -15.36048369738253427, 56.85231026484398598 ) ) ;
#7901=VECTOR ( 'NONE', #5468, 1000.000000000000000 ) ;
#7903=VECTOR ( 'NONE', #9348, 1000.000000000000227 ) ;
#7905=EDGE_CURVE ( 'NONE', #612, #5816, #100, .T. ) ;
#7906=DIRECTION ( 'NONE',  ( -8.018662683283438208E-16, 5.975035461963189015E-16, 1.000000000000000000 ) ) ;
#7908=VERTEX_POINT ( 'NONE', #1318 ) ;
#7909=DIRECTION ( 'NONE',  ( -8.018662683283438208E-16, 5.975035461963189015E-16, 1.000000000000000000 ) ) ;
#7913=CARTESIAN_POINT ( 'NONE',  ( -13.95777467540137806, -22.45074059323463089, 56.85231026484400019 ) ) ;
#7914=EDGE_CURVE ( 'NONE', #8039, #8731, #270, .T. ) ;
#7917=VECTOR ( 'NONE', #14919, 1000.000000000000000 ) ;
#7918=ORIENTED_EDGE ( 'NONE', *, *, #3271, .F. ) ;
#7919=CARTESIAN_POINT ( 'NONE',  ( -18.18846581869429713, -17.11577719991581148, -13.99768973515600301 ) ) ;
#7923=DIRECTION ( 'NONE',  ( 0.5975035461963189576, 0.8018662683283437342, 0.000000000000000000 ) ) ;
#7925=CARTESIAN_POINT ( 'NONE',  ( -6.426265323245524463, -13.69186664111786200, 56.85231026484400019 ) ) ;
#7926=ORIENTED_EDGE ( 'NONE', *, *, #9404, .T. ) ;
#7930=DIRECTION ( 'NONE',  ( -8.018662683283438208E-16, 5.975035461963189015E-16, 1.000000000000000000 ) ) ;
#7931=VECTOR ( 'NONE', #8110, 1000.000000000000114 ) ;
#7933=ORIENTED_EDGE ( 'NONE', *, *, #282, .F. ) ;
#7934=DIRECTION ( 'NONE',  ( 0.2872152572324145892, 0.9578660637129379207, -3.420201433256678811E-16 ) ) ;
#7935=ORIENTED_EDGE ( 'NONE', *, *, #5360, .T. ) ;
#7937=DIRECTION ( 'NONE',  ( 8.018662683283438208E-16, -5.975035461963189015E-16, -1.000000000000000000 ) ) ;
#7938=EDGE_CURVE ( 'NONE', #9010, #33, #12805, .T. ) ;
#7939=DIRECTION ( 'NONE',  ( 0.5975035461963189576, 0.8018662683283437342, 0.000000000000000000 ) ) ;
#7942=PLANE ( 'NONE',  #12872 ) ;
#7944=DIRECTION ( 'NONE',  ( 8.018662683283438208E-16, -5.975035461963189015E-16, -1.000000000000000000 ) ) ;
#7945=DIRECTION ( 'NONE',  ( -0.9225966037272106401, 0.3857661296576155863, -9.702957262759965065E-16 ) ) ;
#7948=ORIENTED_EDGE ( 'NONE', *, *, #14764, .T. ) ;
#7949=DIRECTION ( 'NONE',  ( 0.2301973227387160703, -0.9731439732146149879, 7.660444431189776467E-16 ) ) ;
#7950=FACE_OUTER_BOUND ( 'NONE', #9305, .T. ) ;
#7952=EDGE_LOOP ( 'NONE', ( #9292, #2381, #6622, #6298 ) ) ;
#7955=FACE_OUTER_BOUND ( 'NONE', #9789, .T. ) ;
#7957=EDGE_CURVE ( 'NONE', #11664, #3186, #4687, .T. ) ;
#7961=ORIENTED_EDGE ( 'NONE', *, *, #10998, .T. ) ;
#7963=EDGE_LOOP ( 'NONE', ( #12052, #1681, #721, #13717 ) ) ;
#7964=DIRECTION ( 'NONE',  ( -0.3857661296576155308, -0.9225966037272105291, 2.419218955996680478E-16 ) ) ;
#7968=EDGE_LOOP ( 'NONE', ( #8239, #4923, #7234, #7961 ) ) ;
#7969=CARTESIAN_POINT ( 'NONE',  ( -15.36741682587554969, -22.58172476492607572, 56.85231026484400019 ) ) ;
#7970=AXIS2_PLACEMENT_3D ( 'NONE', #11000, #9705, #8774 ) ;
#7971=EDGE_CURVE ( 'NONE', #4831, #1003, #14321, .T. ) ;
#7973=FACE_OUTER_BOUND ( 'NONE', #1833, .T. ) ;
#7980=DIRECTION ( 'NONE',  ( -0.7511640317997414495, -0.6601155939154573771, -2.079116908177570050E-16 ) ) ;
#7981=AXIS2_PLACEMENT_3D ( 'NONE', #6402, #14529, #10147 ) ;
#7984=ORIENTED_EDGE ( 'NONE', *, *, #12738, .T. ) ;
#7988=LINE ( 'NONE', #13896, #599 ) ;
#7990=CARTESIAN_POINT ( 'NONE',  ( -15.16333526000375187, -10.64029123852186132, 56.75231026484397745 ) ) ;
#7991=EDGE_CURVE ( 'NONE', #3619, #2590, #2465, .T. ) ;
#7993=VECTOR ( 'NONE', #13168, 999.9999999999998863 ) ;
#7994=CIRCLE ( 'NONE', #924, 9.974999999999999645 ) ;
#7998=LINE ( 'NONE', #2200, #10148 ) ;
#8000=VERTEX_POINT ( 'NONE', #2317 ) ;
#8005=VERTEX_POINT ( 'NONE', #11792 ) ;
#8010=CARTESIAN_POINT ( 'NONE',  ( -21.45979773411919922, -21.50599501901345434, 54.00231026484399166 ) ) ;
#8012=EDGE_CURVE ( 'NONE', #6877, #9544, #9498, .T. ) ;
#8013=CARTESIAN_POINT ( 'NONE',  ( -21.24026693782044717, -7.828337292084670551, 57.00231026484397745 ) ) ;
#8015=AXIS2_PLACEMENT_3D ( 'NONE', #12895, #4705, #4781 ) ;
#8019=VECTOR ( 'NONE', #6973, 1000.000000000000000 ) ;
#8020=LINE ( 'NONE', #5731, #14615 ) ;
#8021=ADVANCED_FACE ( 'NONE', ( #14247 ), #3764, .T. ) ;
#8026=LINE ( 'NONE', #14, #6898 ) ;
#8029=ORIENTED_EDGE ( 'NONE', *, *, #5788, .T. ) ;
#8031=CARTESIAN_POINT ( 'NONE',  ( -15.49969986081092088, -13.50737899243822504, 56.85231026484398598 ) ) ;
#8034=EDGE_CURVE ( 'NONE', #5981, #5306, #14544, .T. ) ;
#8035=EDGE_CURVE ( 'NONE', #7250, #10194, #6344, .T. ) ;
#8036=CARTESIAN_POINT ( 'NONE',  ( -12.84086554789186607, -5.882298658668338120, 56.85231026484398598 ) ) ;
#8038=VECTOR ( 'NONE', #58, 1000.000000000000000 ) ;
#8039=VERTEX_POINT ( 'NONE', #4061 ) ;
#8041=ORIENTED_EDGE ( 'NONE', *, *, #11773, .F. ) ;
#8044=CARTESIAN_POINT ( 'NONE',  ( -19.45253106704483770, -6.466019006254929202, 56.85231026484398598 ) ) ;
#8045=ORIENTED_EDGE ( 'NONE', *, *, #7126, .F. ) ;
#8048=ORIENTED_EDGE ( 'NONE', *, *, #4995, .T. ) ;
#8050=EDGE_CURVE ( 'NONE', #5847, #9327, #7578, .T. ) ;
#8051=DIRECTION ( 'NONE',  ( 0.3633925226508256667, -0.9316361277244830097, 8.480480961564259036E-16 ) ) ;
#8053=AXIS2_PLACEMENT_3D ( 'NONE', #14559, #494, #5148 ) ;
#8054=CARTESIAN_POINT ( 'NONE',  ( -7.785174720008381399, -8.727488632615573394, 56.85231026484400019 ) ) ;
#8055=DIRECTION ( 'NONE',  ( 0.5975035461963188466, 0.8018662683283437342, 0.000000000000000000 ) ) ;
#8057=ORIENTED_EDGE ( 'NONE', *, *, #6921, .F. ) ;
#8059=DIRECTION ( 'NONE',  ( -0.9826409426582665141, 0.1855175943453169496, -8.987940462991673516E-16 ) ) ;
#8064=VECTOR ( 'NONE', #1612, 1000.000000000000000 ) ;
#8065=DIRECTION ( 'NONE',  ( 0.5975035461963189576, 0.8018662683283437342, 0.000000000000000000 ) ) ;
#8068=DIRECTION ( 'NONE',  ( 0.9645173894937585368, 0.2640193276336892936, 6.156614753256587028E-16 ) ) ;
#8069=FACE_OUTER_BOUND ( 'NONE', #4524, .T. ) ;
#8070=CARTESIAN_POINT ( 'NONE',  ( -22.56723502526082470, -13.84084068328822248, 56.85231026484398598 ) ) ;
#8073=VERTEX_POINT ( 'NONE', #544 ) ;
#8075=LINE ( 'NONE', #5785, #909 ) ;
#8076=CARTESIAN_POINT ( 'NONE',  ( -17.95685260396766125, -23.17500669507537836, 57.00231026484399166 ) ) ;
#8078=CARTESIAN_POINT ( 'NONE',  ( -21.17290370923395670, -9.280041403099277275, 57.00231026484397745 ) ) ;
#8079=ORIENTED_EDGE ( 'NONE', *, *, #2874, .T. ) ;
#8081=ORIENTED_EDGE ( 'NONE', *, *, #7255, .T. ) ;
#8083=DIRECTION ( 'NONE',  ( 0.5975035461963188466, 0.8018662683283438453, 0.000000000000000000 ) ) ;
#8084=DIRECTION ( 'NONE',  ( -0.5401126942952660936, -0.8415927028326163351, 6.975647374412055055E-17 ) ) ;
#8086=CARTESIAN_POINT ( 'NONE',  ( -13.01672903104007872, -13.79867928167105440, 51.00231026484399166 ) ) ;
#8087=CARTESIAN_POINT ( 'NONE',  ( -21.79367780933653620, -21.24601366423100401, 56.85231026484398598 ) ) ;
#8088=VECTOR ( 'NONE', #1246, 1000.000000000000114 ) ;
#8089=AXIS2_PLACEMENT_3D ( 'NONE', #1601, #6606, #13518 ) ;
#8090=CARTESIAN_POINT ( 'NONE',  ( -20.65541546412893936, -22.04665423204160035, 57.00231026484397745 ) ) ;
#8091=DIRECTION ( 'NONE',  ( 0.9183863840214729901, 0.3956847857120157075, 4.999999999999999402E-16 ) ) ;
#8092=CARTESIAN_POINT ( 'NONE',  ( -13.18491133144367389, -15.23222315862922827, 51.00231026484399166 ) ) ;
#8095=PLANE ( 'NONE',  #530 ) ;
#8097=CARTESIAN_POINT ( 'NONE',  ( -24.85752488709640673, -10.05314452190415331, 56.85231026484398598 ) ) ;
#8100=VERTEX_POINT ( 'NONE', #3912 ) ;
#8101=DIRECTION ( 'NONE',  ( -0.9826409426582659590, 0.1855175943453191978, -8.987940462991681405E-16 ) ) ;
#8103=VECTOR ( 'NONE', #1192, 1000.000000000000000 ) ;
#8104=FACE_OUTER_BOUND ( 'NONE', #2209, .T. ) ;
#8106=AXIS2_PLACEMENT_3D ( 'NONE', #10240, #3208, #764 ) ;
#8110=DIRECTION ( 'NONE',  ( 0.4895147004624045839, -0.8719950447285823580, 9.135454576426008610E-16 ) ) ;
#8116=EDGE_CURVE ( 'NONE', #13227, #14849, #6268, .T. ) ;
#8120=ORIENTED_EDGE ( 'NONE', *, *, #2797, .F. ) ;
#8121=DIRECTION ( 'NONE',  ( 0.5975035461963188466, 0.8018662683283437342, 0.000000000000000000 ) ) ;
#8127=CARTESIAN_POINT ( 'NONE',  ( -7.528759897616733809, -14.80173833325270571, 56.85231026484400019 ) ) ;
#8131=CARTESIAN_POINT ( 'NONE',  ( -9.760873592531984499, -5.348549538251087476, 54.00231026484399166 ) ) ;
#8134=CARTESIAN_POINT ( 'NONE',  ( -24.08903783298838519, -16.43731469134198520, 57.00231026484397745 ) ) ;
#8136=ORIENTED_EDGE ( 'NONE', *, *, #8594, .F. ) ;
#8137=PLANE ( 'NONE',  #15095 ) ;
#8138=EDGE_CURVE ( 'NONE', #532, #7723, #10915, .T. ) ;
#8139=EDGE_CURVE ( 'NONE', #2792, #4546, #2987, .T. ) ;
#8140=FACE_OUTER_BOUND ( 'NONE', #2778, .T. ) ;
#8141=ORIENTED_EDGE ( 'NONE', *, *, #10463, .F. ) ;
#8144=VECTOR ( 'NONE', #14371, 999.9999999999998863 ) ;
#8148=EDGE_LOOP ( 'NONE', ( #12489, #14777, #12496, #12792 ) ) ;
#8149=VECTOR ( 'NONE', #10387, 1000.000000000000227 ) ;
#8150=CARTESIAN_POINT ( 'NONE',  ( -20.19618812003464470, -21.27295997720514720, 56.85231026484398598 ) ) ;
#8153=VECTOR ( 'NONE', #5293, 1000.000000000000000 ) ;
#8155=CARTESIAN_POINT ( 'NONE',  ( -13.72291223624743317, -3.691898834178107602, 57.00231026484397745 ) ) ;
#8156=CARTESIAN_POINT ( 'NONE',  ( -7.285742840713465007, -17.36641515085804599, 57.00231026484399166 ) ) ;
#8159=CARTESIAN_POINT ( 'NONE',  ( -17.81448839017816965, -11.78253482624722004, 56.75231026484397745 ) ) ;
#8162=LINE ( 'NONE', #7649, #230 ) ;
#8163=ORIENTED_EDGE ( 'NONE', *, *, #619, .T. ) ;
#8164=CARTESIAN_POINT ( 'NONE',  ( -17.72867398697626129, -22.30470383268854562, 56.85231026484400019 ) ) ;
#8166=CARTESIAN_POINT ( 'NONE',  ( -7.499849062438288527, -12.40572695854698360, 56.85231026484400019 ) ) ;
#8168=CARTESIAN_POINT ( 'NONE',  ( -9.291286065451622278, -6.887949398765353060, 56.85231026484398598 ) ) ;
#8169=CARTESIAN_POINT ( 'NONE',  ( -18.48721759179251123, -17.51671033407994926, 54.00231026484399166 ) ) ;
#8173=DIRECTION ( 'NONE',  ( 8.018662683283438208E-16, -5.975035461963189015E-16, -1.000000000000000000 ) ) ;
#8174=CARTESIAN_POINT ( 'NONE',  ( -13.92794721577312878, -5.586467200048621073, 56.85231026484398598 ) ) ;
#8176=DIRECTION ( 'NONE',  ( -0.9040177279761104634, -0.4274949678123838859, -4.694715627858909121E-16 ) ) ;
#8177=VERTEX_POINT ( 'NONE', #4367 ) ;
#8178=DIRECTION ( 'NONE',  ( 0.5975035461963189576, 0.8018662683283437342, 0.000000000000000000 ) ) ;
#8182=EDGE_LOOP ( 'NONE', ( #247, #10295, #7137, #7948 ) ) ;
#8184=PLANE ( 'NONE',  #10685 ) ;
#8185=ORIENTED_EDGE ( 'NONE', *, *, #10616, .F. ) ;
#8189=DIRECTION ( 'NONE',  ( 8.018662683283438208E-16, -5.975035461963189015E-16, -1.000000000000000000 ) ) ;
#8199=FACE_OUTER_BOUND ( 'NONE', #7354, .T. ) ;
#8200=ORIENTED_EDGE ( 'NONE', *, *, #5275, .T. ) ;
#8202=DIRECTION ( 'NONE',  ( -8.018662683283438208E-16, 5.975035461963189015E-16, 1.000000000000000000 ) ) ;
#8204=FACE_OUTER_BOUND ( 'NONE', #54, .T. ) ;
#8207=DIRECTION ( 'NONE',  ( -0.9918751611018171710, -0.1272150336605075427, -7.193398003386516820E-16 ) ) ;
#8208=CIRCLE ( 'NONE', #2360, 9.974999999999999645 ) ;
#8211=DIRECTION ( 'NONE',  ( -0.9437508163134049610, -0.3306575217771128283, -5.591929034707468788E-16 ) ) ;
#8214=DIRECTION ( 'NONE',  ( -0.9547156899063192759, -0.2975196656469966672, -5.877852522924767272E-16 ) ) ;
#8217=EDGE_CURVE ( 'NONE', #4500, #1475, #4518, .T. ) ;
#8218=ORIENTED_EDGE ( 'NONE', *, *, #10942, .F. ) ;
#8221=VECTOR ( 'NONE', #4118, 1000.000000000000227 ) ;
#8222=VERTEX_POINT ( 'NONE', #2219 ) ;
#8224=EDGE_LOOP ( 'NONE', ( #14997, #4237, #14793, #13788 ) ) ;
#8226=EDGE_CURVE ( 'NONE', #9490, #6457, #9095, .T. ) ;
#8228=EDGE_CURVE ( 'NONE', #1568, #11735, #7789, .T. ) ;
#8229=VECTOR ( 'NONE', #8308, 1000.000000000000000 ) ;
#8234=ORIENTED_EDGE ( 'NONE', *, *, #1574, .F. ) ;
#8236=CARTESIAN_POINT ( 'NONE',  ( -24.01584079503567182, -10.37104457333969876, 56.85231026484398598 ) ) ;
#8238=LINE ( 'NONE', #1584, #10980 ) ;
#8239=ORIENTED_EDGE ( 'NONE', *, *, #3814, .T. ) ;
#8243=DIRECTION ( 'NONE',  ( 0.5975035461963189576, 0.8018662683283437342, 0.000000000000000000 ) ) ;
#8244=AXIS2_PLACEMENT_3D ( 'NONE', #14602, #1829, #757 ) ;
#8246=CARTESIAN_POINT ( 'NONE',  ( -8.663330333365388825, -17.80566954616001496, 56.85231026484400019 ) ) ;
#8250=FACE_OUTER_BOUND ( 'NONE', #14548, .T. ) ;
#8251=LINE ( 'NONE', #13925, #11433 ) ;
#8252=CARTESIAN_POINT ( 'NONE',  ( -17.40065610530428586, -5.145404622917534532, 56.85231026484398598 ) ) ;
#8254=VERTEX_POINT ( 'NONE', #3293 ) ;
#8255=CARTESIAN_POINT ( 'NONE',  ( -18.68395610307571530, -20.92841410781112899, 56.85231026484398598 ) ) ;
#8256=VERTEX_POINT ( 'NONE', #7862 ) ;
#8258=ORIENTED_EDGE ( 'NONE', *, *, #2655, .T. ) ;
#8259=ORIENTED_EDGE ( 'NONE', *, *, #12178, .T. ) ;
#8260=EDGE_CURVE ( 'NONE', #11198, #3205, #11249, .T. ) ;
#8261=CARTESIAN_POINT ( 'NONE',  ( -18.54556661251663385, -20.98627902725976568, 57.00231026484397745 ) ) ;
#8262=ORIENTED_EDGE ( 'NONE', *, *, #12043, .F. ) ;
#8263=VECTOR ( 'NONE', #13731, 1000.000000000000114 ) ;
#8264=LINE ( 'NONE', #12957, #13808 ) ;
#8265=AXIS2_PLACEMENT_3D ( 'NONE', #5327, #4335, #7685 ) ;
#8266=DIRECTION ( 'NONE',  ( 0.9983330752162417054, 0.05771543059946734194, 7.660444431189781397E-16 ) ) ;
#8267=DIRECTION ( 'NONE',  ( 0.5975035461963189576, 0.8018662683283437342, 0.000000000000000000 ) ) ;
#8274=ORIENTED_EDGE ( 'NONE', *, *, #3359, .F. ) ;
#8275=CARTESIAN_POINT ( 'NONE',  ( -22.53804163936502647, -6.438972523632135569, 56.85231026484398598 ) ) ;
#8277=CLOSED_SHELL ( 'NONE', ( #1288, #1873, #7207, #1034, #2296, #8382, #11476, #3152, #11030, #1916, #829, #13769, #10196, #9425, #13848, #758, #13370, #10480, #2102, #12541, #15101, #10283, #14219, #11122, #11317, #11766, #8662, #1915, #8302, #6616, #11844, #4981, #10107, #1707, #8414, #653, #14010, #8863, #10048, #10751, #1972, #10401, #7786, #8021, #3865, #13039, #955, #3850, #6324, #12349, #5756, #2624, #4876, #10834, #11431, #12061, #9771, #11600, #5872, #2087, #13211, #5969, #4264, #5834, #4472, #2900, #9105, #14211, #5669, #12341, #9993, #1035, #2467, #1304, #1846, #8401, #1360, #9788, #13493, #6935, #10121, #15000, #11971, #12446, #3174, #2420, #10004, #2270, #10157, #11012, #3363, #1766, #11583, #11211, #10264, #9722, #4158, #12437, #132, #3586, #11794, #14373, #1861, #10073, #14558, #7005, #6883, #7497, #4282, #10375, #3767, #6468, #6303, #5099, #7695, #13654, #11604, #4665, #284, #2726, #12538, #3207, #12354, #10511, #4299, #5243, #2436, #14656, #3449, #9228, #8571, #4971, #1269, #6199, #12736, #7731, #13805, #7084, #7515, #3418, #8510, #13869, #5484, #13208, #833, #10154, #3550, #10949, #12064, #14680, #6786, #5709, #9267, #7414, #3553, #4493, #11132, #12592, #11208, #14509, #14946, #10881, #6234, #6149, #12765, #14323, #473, #13621, #11227, #6807, #11518, #1757, #3725, #6713, #3400, #12723, #1214, #13831, #8985, #25, #2207, #2499, #635, #13766, #7516, #14618, #12216, #11390, #4026, #9905, #15123, #3554, #13019, #2239, #4474, #13506, #13355, #9336, #6765, #2426, #7313, #1181, #6130, #7633, #9654, #10740, #1448, #11989, #11783, #1347, #4368, #7466, #3924, #7604, #7775, #14069, #13919, #6075 ) ) ;
#8279=ORIENTED_EDGE ( 'NONE', *, *, #5430, .F. ) ;
#8285=DIRECTION ( 'NONE',  ( 0.3956847857120156520, -0.9183863840214728791, 8.660254037844387408E-16 ) ) ;
#8290=LINE ( 'NONE', #7139, #13767 ) ;
#8291=VERTEX_POINT ( 'NONE', #12476 ) ;
#8293=VERTEX_POINT ( 'NONE', #10323 ) ;
#8296=ORIENTED_EDGE ( 'NONE', *, *, #15055, .T. ) ;
#8298=EDGE_CURVE ( 'NONE', #2388, #2863, #1070, .T. ) ;
#8300=DIRECTION ( 'NONE',  ( -0.9547156899063178326, -0.2975196656470014966, -5.877852522924727828E-16 ) ) ;
#8301=DIRECTION ( 'NONE',  ( -8.018662683283438208E-16, 5.975035461963189015E-16, 1.000000000000000000 ) ) ;
#8302=ADVANCED_FACE ( 'NONE', ( #10089 ), #14689, .F. ) ;
#8303=PLANE ( 'NONE',  #14319 ) ;
#8304=PLANE ( 'NONE',  #7882 ) ;
#8308=DIRECTION ( 'NONE',  ( -8.018662683283438208E-16, 5.975035461963189015E-16, 1.000000000000000000 ) ) ;
#8309=ORIENTED_EDGE ( 'NONE', *, *, #6536, .T. ) ;
#8312=EDGE_CURVE ( 'NONE', #6022, #3165, #3744, .T. ) ;
#8313=ORIENTED_EDGE ( 'NONE', *, *, #4404, .T. ) ;
#8314=CARTESIAN_POINT ( 'NONE',  ( -20.69940085690220144, -18.30574950243923027, 56.85231026484398598 ) ) ;
#8316=DIRECTION ( 'NONE',  ( 0.5975035461963188466, 0.8018662683283437342, 0.000000000000000000 ) ) ;
#8320=CARTESIAN_POINT ( 'NONE',  ( -24.80452494096261518, -9.912819877918103373, 54.00231026484397745 ) ) ;
#8322=CARTESIAN_POINT ( 'NONE',  ( -8.722797460041883610, -15.53942693735753444, 56.85231026484400019 ) ) ;
#8324=VERTEX_POINT ( 'NONE', #4820 ) ;
#8325=CARTESIAN_POINT ( 'NONE',  ( -12.81093390292742740, -9.898980784960722090, -13.99768973515600301 ) ) ;
#8326=CARTESIAN_POINT ( 'NONE',  ( -15.26225645643175710, -10.41069464251649279, 57.00231026484397745 ) ) ;
#8327=VECTOR ( 'NONE', #7664, 1000.000000000000227 ) ;
#8330=CARTESIAN_POINT ( 'NONE',  ( -15.49969986081092088, -13.50737899243822504, 56.85231026484398598 ) ) ;
#8333=ORIENTED_EDGE ( 'NONE', *, *, #7957, .F. ) ;
#8334=LINE ( 'NONE', #1228, #2280 ) ;
#8336=ORIENTED_EDGE ( 'NONE', *, *, #4397, .F. ) ;
#8338=EDGE_CURVE ( 'NONE', #8291, #13071, #4590, .T. ) ;
#8339=CARTESIAN_POINT ( 'NONE',  ( -19.68577560955674954, -20.41303028871448788, 56.85231026484398598 ) ) ;
#8340=ORIENTED_EDGE ( 'NONE', *, *, #11548, .T. ) ;
#8342=CARTESIAN_POINT ( 'NONE',  ( -12.52039621090187893, -4.935039769003430443, 57.00231026484397745 ) ) ;
#8343=AXIS2_PLACEMENT_3D ( 'NONE', #9642, #2603, #14662 ) ;
#8344=CARTESIAN_POINT ( 'NONE',  ( -12.38873450203231030, -7.152605626181999909, 57.00231026484397745 ) ) ;
#8347=EDGE_CURVE ( 'NONE', #221, #12795, #10547, .T. ) ;
#8348=CARTESIAN_POINT ( 'NONE',  ( -8.681233859935401753, -6.226640953275941470, 57.00231026484397745 ) ) ;
#8349=AXIS2_PLACEMENT_3D ( 'NONE', #4167, #3944, #8672 ) ;
#8350=DIRECTION ( 'NONE',  ( 0.5975035461963188466, 0.8018662683283437342, 0.000000000000000000 ) ) ;
#8352=CARTESIAN_POINT ( 'NONE',  ( -15.49969986081092088, -13.50737899243822504, 56.85231026484398598 ) ) ;
#8353=VERTEX_POINT ( 'NONE', #1138 ) ;
#8354=ORIENTED_EDGE ( 'NONE', *, *, #3690, .T. ) ;
#8355=VECTOR ( 'NONE', #5845, 1000.000000000000000 ) ;
#8356=AXIS2_PLACEMENT_3D ( 'NONE', #1974, #8845, #10066 ) ;
#8358=VERTEX_POINT ( 'NONE', #13086 ) ;
#8361=DIRECTION ( 'NONE',  ( 0.08178736187251967049, 0.9966498018049938512, -5.299192642332049884E-16 ) ) ;
#8362=EDGE_CURVE ( 'NONE', #5856, #4847, #11929, .T. ) ;
#8367=ORIENTED_EDGE ( 'NONE', *, *, #2248, .T. ) ;
#8368=CARTESIAN_POINT ( 'NONE',  ( -14.60940909295887913, -15.57374835648654532, 51.25231026484399166 ) ) ;
#8371=ORIENTED_EDGE ( 'NONE', *, *, #14054, .T. ) ;
#8376=CARTESIAN_POINT ( 'NONE',  ( -20.44787060326519423, -4.846187890544671362, 57.00231026484397745 ) ) ;
#8377=EDGE_CURVE ( 'NONE', #551, #1781, #11343, .T. ) ;
#8379=CIRCLE ( 'NONE', #5947, 9.974999999999999645 ) ;
#8381=LINE ( 'NONE', #3876, #9607 ) ;
#8382=ADVANCED_FACE ( 'NONE', ( #9477 ), #8712, .T. ) ;
#8383=ORIENTED_EDGE ( 'NONE', *, *, #9529, .T. ) ;
#8385=CARTESIAN_POINT ( 'NONE',  ( -22.80943503306989584, -20.29474937510043731, 57.00231026484397745 ) ) ;
#8387=DIRECTION ( 'NONE',  ( 8.018662683283438208E-16, -5.975035461963189015E-16, -1.000000000000000000 ) ) ;
#8390=FACE_OUTER_BOUND ( 'NONE', #14238, .T. ) ;
#8391=VERTEX_POINT ( 'NONE', #8087 ) ;
#8392=CARTESIAN_POINT ( 'NONE',  ( -15.49969986081092088, -13.50737899243822504, 56.85231026484398598 ) ) ;
#8395=CARTESIAN_POINT ( 'NONE',  ( -10.90377457632059865, -6.867868786151726468, 57.00231026484397745 ) ) ;
#8397=CARTESIAN_POINT ( 'NONE',  ( -11.61446667642527331, -19.42012692406430574, 57.00231026484399166 ) ) ;
#8399=EDGE_CURVE ( 'NONE', #13135, #8450, #2373, .T. ) ;
#8401=ADVANCED_FACE ( 'NONE', ( #15064 ), #2595, .T. ) ;
#8402=AXIS2_PLACEMENT_3D ( 'NONE', #1564, #11043, #1491 ) ;
#8404=EDGE_CURVE ( 'NONE', #12566, #2877, #11695, .T. ) ;
#8409=ORIENTED_EDGE ( 'NONE', *, *, #5275, .F. ) ;
#8410=FACE_OUTER_BOUND ( 'NONE', #7020, .T. ) ;
#8411=ORIENTED_EDGE ( 'NONE', *, *, #4106, .T. ) ;
#8412=CARTESIAN_POINT ( 'NONE',  ( -13.96026682931439034, -23.36287344688023992, 54.00231026484399166 ) ) ;
#8413=ORIENTED_EDGE ( 'NONE', *, *, #11703, .T. ) ;
#8414=ADVANCED_FACE ( 'NONE', ( #1449 ), #10397, .F. ) ;
#8417=ORIENTED_EDGE ( 'NONE', *, *, #2725, .T. ) ;
#8419=CARTESIAN_POINT ( 'NONE',  ( -10.02446058099324588, -7.572113216692248017, 56.85231026484398598 ) ) ;
#8420=VECTOR ( 'NONE', #12784, 1000.000000000000000 ) ;
#8421=EDGE_CURVE ( 'NONE', #1793, #14007, #14340, .T. ) ;
#8426=CARTESIAN_POINT ( 'NONE',  ( -8.744347237509680681, -17.93190845158491342, 56.85231026484400019 ) ) ;
#8429=ORIENTED_EDGE ( 'NONE', *, *, #2978, .F. ) ;
#8430=DIRECTION ( 'NONE',  ( 0.4895147004624045839, -0.8719950447285823580, 9.135454576426008610E-16 ) ) ;
#8431=CARTESIAN_POINT ( 'NONE',  ( -9.328067836852527606, -18.71527762440592468, 56.85231026484400019 ) ) ;
#8436=EDGE_LOOP ( 'NONE', ( #12868, #14084, #8120, #14963 ) ) ;
#8438=CARTESIAN_POINT ( 'NONE',  ( -8.430459378593662123, -7.816413432484393020, 56.85231026484400019 ) ) ;
#8439=EDGE_CURVE ( 'NONE', #9717, #10845, #6244, .T. ) ;
#8441=CARTESIAN_POINT ( 'NONE',  ( -15.49969986081092088, -13.50737899243822504, 57.00231026484397745 ) ) ;
#8444=DIRECTION ( 'NONE',  ( 8.018662683283438208E-16, -5.975035461963189015E-16, -1.000000000000000000 ) ) ;
#8445=LINE ( 'NONE', #9370, #695 ) ;
#8448=CARTESIAN_POINT ( 'NONE',  ( -15.73714326519009354, -16.60406334235995018, 57.00231026484397745 ) ) ;
#8450=VERTEX_POINT ( 'NONE', #5262 ) ;
#8452=LINE ( 'NONE', #5997, #14711 ) ;
#8456=EDGE_CURVE ( 'NONE', #964, #13913, #2671, .T. ) ;
#8458=CARTESIAN_POINT ( 'NONE',  ( -15.49969986081092088, -13.50737899243822504, 56.85231026484398598 ) ) ;
#8465=CARTESIAN_POINT ( 'NONE',  ( -25.46211945451987191, -14.00819915864900977, 54.00231026484397745 ) ) ;
#8466=VERTEX_POINT ( 'NONE', #524 ) ;
#8472=DIRECTION ( 'NONE',  ( 8.018662683283438208E-16, -5.975035461963189015E-16, -1.000000000000000000 ) ) ;
#8474=CARTESIAN_POINT ( 'NONE',  ( -10.07958688850791162, -7.521259601090221736, 57.00231026484397745 ) ) ;
#8476=VECTOR ( 'NONE', #1374, 1000.000000000000000 ) ;
#8479=CARTESIAN_POINT ( 'NONE',  ( -15.49969986081091378, -13.50737899243822859, 51.00231026484399166 ) ) ;
#8483=CARTESIAN_POINT ( 'NONE',  ( -15.31527533914055539, -21.58027268651140673, 57.00231026484399166 ) ) ;
#8485=CARTESIAN_POINT ( 'NONE',  ( -21.21771647519868154, -9.340181373223902739, 57.00231026484397745 ) ) ;
#8487=CARTESIAN_POINT ( 'NONE',  ( -17.81448839017817320, -11.78253482624721116, 56.89875687425070794 ) ) ;
#8488=ORIENTED_EDGE ( 'NONE', *, *, #9684, .T. ) ;
#8489=VERTEX_POINT ( 'NONE', #14301 ) ;
#8491=CARTESIAN_POINT ( 'NONE',  ( -18.23096777355884157, -13.18694867428211914, 56.75231026484397745 ) ) ;
#8492=LINE ( 'NONE', #6481, #9992 ) ;
#8493=EDGE_CURVE ( 'NONE', #5861, #9932, #4044, .T. ) ;
#8494=CARTESIAN_POINT ( 'NONE',  ( -21.45979773411919567, -21.50599501901345789, 48.00231026484398456 ) ) ;
#8496=DIRECTION ( 'NONE',  ( 8.018662683283438208E-16, -5.975035461963189015E-16, -1.000000000000000000 ) ) ;
#8499=DIRECTION ( 'NONE',  ( -0.3956847857120157075, 0.9183863840214729901, -8.660254037844387408E-16 ) ) ;
#8500=VECTOR ( 'NONE', #8981, 1000.000000000000000 ) ;
#8506=ORIENTED_EDGE ( 'NONE', *, *, #1396, .F. ) ;
#8509=DIRECTION ( 'NONE',  ( -8.018662683283438208E-16, 5.975035461963189015E-16, 1.000000000000000000 ) ) ;
#8510=ADVANCED_FACE ( 'NONE', ( #671 ), #4268, .F. ) ;
#8512=EDGE_LOOP ( 'NONE', ( #1274, #11958, #8969, #2489 ) ) ;
#8513=PLANE ( 'NONE',  #14725 ) ;
#8515=PLANE ( 'NONE',  #2891 ) ;
#8518=CARTESIAN_POINT ( 'NONE',  ( -9.565488148413145097, -20.37370125056455095, 57.00231026484399166 ) ) ;
#8524=CARTESIAN_POINT ( 'NONE',  ( -20.54757852167729837, -19.81012014412530320, 56.85231026484398598 ) ) ;
#8527=EDGE_CURVE ( 'NONE', #7429, #8707, #6697, .T. ) ;
#8529=VECTOR ( 'NONE', #6928, 1000.000000000000000 ) ;
#8533=FACE_OUTER_BOUND ( 'NONE', #9236, .T. ) ;
#8542=FACE_OUTER_BOUND ( 'NONE', #14934, .T. ) ;
#8545=VERTEX_POINT ( 'NONE', #14972 ) ;
#8547=EDGE_LOOP ( 'NONE', ( #6277, #10506, #3801, #4412 ) ) ;
#8548=DIRECTION ( 'NONE',  ( 0.5975035461963189576, 0.8018662683283437342, 0.000000000000000000 ) ) ;
#8555=LINE ( 'NONE', #10498, #1333 ) ;
#8558=DIRECTION ( 'NONE',  ( -0.5975035461963187355, -0.8018662683283439563, 0.000000000000000000 ) ) ;
#8559=ORIENTED_EDGE ( 'NONE', *, *, #4190, .F. ) ;
#8560=CARTESIAN_POINT ( 'NONE',  ( -15.49969986081092088, -13.50737899243822504, 56.85231026484398598 ) ) ;
#8561=VERTEX_POINT ( 'NONE', #4496 ) ;
#8563=ORIENTED_EDGE ( 'NONE', *, *, #1394, .T. ) ;
#8564=VERTEX_POINT ( 'NONE', #12378 ) ;
#8565=DIRECTION ( 'NONE',  ( -8.018662683283438208E-16, 5.975035461963189015E-16, 1.000000000000000000 ) ) ;
#8566=CARTESIAN_POINT ( 'NONE',  ( -15.10625462230756177, -3.540141368888813922, 57.00231026484397745 ) ) ;
#8567=DIRECTION ( 'NONE',  ( 8.018662683283438208E-16, -5.975035461963189015E-16, -1.000000000000000000 ) ) ;
#8571=ADVANCED_FACE ( 'NONE', ( #4348 ), #1898, .T. ) ;
#8572=LINE ( 'NONE', #2768, #5787 ) ;
#8575=LINE ( 'NONE', #5286, #7108 ) ;
#8576=ORIENTED_EDGE ( 'NONE', *, *, #10942, .T. ) ;
#8577=CARTESIAN_POINT ( 'NONE',  ( -22.13265177292497299, -18.11337496850924822, 57.00231026484397745 ) ) ;
#8580=LINE ( 'NONE', #2777, #307 ) ;
#8581=ORIENTED_EDGE ( 'NONE', *, *, #10140, .F. ) ;
#8583=DIRECTION ( 'NONE',  ( 0.5975035461963189576, 0.8018662683283437342, 0.000000000000000000 ) ) ;
#8584=DIRECTION ( 'NONE',  ( -8.018662683283439195E-16, 5.975035461963190001E-16, 1.000000000000000000 ) ) ;
#8585=DIRECTION ( 'NONE',  ( 0.6780482080269577549, 0.7350174335289139105, 1.045284632676540317E-16 ) ) ;
#8586=EDGE_CURVE ( 'NONE', #5325, #12427, #13604, .T. ) ;
#8588=EDGE_CURVE ( 'NONE', #13854, #8833, #10143, .T. ) ;
#8589=CIRCLE ( 'NONE', #3214, 5.000000000000000000 ) ;
#8590=CARTESIAN_POINT ( 'NONE',  ( -24.08903783298838519, -16.43731469134198520, 56.85231026484398598 ) ) ;
#8593=DIRECTION ( 'NONE',  ( -8.018662683283438208E-16, 5.975035461963189015E-16, 1.000000000000000000 ) ) ;
#8594=EDGE_CURVE ( 'NONE', #9544, #12009, #3342, .T. ) ;
#8596=CARTESIAN_POINT ( 'NONE',  ( -9.291286065451622278, -6.887949398765353060, 56.85231026484398598 ) ) ;
#8597=ORIENTED_EDGE ( 'NONE', *, *, #11908, .F. ) ;
#8601=DIRECTION ( 'NONE',  ( 8.018662683283438208E-16, -5.975035461963189015E-16, -1.000000000000000000 ) ) ;
#8602=DIRECTION ( 'NONE',  ( 0.8543800322332385511, 0.5196486895212286683, 3.746065934159130275E-16 ) ) ;
#8604=EDGE_CURVE ( 'NONE', #4315, #4372, #1823, .T. ) ;
#8605=AXIS2_PLACEMENT_3D ( 'NONE', #13451, #12449, #2956 ) ;
#8606=VECTOR ( 'NONE', #471, 1000.000000000000114 ) ;
#8607=AXIS2_PLACEMENT_3D ( 'NONE', #13454, #13233, #1736 ) ;
#8608=AXIS2_PLACEMENT_3D ( 'NONE', #9401, #9166, #7939 ) ;
#8613=LINE ( 'NONE', #7458, #14265 ) ;
#8614=ORIENTED_EDGE ( 'NONE', *, *, #6443, .T. ) ;
#8615=LINE ( 'NONE', #9913, #10682 ) ;
#8618=CARTESIAN_POINT ( 'NONE',  ( -15.47224238247604511, -13.54916519690201149, 56.85231026484398598 ) ) ;
#8619=ORIENTED_EDGE ( 'NONE', *, *, #9684, .F. ) ;
#8624=CARTESIAN_POINT ( 'NONE',  ( -17.87376992080280758, -22.26666214519964271, 56.85231026484400019 ) ) ;
#8626=CARTESIAN_POINT ( 'NONE',  ( -15.49969986081092088, -13.50737899243822504, 57.00231026484397745 ) ) ;
#8631=VECTOR ( 'NONE', #12746, 1000.000000000000114 ) ;
#8633=DIRECTION ( 'NONE',  ( -8.018662683283438208E-16, 5.975035461963189015E-16, 1.000000000000000000 ) ) ;
#8636=CARTESIAN_POINT ( 'NONE',  ( -16.49725497239786520, -3.582384846377123733, 57.00231026484397745 ) ) ;
#8638=VERTEX_POINT ( 'NONE', #8325 ) ;
#8639=CARTESIAN_POINT ( 'NONE',  ( -12.81093390292747536, -9.898980784960686563, 46.00231026484398456 ) ) ;
#8642=VECTOR ( 'NONE', #10371, 1000.000000000000114 ) ;
#8643=LINE ( 'NONE', #13251, #1611 ) ;
#8645=EDGE_CURVE ( 'NONE', #5527, #9881, #6099, .T. ) ;
#8646=DIRECTION ( 'NONE',  ( -8.018662683283438208E-16, 5.975035461963189015E-16, 1.000000000000000000 ) ) ;
#8649=AXIS2_PLACEMENT_3D ( 'NONE', #1670, #2894, #9784 ) ;
#8650=CARTESIAN_POINT ( 'NONE',  ( -14.10579935493720782, -22.47500361547664127, 56.85231026484400019 ) ) ;
#8651=ORIENTED_EDGE ( 'NONE', *, *, #12141, .T. ) ;
#8652=DIRECTION ( 'NONE',  ( -0.9183863840214729901, -0.3956847857120157075, -4.999999999999999402E-16 ) ) ;
#8655=AXIS2_PLACEMENT_3D ( 'NONE', #3631, #8285, #4863 ) ;
#8657=ORIENTED_EDGE ( 'NONE', *, *, #11956, .T. ) ;
#8662=ADVANCED_FACE ( 'NONE', ( #8250 ), #9786, .T. ) ;
#8664=CARTESIAN_POINT ( 'NONE',  ( -7.654212976755197850, -10.04550297615607768, 56.85231026484400019 ) ) ;
#8671=EDGE_LOOP ( 'NONE', ( #891, #10424, #14831, #14241 ) ) ;
#8672=DIRECTION ( 'NONE',  ( -0.8885476655824650072, -0.4587843131450243805, -4.383711467890778149E-16 ) ) ;
#8673=ORIENTED_EDGE ( 'NONE', *, *, #5985, .T. ) ;
#8674=DIRECTION ( 'NONE',  ( 8.018662683283438208E-16, -5.975035461963189015E-16, -1.000000000000000000 ) ) ;
#8675=EDGE_CURVE ( 'NONE', #6428, #8353, #7407, .T. ) ;
#8677=CARTESIAN_POINT ( 'NONE',  ( -22.70913108387521007, -17.14542124616560770, 57.00231026484397745 ) ) ;
#8678=LINE ( 'NONE', #652, #3668 ) ;
#8679=CARTESIAN_POINT ( 'NONE',  ( -8.703838785437527648, -17.86878899887247130, 57.00231026484399166 ) ) ;
#8681=CARTESIAN_POINT ( 'NONE',  ( -22.94870171817393256, -18.69135635822624053, 56.85231026484398598 ) ) ;
#8682=CARTESIAN_POINT ( 'NONE',  ( -12.84854673063649777, -12.36513540471286277, 56.89875687425070794 ) ) ;
#8684=CARTESIAN_POINT ( 'NONE',  ( -8.561607448813433052, -9.375294326971793879, 56.85231026484400019 ) ) ;
#8685=LINE ( 'NONE', #2879, #4488 ) ;
#8686=ORIENTED_EDGE ( 'NONE', *, *, #4404, .F. ) ;
#8687=AXIS2_PLACEMENT_3D ( 'NONE', #359, #13577, #4164 ) ;
#8690=VERTEX_POINT ( 'NONE', #4976 ) ;
#8691=EDGE_CURVE ( 'NONE', #7312, #4275, #4903, .T. ) ;
#8692=AXIS2_PLACEMENT_3D ( 'NONE', #4726, #9388, #15121 ) ;
#8694=EDGE_LOOP ( 'NONE', ( #12694, #4389, #3318, #13687 ) ) ;
#8695=CARTESIAN_POINT ( 'NONE',  ( -8.971570239337626873, -21.04953708182106098, 56.85231026484400019 ) ) ;
#8701=DIRECTION ( 'NONE',  ( 0.5975035461963189576, 0.8018662683283437342, 0.000000000000000000 ) ) ;
#8703=ORIENTED_EDGE ( 'NONE', *, *, #8998, .T. ) ;
#8704=DIRECTION ( 'NONE',  ( -8.018662683283438208E-16, 5.975035461963189015E-16, 1.000000000000000000 ) ) ;
#8705=DIRECTION ( 'NONE',  ( -8.018662683283438208E-16, 5.975035461963189015E-16, 1.000000000000000000 ) ) ;
#8706=VERTEX_POINT ( 'NONE', #2752 ) ;
#8707=VERTEX_POINT ( 'NONE', #12088 ) ;
#8710=ORIENTED_EDGE ( 'NONE', *, *, #1207, .T. ) ;
#8712=CONICAL_SURFACE ( 'NONE', #4562, 4.499999999999999112, 0.7853981633974476129 ) ;
#8713=CARTESIAN_POINT ( 'NONE',  ( -25.29546517631143132, -15.38982603914036140, 56.85231026484398598 ) ) ;
#8719=DIRECTION ( 'NONE',  ( 0.5975035461963189576, 0.8018662683283437342, 0.000000000000000000 ) ) ;
#8721=VECTOR ( 'NONE', #7844, 1000.000000000000114 ) ;
#8723=CARTESIAN_POINT ( 'NONE',  ( -21.17290370923395670, -9.280041403099277275, 56.85231026484398598 ) ) ;
#8725=VERTEX_POINT ( 'NONE', #9927 ) ;
#8727=CARTESIAN_POINT ( 'NONE',  ( -15.49969986081092088, -13.50737899243822504, 56.85231026484398598 ) ) ;
#8729=EDGE_LOOP ( 'NONE', ( #11742, #4835, #6572, #13392 ) ) ;
#8731=VERTEX_POINT ( 'NONE', #14755 ) ;
#8734=CARTESIAN_POINT ( 'NONE',  ( -7.145558396657055944, -18.95797028117975458, 54.00231026484400587 ) ) ;
#8735=VECTOR ( 'NONE', #6227, 1000.000000000000227 ) ;
#8736=DIRECTION ( 'NONE',  ( 0.5975035461963172922, 0.8018662683283449555, 0.000000000000000000 ) ) ;
#8737=EDGE_CURVE ( 'NONE', #7024, #13353, #5491, .T. ) ;
#8738=PLANE ( 'NONE',  #2507 ) ;
#8740=ORIENTED_EDGE ( 'NONE', *, *, #13016, .F. ) ;
#8742=DIRECTION ( 'NONE',  ( 0.5975035461963187355, 0.8018662683283439563, 0.000000000000000000 ) ) ;
#8743=ORIENTED_EDGE ( 'NONE', *, *, #193, .F. ) ;
#8744=ORIENTED_EDGE ( 'NONE', *, *, #6824, .T. ) ;
#8746=CIRCLE ( 'NONE', #2165, 9.974999999999999645 ) ;
#8747=CARTESIAN_POINT ( 'NONE',  ( -5.615565924346646476, -12.16405426399944112, 56.85231026484400019 ) ) ;
#8753=AXIS2_PLACEMENT_3D ( 'NONE', #7311, #1962, #12367 ) ;
#8754=LINE ( 'NONE', #12593, #7265 ) ;
#8757=EDGE_CURVE ( 'NONE', #3679, #6892, #2968, .T. ) ;
#8758=DIRECTION ( 'NONE',  ( -8.018662683283439195E-16, 5.975035461963190001E-16, 1.000000000000000000 ) ) ;
#8760=CARTESIAN_POINT ( 'NONE',  ( -7.307539508764906877, -16.04208977798462854, 56.85231026484400019 ) ) ;
#8761=VECTOR ( 'NONE', #11182, 1000.000000000000114 ) ;
#8762=DIRECTION ( 'NONE',  ( 0.8018662683283436232, -0.5975035461963189576, 9.999999999999996833E-16 ) ) ;
#8766=DIRECTION ( 'NONE',  ( 0.2196982563774082797, 0.9755678736739573642, -4.067366430757958773E-16 ) ) ;
#8768=LINE ( 'NONE', #14442, #5666 ) ;
#8773=VECTOR ( 'NONE', #3019, 1000.000000000000227 ) ;
#8774=DIRECTION ( 'NONE',  ( 0.5975035461963189576, 0.8018662683283437342, 0.000000000000000000 ) ) ;
#8780=EDGE_CURVE ( 'NONE', #5861, #13533, #11661, .T. ) ;
#8784=ORIENTED_EDGE ( 'NONE', *, *, #11773, .T. ) ;
#8785=ORIENTED_EDGE ( 'NONE', *, *, #12420, .T. ) ;
#8786=AXIS2_PLACEMENT_3D ( 'NONE', #12666, #5688, #11655 ) ;
#8792=CARTESIAN_POINT ( 'NONE',  ( -15.49969986081092088, -13.50737899243822504, 56.85231026484398598 ) ) ;
#8794=CARTESIAN_POINT ( 'NONE',  ( -9.425865349984700714, -18.82901260770113794, 56.85231026484400019 ) ) ;
#8797=DIRECTION ( 'NONE',  ( -0.8772189822852959340, 0.4800904676395371662, -9.902680687415702019E-16 ) ) ;
#8799=DIRECTION ( 'NONE',  ( 0.8018662683283436232, -0.5975035461963189576, 9.999999999999996833E-16 ) ) ;
#8800=VECTOR ( 'NONE', #4993, 1000.000000000000000 ) ;
#8802=CARTESIAN_POINT ( 'NONE',  ( -15.53608329785963527, -13.54167542823733328, 56.85231026484398598 ) ) ;
#8803=CARTESIAN_POINT ( 'NONE',  ( -20.65541546412893226, -22.04665423204158969, 56.85231026484398598 ) ) ;
#8804=ORIENTED_EDGE ( 'NONE', *, *, #1496, .T. ) ;
#8808=VERTEX_POINT ( 'NONE', #5343 ) ;
#8810=EDGE_CURVE ( 'NONE', #10889, #10559, #2825, .T. ) ;
#8811=DIRECTION ( 'NONE',  ( 0.5975035461963188466, 0.8018662683283437342, 0.000000000000000000 ) ) ;
#8812=CARTESIAN_POINT ( 'NONE',  ( -20.69940085690220144, -18.30574950243923027, 56.85231026484398598 ) ) ;
#8813=DIRECTION ( 'NONE',  ( -8.018662683283438208E-16, 5.975035461963189015E-16, 1.000000000000000000 ) ) ;
#8814=FACE_OUTER_BOUND ( 'NONE', #7963, .T. ) ;
#8817=CARTESIAN_POINT ( 'NONE',  ( -21.18752042047970363, -7.775019331617081697, 57.00231026484397745 ) ) ;
#8818=ORIENTED_EDGE ( 'NONE', *, *, #14745, .T. ) ;
#8821=VERTEX_POINT ( 'NONE', #5193 ) ;
#8822=CARTESIAN_POINT ( 'NONE',  ( -24.08903783298838519, -16.43731469134198520, 56.85231026484398598 ) ) ;
#8825=CARTESIAN_POINT ( 'NONE',  ( -15.53608329785963527, -13.54167542823733328, 56.85231026484398598 ) ) ;
#8829=DIRECTION ( 'NONE',  ( 0.1165201156931293391, 0.9931883319083343320, -4.999999999999998416E-16 ) ) ;
#8833=VERTEX_POINT ( 'NONE', #7555 ) ;
#8837=CIRCLE ( 'NONE', #10060, 9.974999999999997868 ) ;
#8838=DIRECTION ( 'NONE',  ( -0.9354976265738682573, 0.3533329742249642913, -9.612616959383187437E-16 ) ) ;
#8839=VERTEX_POINT ( 'NONE', #4196 ) ;
#8840=PLANE ( 'NONE',  #1248 ) ;
#8845=DIRECTION ( 'NONE',  ( -8.018662683283439195E-16, 5.975035461963190001E-16, 1.000000000000000000 ) ) ;
#8849=VECTOR ( 'NONE', #10509, 999.9999999999998863 ) ;
#8852=CARTESIAN_POINT ( 'NONE',  ( -18.54556661251663030, -20.98627902725976213, 56.85231026484398598 ) ) ;
#8859=ORIENTED_EDGE ( 'NONE', *, *, #6154, .F. ) ;
#8860=EDGE_LOOP ( 'NONE', ( #5597, #5265, #7851, #11276 ) ) ;
#8861=DIRECTION ( 'NONE',  ( 0.7805252200231685977, -0.6251242923673534513, 9.993908270190957033E-16 ) ) ;
#8863=ADVANCED_FACE ( 'NONE', ( #10307 ), #13908, .F. ) ;
#8864=FACE_OUTER_BOUND ( 'NONE', #322, .T. ) ;
#8865=CIRCLE ( 'NONE', #4729, 5.000000000000000000 ) ;
#8868=EDGE_CURVE ( 'NONE', #9881, #6584, #14399, .T. ) ;
#8871=CYLINDRICAL_SURFACE ( 'NONE', #14128, 9.974999999999999645 ) ;
#8872=EDGE_CURVE ( 'NONE', #2134, #6821, #4427, .T. ) ;
#8873=AXIS2_PLACEMENT_3D ( 'NONE', #8392, #7233, #11919 ) ;
#8874=DIRECTION ( 'NONE',  ( 0.5975035461963188466, 0.8018662683283437342, 0.000000000000000000 ) ) ;
#8877=DIRECTION ( 'NONE',  ( 0.2640193276336892936, -0.9645173894937585368, 7.880107536067212861E-16 ) ) ;
#8878=CARTESIAN_POINT ( 'NONE',  ( -11.58094331127308507, -5.879823872646938732, 57.00231026484397745 ) ) ;
#8883=ORIENTED_EDGE ( 'NONE', *, *, #10588, .T. ) ;
#8887=EDGE_CURVE ( 'NONE', #8293, #7892, #3878, .T. ) ;
#8892=DIRECTION ( 'NONE',  ( -0.2975196656470009415, 0.9547156899063180546, -8.090169943749472730E-16 ) ) ;
#8893=AXIS2_PLACEMENT_3D ( 'NONE', #195, #9516, #5085 ) ;
#8894=CARTESIAN_POINT ( 'NONE',  ( -7.016473591028808521, -8.259951331604913349, 56.85231026484400019 ) ) ;
#8896=CARTESIAN_POINT ( 'NONE',  ( -16.48891182509095543, -11.21141303238454334, 51.00231026484399166 ) ) ;
#8897=ORIENTED_EDGE ( 'NONE', *, *, #2672, .F. ) ;
#8898=CARTESIAN_POINT ( 'NONE',  ( -15.49969986081086226, -13.50737899243826767, -13.99768973515600301 ) ) ;
#8900=ORIENTED_EDGE ( 'NONE', *, *, #11496, .F. ) ;
#8901=VECTOR ( 'NONE', #15122, 1000.000000000000000 ) ;
#8903=ORIENTED_EDGE ( 'NONE', *, *, #15077, .T. ) ;
#8906=LINE ( 'NONE', #13440, #4896 ) ;
#8907=DIRECTION ( 'NONE',  ( -8.018662683283438208E-16, 5.975035461963189015E-16, 1.000000000000000000 ) ) ;
#8908=PLANE ( 'NONE',  #11574 ) ;
#8909=FACE_OUTER_BOUND ( 'NONE', #10576, .T. ) ;
#8914=EDGE_CURVE ( 'NONE', #13944, #11184, #375, .T. ) ;
#8915=ORIENTED_EDGE ( 'NONE', *, *, #2193, .T. ) ;
#8917=EDGE_CURVE ( 'NONE', #13555, #14491, #3657, .T. ) ;
#8919=CARTESIAN_POINT ( 'NONE',  ( -18.15085299098533866, -14.64962258016358554, 51.10586365543726117 ) ) ;
#8920=DIRECTION ( 'NONE',  ( -8.018662683283439195E-16, 5.975035461963190001E-16, 1.000000000000000000 ) ) ;
#8925=DIRECTION ( 'NONE',  ( -8.018662683283438208E-16, 5.975035461963189015E-16, 1.000000000000000000 ) ) ;
#8926=DIRECTION ( 'NONE',  ( -0.5975035461963187355, -0.8018662683283439563, 0.000000000000000000 ) ) ;
#8927=CARTESIAN_POINT ( 'NONE',  ( -12.32172653804166096, -7.186294389320899256, 56.85231026484398598 ) ) ;
#8928=VERTEX_POINT ( 'NONE', #3802 ) ;
#8931=LINE ( 'NONE', #1980, #13877 ) ;
#8933=ORIENTED_EDGE ( 'NONE', *, *, #6782, .F. ) ;
#8942=DIRECTION ( 'NONE',  ( -8.018662683283438208E-16, 5.975035461963189015E-16, 1.000000000000000000 ) ) ;
#8949=VERTEX_POINT ( 'NONE', #11835 ) ;
#8950=ORIENTED_EDGE ( 'NONE', *, *, #2351, .T. ) ;
#8955=AXIS2_PLACEMENT_3D ( 'NONE', #1168, #13872, #8121 ) ;
#8957=DIRECTION ( 'NONE',  ( 8.018662683283438208E-16, -5.975035461963189015E-16, -1.000000000000000000 ) ) ;
#8958=FACE_OUTER_BOUND ( 'NONE', #6317, .T. ) ;
#8961=DIRECTION ( 'NONE',  ( 0.5975035461963188466, 0.8018662683283437342, 0.000000000000000000 ) ) ;
#8962=FACE_OUTER_BOUND ( 'NONE', #7467, .T. ) ;
#8963=EDGE_CURVE ( 'NONE', #14661, #13499, #7155, .T. ) ;
#8964=ORIENTED_EDGE ( 'NONE', *, *, #4779, .T. ) ;
#8967=VERTEX_POINT ( 'NONE', #8385 ) ;
#8968=ORIENTED_EDGE ( 'NONE', *, *, #6901, .F. ) ;
#8969=ORIENTED_EDGE ( 'NONE', *, *, #8338, .T. ) ;
#8971=ORIENTED_EDGE ( 'NONE', *, *, #14933, .F. ) ;
#8972=AXIS2_PLACEMENT_3D ( 'NONE', #10462, #6995, #14977 ) ;
#8975=CARTESIAN_POINT ( 'NONE',  ( -15.49969986081091378, -13.50737899243822859, 51.00231026484399166 ) ) ;
#8980=LINE ( 'NONE', #14657, #13771 ) ;
#8981=DIRECTION ( 'NONE',  ( -8.018662683283438208E-16, 5.975035461963189015E-16, 1.000000000000000000 ) ) ;
#8982=VECTOR ( 'NONE', #12361, 1000.000000000000000 ) ;
#8985=ADVANCED_FACE ( 'NONE', ( #11913 ), #1436, .F. ) ;
#8986=DIRECTION ( 'NONE',  ( -0.8599296884906622029, 0.5104125104779001498, -9.945218953682734920E-16 ) ) ;
#8987=VERTEX_POINT ( 'NONE', #14058 ) ;
#8995=( GEOMETRIC_REPRESENTATION_CONTEXT ( 3 ) GLOBAL_UNCERTAINTY_ASSIGNED_CONTEXT ( ( #9252 ) ) GLOBAL_UNIT_ASSIGNED_CONTEXT ( ( #11714, #5890, #6040 ) ) REPRESENTATION_CONTEXT ( 'NONE', 'WORKASPACE' ) );
#8998=EDGE_CURVE ( 'NONE', #9327, #14941, #6161, .T. ) ;
#8999=CARTESIAN_POINT ( 'NONE',  ( -13.95777467540137806, -22.45074059323463089, 57.00231026484399166 ) ) ;
#9000=AXIS2_PLACEMENT_3D ( 'NONE', #12168, #1683, #14317 ) ;
#9006=DIRECTION ( 'NONE',  ( -0.7109061395677416240, 0.7032868978765995926, -9.902680687415702019E-16 ) ) ;
#9008=ORIENTED_EDGE ( 'NONE', *, *, #13659, .F. ) ;
#9010=VERTEX_POINT ( 'NONE', #5032 ) ;
#9011=ORIENTED_EDGE ( 'NONE', *, *, #13728, .F. ) ;
#9014=VECTOR ( 'NONE', #3920, 999.9999999999998863 ) ;
#9015=CARTESIAN_POINT ( 'NONE',  ( -13.81224214977857123, -23.33861042463823665, 57.00231026484399166 ) ) ;
#9016=DIRECTION ( 'NONE',  ( -8.018662683283438208E-16, 5.975035461963189015E-16, 1.000000000000000000 ) ) ;
#9017=EDGE_CURVE ( 'NONE', #13485, #10787, #7745, .T. ) ;
#9021=VECTOR ( 'NONE', #9994, 1000.000000000000000 ) ;
#9023=ORIENTED_EDGE ( 'NONE', *, *, #9159, .F. ) ;
#9025=CARTESIAN_POINT ( 'NONE',  ( -15.49969986081092088, -13.50737899243822504, 57.00231026484397745 ) ) ;
#9031=DIRECTION ( 'NONE',  ( -8.018662683283438208E-16, 5.975035461963189015E-16, 1.000000000000000000 ) ) ;
#9037=AXIS2_PLACEMENT_3D ( 'NONE', #5446, #11264, #12491 ) ;
#9040=PLANE ( 'NONE',  #13749 ) ;
#9046=ORIENTED_EDGE ( 'NONE', *, *, #13100, .T. ) ;
#9052=EDGE_CURVE ( 'NONE', #7657, #221, #6533, .T. ) ;
#9055=CIRCLE ( 'NONE', #6858, 9.974999999999999645 ) ;
#9057=DIRECTION ( 'NONE',  ( -8.018662683283438208E-16, 5.975035461963189015E-16, 1.000000000000000000 ) ) ;
#9061=LINE ( 'NONE', #7825, #3369 ) ;
#9063=ORIENTED_EDGE ( 'NONE', *, *, #11602, .T. ) ;
#9064=EDGE_CURVE ( 'NONE', #13179, #12486, #14513, .T. ) ;
#9065=ORIENTED_EDGE ( 'NONE', *, *, #7217, .F. ) ;
#9069=VERTEX_POINT ( 'NONE', #8684 ) ;
#9072=CARTESIAN_POINT ( 'NONE',  ( -12.04767799572592502, -20.80732214584531548, 56.85231026484400019 ) ) ;
#9076=CARTESIAN_POINT ( 'NONE',  ( -15.19690733689918538, -23.47778227853769195, 57.00231026484399166 ) ) ;
#9078=EDGE_LOOP ( 'NONE', ( #11352, #4443, #5002, #1344 ) ) ;
#9080=LINE ( 'NONE', #5267, #5553 ) ;
#9083=VECTOR ( 'NONE', #11319, 1000.000000000000114 ) ;
#9086=VERTEX_POINT ( 'NONE', #512 ) ;
#9090=VECTOR ( 'NONE', #3641, 1000.000000000000000 ) ;
#9091=CARTESIAN_POINT ( 'NONE',  ( -5.596483669297570351, -12.31283553816471432, 57.00231026484399166 ) ) ;
#9093=VECTOR ( 'NONE', #15060, 1000.000000000000114 ) ;
#9095=LINE ( 'NONE', #14839, #1875 ) ;
#9096=CARTESIAN_POINT ( 'NONE',  ( -18.50396719079564889, -6.011671700261853601, 57.00231026484397745 ) ) ;
#9097=PLANE ( 'NONE',  #5001 ) ;
#9099=VERTEX_POINT ( 'NONE', #443 ) ;
#9101=ORIENTED_EDGE ( 'NONE', *, *, #10473, .T. ) ;
#9104=VERTEX_POINT ( 'NONE', #9768 ) ;
#9105=ADVANCED_FACE ( 'NONE', ( #2953 ), #2808, .T. ) ;
#9106=ORIENTED_EDGE ( 'NONE', *, *, #5228, .F. ) ;
#9108=VECTOR ( 'NONE', #11856, 1000.000000000000114 ) ;
#9111=DIRECTION ( 'NONE',  ( -8.018662683283439195E-16, 5.975035461963190001E-16, 1.000000000000000000 ) ) ;
#9114=VECTOR ( 'NONE', #7335, 1000.000000000000000 ) ;
#9115=AXIS2_PLACEMENT_3D ( 'NONE', #3478, #4710, #6972 ) ;
#9116=ORIENTED_EDGE ( 'NONE', *, *, #13819, .F. ) ;
#9118=VERTEX_POINT ( 'NONE', #9843 ) ;
#9119=CARTESIAN_POINT ( 'NONE',  ( -15.49969986081092088, -13.50737899243822504, 56.85231026484398598 ) ) ;
#9120=ORIENTED_EDGE ( 'NONE', *, *, #6078, .F. ) ;
#9121=ORIENTED_EDGE ( 'NONE', *, *, #1994, .F. ) ;
#9123=EDGE_CURVE ( 'NONE', #6010, #5192, #8615, .T. ) ;
#9124=CARTESIAN_POINT ( 'NONE',  ( -8.722797460041883610, -15.53942693735753444, 57.00231026484399166 ) ) ;
#9125=EDGE_LOOP ( 'NONE', ( #1943, #13224, #3104, #6164 ) ) ;
#9127=PLANE ( 'NONE',  #4159 ) ;
#9129=AXIS2_PLACEMENT_3D ( 'NONE', #9232, #12774, #12618 ) ;
#9130=AXIS2_PLACEMENT_3D ( 'NONE', #11520, #3107, #6539 ) ;
#9131=DIRECTION ( 'NONE',  ( 8.018662683283438208E-16, -5.975035461963189015E-16, -1.000000000000000000 ) ) ;
#9135=FACE_OUTER_BOUND ( 'NONE', #10884, .T. ) ;
#9137=VERTEX_POINT ( 'NONE', #6310 ) ;
#9138=ORIENTED_EDGE ( 'NONE', *, *, #12487, .T. ) ;
#9141=DIRECTION ( 'NONE',  ( 0.9931883319083343320, -0.1165201156931293391, 8.660254037844387408E-16 ) ) ;
#9143=EDGE_LOOP ( 'NONE', ( #12778, #2922, #5475, #12312 ) ) ;
#9144=DIRECTION ( 'NONE',  ( -8.018662683283438208E-16, 5.975035461963189015E-16, 1.000000000000000000 ) ) ;
#9145=EDGE_CURVE ( 'NONE', #12780, #2678, #2878, .T. ) ;
#9150=CARTESIAN_POINT ( 'NONE',  ( -18.72761429428784297, -5.025526694139714756, 57.00231026484397745 ) ) ;
#9151=CARTESIAN_POINT ( 'NONE',  ( -13.72291223624743317, -3.691898834178107602, 56.85231026484398598 ) ) ;
#9152=DIRECTION ( 'NONE',  ( 0.5975035461963188466, 0.8018662683283437342, 0.000000000000000000 ) ) ;
#9153=VERTEX_POINT ( 'NONE', #9982 ) ;
#9159=EDGE_CURVE ( 'NONE', #5814, #2590, #3025, .T. ) ;
#9161=DIRECTION ( 'NONE',  ( -0.7805252200231699300, 0.6251242923673516749, -9.993908270190957033E-16 ) ) ;
#9162=ORIENTED_EDGE ( 'NONE', *, *, #12717, .F. ) ;
#9163=LINE ( 'NONE', #4362, #541 ) ;
#9164=CARTESIAN_POINT ( 'NONE',  ( -22.64353467404651354, -6.545608444567306172, 56.85231026484398598 ) ) ;
#9166=DIRECTION ( 'NONE',  ( 8.018662683283438208E-16, -5.975035461963189015E-16, -1.000000000000000000 ) ) ;
#9169=DIRECTION ( 'NONE',  ( -8.018662683283438208E-16, 5.975035461963189015E-16, 1.000000000000000000 ) ) ;
#9170=DIRECTION ( 'NONE',  ( -8.018662683283438208E-16, 5.975035461963189015E-16, 1.000000000000000000 ) ) ;
#9171=CARTESIAN_POINT ( 'NONE',  ( -21.18752042047970363, -7.775019331617081697, 56.85231026484398598 ) ) ;
#9174=EDGE_CURVE ( 'NONE', #8039, #7394, #9061, .T. ) ;
#9180=ORIENTED_EDGE ( 'NONE', *, *, #10030, .T. ) ;
#9181=AXIS2_PLACEMENT_3D ( 'NONE', #8479, #12232, #12306 ) ;
#9185=EDGE_CURVE ( 'NONE', #14032, #11333, #6907, .T. ) ;
#9188=ORIENTED_EDGE ( 'NONE', *, *, #5188, .F. ) ;
#9189=DIRECTION ( 'NONE',  ( 0.9755678736739583634, -0.2196982563774038943, 9.135454576426008610E-16 ) ) ;
#9190=ORIENTED_EDGE ( 'NONE', *, *, #13751, .F. ) ;
#9191=FACE_OUTER_BOUND ( 'NONE', #5364, .T. ) ;
#9196=ORIENTED_EDGE ( 'NONE', *, *, #2626, .F. ) ;
#9198=VECTOR ( 'NONE', #5728, 1000.000000000000000 ) ;
#9200=DIRECTION ( 'NONE',  ( 0.8357240892757724637, 0.5491495666976170531, 3.420201433256690644E-16 ) ) ;
#9210=VERTEX_POINT ( 'NONE', #4481 ) ;
#9213=CIRCLE ( 'NONE', #5082, 9.974999999999999645 ) ;
#9214=CARTESIAN_POINT ( 'NONE',  ( -16.57334897777262483, -22.01522992987520766, 56.85231026484400019 ) ) ;
#9217=DIRECTION ( 'NONE',  ( 0.5975035461963189576, 0.8018662683283437342, 0.000000000000000000 ) ) ;
#9220=VECTOR ( 'NONE', #7293, 1000.000000000000000 ) ;
#9223=DIRECTION ( 'NONE',  ( -8.018662683283438208E-16, 5.975035461963189015E-16, 1.000000000000000000 ) ) ;
#9224=VECTOR ( 'NONE', #8084, 1000.000000000000000 ) ;
#9225=CIRCLE ( 'NONE', #13880, 9.974999999999999645 ) ;
#9226=CARTESIAN_POINT ( 'NONE',  ( -15.49969986081092088, -13.50737899243822504, 56.85231026484398598 ) ) ;
#9228=ADVANCED_FACE ( 'NONE', ( #1961 ), #8137, .T. ) ;
#9232=CARTESIAN_POINT ( 'NONE',  ( -15.47724068538499154, -13.46270701644446177, 56.85231026484398598 ) ) ;
#9233=LINE ( 'NONE', #11685, #8761 ) ;
#9234=VERTEX_POINT ( 'NONE', #11288 ) ;
#9235=FACE_OUTER_BOUND ( 'NONE', #5560, .T. ) ;
#9236=EDGE_LOOP ( 'NONE', ( #66, #13435, #8029, #7807 ) ) ;
#9241=CARTESIAN_POINT ( 'NONE',  ( -16.24681173062539230, -5.467015265965240012, 56.85231026484398598 ) ) ;
#9244=DIRECTION ( 'NONE',  ( 0.5975035461963188466, 0.8018662683283437342, 0.000000000000000000 ) ) ;
#9245=EDGE_CURVE ( 'NONE', #13936, #1243, #3481, .T. ) ;
#9249=LINE ( 'NONE', #853, #4960 ) ;
#9251=DIRECTION ( 'NONE',  ( 0.5975035461963189576, 0.8018662683283437342, 0.000000000000000000 ) ) ;
#9252=UNCERTAINTY_MEASURE_WITH_UNIT (LENGTH_MEASURE( 1.000000000000000082E-05 ), #11714, 'distance_accuracy_value', 'NONE');
#9256=EDGE_LOOP ( 'NONE', ( #3659, #7064, #5680, #4910 ) ) ;
#9258=ORIENTED_EDGE ( 'NONE', *, *, #7282, .F. ) ;
#9259=PRODUCT_DEFINITION_FORMATION_WITH_SPECIFIED_SOURCE ( 'ANY', '', #7330, .NOT_KNOWN. ) ;
#9261=ORIENTED_EDGE ( 'NONE', *, *, #14593, .F. ) ;
#9264=CARTESIAN_POINT ( 'NONE',  ( -23.59621936791819863, -19.33378413377806027, 54.00231026484399166 ) ) ;
#9266=EDGE_CURVE ( 'NONE', #2114, #1582, #5695, .T. ) ;
#9267=ADVANCED_FACE ( 'NONE', ( #9135 ), #965, .F. ) ;
#9268=AXIS2_PLACEMENT_3D ( 'NONE', #12042, #14705, #12187 ) ;
#9271=ORIENTED_EDGE ( 'NONE', *, *, #5030, .F. ) ;
#9274=FACE_OUTER_BOUND ( 'NONE', #10172, .T. ) ;
#9275=VERTEX_POINT ( 'NONE', #6682 ) ;
#9277=LINE ( 'NONE', #5830, #11038 ) ;
#9280=LINE ( 'NONE', #13951, #3488 ) ;
#9282=DIRECTION ( 'NONE',  ( 0.5975035461963188466, 0.8018662683283437342, 0.000000000000000000 ) ) ;
#9283=DIRECTION ( 'NONE',  ( 0.5975035461963189576, 0.8018662683283437342, 0.000000000000000000 ) ) ;
#9291=ORIENTED_EDGE ( 'NONE', *, *, #9185, .T. ) ;
#9292=ORIENTED_EDGE ( 'NONE', *, *, #4961, .T. ) ;
#9298=ORIENTED_EDGE ( 'NONE', *, *, #10357, .T. ) ;
#9299=CARTESIAN_POINT ( 'NONE',  ( -8.791486474964740339, -6.124933722071906672, 54.00231026484399166 ) ) ;
#9304=DIRECTION ( 'NONE',  ( -0.9999272109403024578, 0.01206535623791937448, -8.090169943749475688E-16 ) ) ;
#9305=EDGE_LOOP ( 'NONE', ( #6906, #834, #6557, #6188 ) ) ;
#9307=DIRECTION ( 'NONE',  ( -0.8222303661035965661, 0.5691548339926012501, -9.993908270190953088E-16 ) ) ;
#9308=DIRECTION ( 'NONE',  ( -8.018662683283439195E-16, 5.975035461963190001E-16, 1.000000000000000000 ) ) ;
#9312=PLANE ( 'NONE',  #5427 ) ;
#9313=AXIS2_PLACEMENT_3D ( 'NONE', #3933, #14415, #8444 ) ;
#9314=EDGE_CURVE ( 'NONE', #2588, #4531, #4867, .T. ) ;
#9316=DIRECTION ( 'NONE',  ( 0.9225966037272106401, -0.3857661296576155863, 9.702957262759965065E-16 ) ) ;
#9320=DIRECTION ( 'NONE',  ( 0.2872152572324145892, 0.9578660637129379207, -3.420201433256678811E-16 ) ) ;
#9322=AXIS2_PLACEMENT_3D ( 'NONE', #8560, #3029, #3822 ) ;
#9326=DIRECTION ( 'NONE',  ( -0.9868311969055005850, -0.1617534816134010012, -6.946583704589984503E-16 ) ) ;
#9327=VERTEX_POINT ( 'NONE', #12901 ) ;
#9328=DIRECTION ( 'NONE',  ( 0.5975035461963189576, 0.8018662683283437342, 0.000000000000000000 ) ) ;
#9331=ORIENTED_EDGE ( 'NONE', *, *, #1377, .F. ) ;
#9333=EDGE_CURVE ( 'NONE', #8707, #13092, #14346, .T. ) ;
#9334=CIRCLE ( 'NONE', #8605, 9.974999999999999645 ) ;
#9335=LINE ( 'NONE', #6035, #12908 ) ;
#9336=ADVANCED_FACE ( 'NONE', ( #5840 ), #3711, .F. ) ;
#9346=EDGE_CURVE ( 'NONE', #17, #3306, #13133, .T. ) ;
#9347=CARTESIAN_POINT ( 'NONE',  ( -9.002116193859002635, -10.70790913352571927, 57.00231026484399166 ) ) ;
#9348=DIRECTION ( 'NONE',  ( 0.9885168150181788960, -0.1511109077013150503, 8.829475928589270966E-16 ) ) ;
#9349=VECTOR ( 'NONE', #2168, 1000.000000000000000 ) ;
#9350=DIRECTION ( 'NONE',  ( -0.5975035461963188466, -0.8018662683283437342, 0.000000000000000000 ) ) ;
#9351=ORIENTED_EDGE ( 'NONE', *, *, #8439, .F. ) ;
#9353=ORIENTED_EDGE ( 'NONE', *, *, #7816, .F. ) ;
#9354=DIRECTION ( 'NONE',  ( -0.8719950447285834683, -0.4895147004624025855, -4.067366430758019910E-16 ) ) ;
#9356=ORIENTED_EDGE ( 'NONE', *, *, #6967, .T. ) ;
#9357=EDGE_CURVE ( 'NONE', #6428, #2864, #13330, .T. ) ;
#9358=DIRECTION ( 'NONE',  ( -0.5691548339926102429, -0.8222303661035904598, 3.489949670250058899E-17 ) ) ;
#9359=EDGE_CURVE ( 'NONE', #3205, #11477, #13056, .T. ) ;
#9361=DIRECTION ( 'NONE',  ( 0.01206535623791937274, 0.9999272109403024578, -5.877852522924727828E-16 ) ) ;
#9363=VECTOR ( 'NONE', #14420, 999.9999999999998863 ) ;
#9368=LINE ( 'NONE', #13886, #7420 ) ;
#9369=LINE ( 'NONE', #3328, #8631 ) ;
#9370=CARTESIAN_POINT ( 'NONE',  ( -13.81224214977857123, -23.33861042463823665, 54.00231026484399166 ) ) ;
#9372=CARTESIAN_POINT ( 'NONE',  ( -19.55678615628314532, -20.48959216528617233, 56.85231026484398598 ) ) ;
#9375=EDGE_LOOP ( 'NONE', ( #3757, #4229, #3942, #7337 ) ) ;
#9376=PLANE ( 'NONE',  #10564 ) ;
#9380=CARTESIAN_POINT ( 'NONE',  ( -16.58746603607634995, -23.42289157363888208, 56.85231026484400019 ) ) ;
#9382=EDGE_CURVE ( 'NONE', #12036, #7447, #4346, .T. ) ;
#9386=EDGE_CURVE ( 'NONE', #12018, #551, #4938, .T. ) ;
#9387=EDGE_CURVE ( 'NONE', #9600, #14274, #7213, .T. ) ;
#9388=DIRECTION ( 'NONE',  ( 0.5491495666976171641, -0.8357240892757725748, 9.396926207859082113E-16 ) ) ;
#9389=CYLINDRICAL_SURFACE ( 'NONE', #14740, 0.2500000000000014433 ) ;
#9395=ORIENTED_EDGE ( 'NONE', *, *, #9245, .T. ) ;
#9396=CARTESIAN_POINT ( 'NONE',  ( -12.84854673063649422, -12.36513540471287342, 51.10586365543726117 ) ) ;
#9398=FACE_OUTER_BOUND ( 'NONE', #6977, .T. ) ;
#9401=CARTESIAN_POINT ( 'NONE',  ( -15.49969986081092088, -13.50737899243822504, 56.85231026484398598 ) ) ;
#9404=EDGE_CURVE ( 'NONE', #7427, #11933, #3611, .T. ) ;
#9407=DIRECTION ( 'NONE',  ( 0.5975035461963187355, 0.8018662683283439563, 0.000000000000000000 ) ) ;
#9408=CARTESIAN_POINT ( 'NONE',  ( -12.11547932532413263, -20.83938426843124603, 56.85231026484400019 ) ) ;
#9409=ORIENTED_EDGE ( 'NONE', *, *, #2149, .F. ) ;
#9410=PLANE ( 'NONE',  #13003 ) ;
#9411=ORIENTED_EDGE ( 'NONE', *, *, #14845, .T. ) ;
#9412=FACE_OUTER_BOUND ( 'NONE', #3024, .T. ) ;
#9413=ORIENTED_EDGE ( 'NONE', *, *, #13313, .F. ) ;
#9423=FACE_OUTER_BOUND ( 'NONE', #514, .T. ) ;
#9424=DIRECTION ( 'NONE',  ( -0.9731439732146150989, -0.2301973227387161258, -6.427876096865397836E-16 ) ) ;
#9425=ADVANCED_FACE ( 'NONE', ( #1258 ), #4788, .F. ) ;
#9426=ORIENTED_EDGE ( 'NONE', *, *, #1484, .F. ) ;
#9429=AXIS2_PLACEMENT_3D ( 'NONE', #10231, #10458, #7923 ) ;
#9430=ORIENTED_EDGE ( 'NONE', *, *, #3266, .F. ) ;
#9434=VERTEX_POINT ( 'NONE', #14113 ) ;
#9435=DIRECTION ( 'NONE',  ( -8.018662683283438208E-16, 5.975035461963189015E-16, 1.000000000000000000 ) ) ;
#9444=EDGE_LOOP ( 'NONE', ( #10676, #10866, #2118, #2487 ) ) ;
#9447=ORIENTED_EDGE ( 'NONE', *, *, #9386, .T. ) ;
#9448=EDGE_LOOP ( 'NONE', ( #10711, #7702, #13041, #2661 ) ) ;
#9450=VERTEX_POINT ( 'NONE', #14191 ) ;
#9453=AXIS2_PLACEMENT_3D ( 'NONE', #11535, #1057, #9307 ) ;
#9454=LINE ( 'NONE', #210, #11667 ) ;
#9460=ORIENTED_EDGE ( 'NONE', *, *, #10527, .T. ) ;
#9461=DIRECTION ( 'NONE',  ( -8.018662683283438208E-16, 5.975035461963189015E-16, 1.000000000000000000 ) ) ;
#9463=ORIENTED_EDGE ( 'NONE', *, *, #13561, .F. ) ;
#9465=ORIENTED_EDGE ( 'NONE', *, *, #3225, .F. ) ;
#9466=DIRECTION ( 'NONE',  ( 8.018662683283438208E-16, -5.975035461963189015E-16, -1.000000000000000000 ) ) ;
#9475=VECTOR ( 'NONE', #12919, 1000.000000000000000 ) ;
#9477=FACE_OUTER_BOUND ( 'NONE', #11780, .T. ) ;
#9482=AXIS2_PLACEMENT_3D ( 'NONE', #13849, #9170, #9407 ) ;
#9484=PLANE ( 'NONE',  #12551 ) ;
#9487=FACE_OUTER_BOUND ( 'NONE', #12640, .T. ) ;
#9490=VERTEX_POINT ( 'NONE', #10900 ) ;
#9491=ORIENTED_EDGE ( 'NONE', *, *, #2608, .F. ) ;
#9492=FACE_OUTER_BOUND ( 'NONE', #10115, .T. ) ;
#9494=AXIS2_PLACEMENT_3D ( 'NONE', #8441, #11810, #192 ) ;
#9496=LINE ( 'NONE', #4684, #7931 ) ;
#9497=VECTOR ( 'NONE', #8986, 1000.000000000000114 ) ;
#9498=LINE ( 'NONE', #14171, #10767 ) ;
#9502=ORIENTED_EDGE ( 'NONE', *, *, #9743, .F. ) ;
#9507=LINE ( 'NONE', #14181, #9577 ) ;
#9508=ORIENTED_EDGE ( 'NONE', *, *, #4839, .T. ) ;
#9509=PLANE ( 'NONE',  #4720 ) ;
#9511=VECTOR ( 'NONE', #9741, 1000.000000000000000 ) ;
#9516=DIRECTION ( 'NONE',  ( -8.018662683283438208E-16, 5.975035461963189015E-16, 1.000000000000000000 ) ) ;
#9522=ORIENTED_EDGE ( 'NONE', *, *, #12174, .T. ) ;
#9523=VECTOR ( 'NONE', #6674, 1000.000000000000227 ) ;
#9524=ORIENTED_EDGE ( 'NONE', *, *, #3185, .F. ) ;
#9527=ORIENTED_EDGE ( 'NONE', *, *, #7076, .T. ) ;
#9528=PLANE ( 'NONE',  #6197 ) ;
#9529=EDGE_CURVE ( 'NONE', #7124, #11066, #6295, .T. ) ;
#9530=VECTOR ( 'NONE', #6808, 1000.000000000000000 ) ;
#9531=EDGE_CURVE ( 'NONE', #6280, #13533, #7444, .T. ) ;
#9532=EDGE_CURVE ( 'NONE', #8833, #5844, #11124, .T. ) ;
#9533=DIRECTION ( 'NONE',  ( 8.018662683283438208E-16, -5.975035461963189015E-16, -1.000000000000000000 ) ) ;
#9534=EDGE_CURVE ( 'NONE', #9709, #560, #643, .T. ) ;
#9538=ORIENTED_EDGE ( 'NONE', *, *, #9704, .F. ) ;
#9541=VERTEX_POINT ( 'NONE', #12122 ) ;
#9544=VERTEX_POINT ( 'NONE', #5305 ) ;
#9546=ORIENTED_EDGE ( 'NONE', *, *, #11443, .T. ) ;
#9548=EDGE_CURVE ( 'NONE', #13197, #8821, #10939, .T. ) ;
#9550=PLANE ( 'NONE',  #10812 ) ;
#9551=CARTESIAN_POINT ( 'NONE',  ( -22.56723502526082470, -13.84084068328822070, 57.00231026484397745 ) ) ;
#9552=DIRECTION ( 'NONE',  ( 0.6334982226805337957, -0.7737441449604673949, 9.702957262759957177E-16 ) ) ;
#9554=ORIENTED_EDGE ( 'NONE', *, *, #14708, .F. ) ;
#9560=ORIENTED_EDGE ( 'NONE', *, *, #12998, .T. ) ;
#9562=ORIENTED_EDGE ( 'NONE', *, *, #12253, .F. ) ;
#9564=ORIENTED_EDGE ( 'NONE', *, *, #5100, .T. ) ;
#9566=CARTESIAN_POINT ( 'NONE',  ( -12.25471857405102405, -7.219983152459794162, 56.85231026484398598 ) ) ;
#9568=LINE ( 'NONE', #3606, #11704 ) ;
#9573=LINE ( 'NONE', #9347, #2408 ) ;
#9576=CARTESIAN_POINT ( 'NONE',  ( -17.54662770128649285, -5.179934221328323929, 56.85231026484398598 ) ) ;
#9577=VECTOR ( 'NONE', #4776, 1000.000000000000114 ) ;
#9578=LINE ( 'NONE', #3769, #4933 ) ;
#9581=EDGE_LOOP ( 'NONE', ( #14345, #3656, #4165, #10022 ) ) ;
#9582=EDGE_LOOP ( 'NONE', ( #14856, #14789, #1095, #1718 ) ) ;
#9583=AXIS2_PLACEMENT_3D ( 'NONE', #8626, #9625, #8548 ) ;
#9584=VECTOR ( 'NONE', #5866, 1000.000000000000114 ) ;
#9588=CARTESIAN_POINT ( 'NONE',  ( -10.95221305062249506, -4.629260458021023261, 54.00231026484399166 ) ) ;
#9590=DIRECTION ( 'NONE',  ( 8.018662683283438208E-16, -5.975035461963189015E-16, -1.000000000000000000 ) ) ;
#9591=AXIS2_PLACEMENT_3D ( 'NONE', #7163, #2670, #2442 ) ;
#9592=VECTOR ( 'NONE', #14400, 1000.000000000000000 ) ;
#9593=CARTESIAN_POINT ( 'NONE',  ( -23.54290256004220439, -7.607589560680598773, 57.00231026484397745 ) ) ;
#9600=VERTEX_POINT ( 'NONE', #12348 ) ;
#9607=VECTOR ( 'NONE', #14431, 1000.000000000000000 ) ;
#9608=PLANE ( 'NONE',  #7548 ) ;
#9610=VECTOR ( 'NONE', #10314, 1000.000000000000114 ) ;
#9611=PLANE ( 'NONE',  #10398 ) ;
#9613=DIRECTION ( 'NONE',  ( 0.5975035461963189576, 0.8018662683283437342, 0.000000000000000000 ) ) ;
#9615=DIRECTION ( 'NONE',  ( -8.018662683283438208E-16, 5.975035461963189015E-16, 1.000000000000000000 ) ) ;
#9616=FACE_OUTER_BOUND ( 'NONE', #12836, .T. ) ;
#9617=ORIENTED_EDGE ( 'NONE', *, *, #2541, .T. ) ;
#9619=CARTESIAN_POINT ( 'NONE',  ( -7.490307934913750465, -12.48011759562962020, 56.85231026484400019 ) ) ;
#9621=ORIENTED_EDGE ( 'NONE', *, *, #11677, .F. ) ;
#9623=VECTOR ( 'NONE', #6361, 1000.000000000000000 ) ;
#9624=VERTEX_POINT ( 'NONE', #10271 ) ;
#9625=DIRECTION ( 'NONE',  ( -8.018662683283438208E-16, 5.975035461963189015E-16, 1.000000000000000000 ) ) ;
#9627=EDGE_CURVE ( 'NONE', #8100, #9541, #7994, .T. ) ;
#9628=AXIS2_PLACEMENT_3D ( 'NONE', #27, #12153, #6249 ) ;
#9629=CARTESIAN_POINT ( 'NONE',  ( -18.30022887753442618, -14.85008914724566509, 57.00231026484397745 ) ) ;
#9631=AXIS2_PLACEMENT_3D ( 'NONE', #11460, #987, #11611 ) ;
#9632=CARTESIAN_POINT ( 'NONE',  ( -8.744347237509680681, -17.93190845158491342, 56.85231026484400019 ) ) ;
#9635=DIRECTION ( 'NONE',  ( -8.018662683283438208E-16, 5.975035461963189015E-16, 1.000000000000000000 ) ) ;
#9642=CARTESIAN_POINT ( 'NONE',  ( -22.08930316869620825, -18.17457871440291228, 56.85231026484398598 ) ) ;
#9643=VERTEX_POINT ( 'NONE', #6889 ) ;
#9647=CARTESIAN_POINT ( 'NONE',  ( -5.859109405273538407, -10.94619944609606677, 57.00231026484399166 ) ) ;
#9648=CARTESIAN_POINT ( 'NONE',  ( -15.47224238247604511, -13.54916519690201149, 56.85231026484398598 ) ) ;
#9654=ADVANCED_FACE ( 'NONE', ( #11421 ), #797, .F. ) ;
#9656=PLANE ( 'NONE',  #2970 ) ;
#9660=ORIENTED_EDGE ( 'NONE', *, *, #9052, .T. ) ;
#9661=LINE ( 'NONE', #5222, #5410 ) ;
#9664=DIRECTION ( 'NONE',  ( -8.018662683283438208E-16, 5.975035461963189015E-16, 1.000000000000000000 ) ) ;
#9666=DIRECTION ( 'NONE',  ( 0.5975035461963189576, 0.8018662683283437342, 0.000000000000000000 ) ) ;
#9669=CARTESIAN_POINT ( 'NONE',  ( -22.04595456446742929, -18.23578246029658345, 57.00231026484397745 ) ) ;
#9671=PLANE ( 'NONE',  #11345 ) ;
#9672=CARTESIAN_POINT ( 'NONE',  ( -13.18491133144367389, -15.23222315862922827, 51.25231026484399166 ) ) ;
#9674=ORIENTED_EDGE ( 'NONE', *, *, #8404, .F. ) ;
#9675=DIRECTION ( 'NONE',  ( -0.3956847857120158740, 0.9183863840214728791, 0.000000000000000000 ) ) ;
#9676=CARTESIAN_POINT ( 'NONE',  ( -19.87664613915258371, -5.557310358991672139, 56.85231026484398598 ) ) ;
#9677=VERTEX_POINT ( 'NONE', #1018 ) ;
#9681=ORIENTED_EDGE ( 'NONE', *, *, #15052, .T. ) ;
#9684=EDGE_CURVE ( 'NONE', #14495, #13725, #5677, .T. ) ;
#9687=FACE_OUTER_BOUND ( 'NONE', #12583, .T. ) ;
#9690=CARTESIAN_POINT ( 'NONE',  ( -21.05979293892203330, -6.334749421441233430, 56.85231026484398598 ) ) ;
#9704=EDGE_CURVE ( 'NONE', #13117, #2290, #9578, .T. ) ;
#9705=DIRECTION ( 'NONE',  ( -8.018662683283438208E-16, 5.975035461963189015E-16, 1.000000000000000000 ) ) ;
#9709=VERTEX_POINT ( 'NONE', #2618 ) ;
#9717=VERTEX_POINT ( 'NONE', #14254 ) ;
#9718=VERTEX_POINT ( 'NONE', #11721 ) ;
#9719=CIRCLE ( 'NONE', #3853, 9.974999999999999645 ) ;
#9721=DIRECTION ( 'NONE',  ( -8.018662683283438208E-16, 5.975035461963189015E-16, 1.000000000000000000 ) ) ;
#9722=ADVANCED_FACE ( 'NONE', ( #5897 ), #30, .T. ) ;
#9725=EDGE_CURVE ( 'NONE', #10291, #5981, #10730, .T. ) ;
#9726=DIRECTION ( 'NONE',  ( 0.9183863840214729901, 0.3956847857120157075, 4.999999999999999402E-16 ) ) ;
#9731=EDGE_CURVE ( 'NONE', #14388, #6962, #3917, .T. ) ;
#9734=CARTESIAN_POINT ( 'NONE',  ( -8.703838785437527648, -17.86878899887247130, 56.85231026484400019 ) ) ;
#9738=VERTEX_POINT ( 'NONE', #5214 ) ;
#9739=DIRECTION ( 'NONE',  ( -8.018662683283438208E-16, 5.975035461963189015E-16, 1.000000000000000000 ) ) ;
#9741=DIRECTION ( 'NONE',  ( -8.018662683283438208E-16, 5.975035461963189015E-16, 1.000000000000000000 ) ) ;
#9743=EDGE_CURVE ( 'NONE', #2536, #13533, #8575, .T. ) ;
#9744=FACE_OUTER_BOUND ( 'NONE', #12584, .T. ) ;
#9745=DIRECTION ( 'NONE',  ( 8.018662683283438208E-16, -5.975035461963189015E-16, -1.000000000000000000 ) ) ;
#9747=LINE ( 'NONE', #3706, #2798 ) ;
#9751=DIRECTION ( 'NONE',  ( 0.5975035461963189576, 0.8018662683283437342, 0.000000000000000000 ) ) ;
#9753=FACE_OUTER_BOUND ( 'NONE', #1534, .T. ) ;
#9755=ORIENTED_EDGE ( 'NONE', *, *, #8868, .F. ) ;
#9763=CARTESIAN_POINT ( 'NONE',  ( -15.49969986081092088, -13.50737899243822504, 56.85231026484398598 ) ) ;
#9764=AXIS2_PLACEMENT_3D ( 'NONE', #1895, #1665, #6321 ) ;
#9767=EDGE_LOOP ( 'NONE', ( #4787, #15094, #10039, #615 ) ) ;
#9768=CARTESIAN_POINT ( 'NONE',  ( -7.506093261461533217, -14.65346081099998088, 56.85231026484400019 ) ) ;
#9770=ORIENTED_EDGE ( 'NONE', *, *, #14236, .T. ) ;
#9771=ADVANCED_FACE ( 'NONE', ( #4998 ), #13481, .F. ) ;
#9775=ORIENTED_EDGE ( 'NONE', *, *, #11730, .F. ) ;
#9777=ORIENTED_EDGE ( 'NONE', *, *, #6627, .T. ) ;
#9784=DIRECTION ( 'NONE',  ( 0.5975035461963189576, 0.8018662683283437342, 0.000000000000000000 ) ) ;
#9785=ORIENTED_EDGE ( 'NONE', *, *, #5602, .F. ) ;
#9786=PLANE ( 'NONE',  #10430 ) ;
#9787=DIRECTION ( 'NONE',  ( -0.9645173894937585368, -0.2640193276336892936, -6.156614753256587028E-16 ) ) ;
#9788=ADVANCED_FACE ( 'NONE', ( #2841 ), #9656, .F. ) ;
#9789=EDGE_LOOP ( 'NONE', ( #13645, #1800, #6984, #2697 ) ) ;
#9790=CARTESIAN_POINT ( 'NONE',  ( -24.33650094517379614, -11.44044972528773130, 56.85231026484398598 ) ) ;
#9793=ORIENTED_EDGE ( 'NONE', *, *, #13170, .F. ) ;
#9794=VERTEX_POINT ( 'NONE', #12255 ) ;
#9796=ORIENTED_EDGE ( 'NONE', *, *, #4626, .T. ) ;
#9799=DIRECTION ( 'NONE',  ( 0.4224988092984258703, 0.5670050759397237128, 0.7071067811865479058 ) ) ;
#9800=AXIS2_PLACEMENT_3D ( 'NONE', #4185, #9144, #12301 ) ;
#9802=EDGE_CURVE ( 'NONE', #2549, #3663, #9812, .T. ) ;
#9804=LINE ( 'NONE', #11023, #2247 ) ;
#9812=CIRCLE ( 'NONE', #10047, 9.974999999999999645 ) ;
#9813=CARTESIAN_POINT ( 'NONE',  ( -17.73437360760467030, -13.24520873212868644, 51.00231026484399166 ) ) ;
#9815=DIRECTION ( 'NONE',  ( 0.5975035461963189576, 0.8018662683283437342, 0.000000000000000000 ) ) ;
#9816=LINE ( 'NONE', #7590, #11694 ) ;
#9820=AXIS2_PLACEMENT_3D ( 'NONE', #13445, #8829, #12291 ) ;
#9821=LINE ( 'NONE', #3079, #8327 ) ;
#9822=LINE ( 'NONE', #12051, #4743 ) ;
#9825=DIRECTION ( 'NONE',  ( -0.9868311969055005850, -0.1617534816134010012, -6.946583704589984503E-16 ) ) ;
#9826=EDGE_CURVE ( 'NONE', #9434, #7024, #8589, .T. ) ;
#9829=ORIENTED_EDGE ( 'NONE', *, *, #9921, .F. ) ;
#9831=EDGE_LOOP ( 'NONE', ( #5379, #10130, #7486, #4319 ) ) ;
#9832=DIRECTION ( 'NONE',  ( -8.018662683283438208E-16, 5.975035461963189015E-16, 1.000000000000000000 ) ) ;
#9833=VECTOR ( 'NONE', #11668, 1000.000000000000000 ) ;
#9834=AXIS2_PLACEMENT_3D ( 'NONE', #11388, #11243, #5568 ) ;
#9841=CARTESIAN_POINT ( 'NONE',  ( -15.49969986081086226, -13.50737899243826767, -13.49768973515600301 ) ) ;
#9842=ORIENTED_EDGE ( 'NONE', *, *, #4215, .T. ) ;
#9843=CARTESIAN_POINT ( 'NONE',  ( -21.45979773411920277, -21.50599501901345434, 54.00231026484399166 ) ) ;
#9846=EDGE_LOOP ( 'NONE', ( #9955, #3923, #12451, #7704 ) ) ;
#9847=EDGE_CURVE ( 'NONE', #14164, #12982, #9804, .T. ) ;
#9850=EDGE_LOOP ( 'NONE', ( #12389, #3826, #319, #2274 ) ) ;
#9853=DIRECTION ( 'NONE',  ( -0.9472588896649086765, 0.3204693369899911382, -9.510565162951535624E-16 ) ) ;
#9854=VECTOR ( 'NONE', #12981, 1000.000000000000227 ) ;
#9859=DIRECTION ( 'NONE',  ( -0.1511109077013120527, -0.9885168150181793401, 4.694715627858928842E-16 ) ) ;
#9861=ORIENTED_EDGE ( 'NONE', *, *, #6443, .F. ) ;
#9862=DIRECTION ( 'NONE',  ( -8.018662683283438208E-16, 5.975035461963189015E-16, 1.000000000000000000 ) ) ;
#9863=CARTESIAN_POINT ( 'NONE',  ( -24.88854884048805971, -16.87637585156647191, 56.85231026484398598 ) ) ;
#9867=ORIENTED_EDGE ( 'NONE', *, *, #1201, .F. ) ;
#9870=DIRECTION ( 'NONE',  ( -8.018662683283439195E-16, 5.975035461963190001E-16, 1.000000000000000000 ) ) ;
#9871=ORIENTED_EDGE ( 'NONE', *, *, #14953, .T. ) ;
#9872=CARTESIAN_POINT ( 'NONE',  ( -20.45368390747784204, -7.130130991507916072, 56.85231026484398598 ) ) ;
#9873=LINE ( 'NONE', #475, #9893 ) ;
#9879=DIRECTION ( 'NONE',  ( -0.9183863840214729901, -0.3956847857120157075, -4.999999999999999402E-16 ) ) ;
#9880=DIRECTION ( 'NONE',  ( -0.2536112499260171349, -0.9673062255102895524, 3.746065934159117949E-16 ) ) ;
#9881=VERTEX_POINT ( 'NONE', #2921 ) ;
#9883=LINE ( 'NONE', #4293, #12060 ) ;
#9884=ORIENTED_EDGE ( 'NONE', *, *, #7855, .F. ) ;
#9886=CARTESIAN_POINT ( 'NONE',  ( -15.45378054160984682, -13.48759475315262613, 56.85231026484398598 ) ) ;
#9887=ORIENTED_EDGE ( 'NONE', *, *, #3746, .T. ) ;
#9888=LINE ( 'NONE', #2779, #2916 ) ;
#9889=EDGE_CURVE ( 'NONE', #12295, #15022, #2004, .T. ) ;
#9890=CARTESIAN_POINT ( 'NONE',  ( -14.95642007119156425, -3.547184613301258782, 56.85231026484398598 ) ) ;
#9893=VECTOR ( 'NONE', #14394, 1000.000000000000227 ) ;
#9894=FACE_OUTER_BOUND ( 'NONE', #2649, .T. ) ;
#9896=ORIENTED_EDGE ( 'NONE', *, *, #9346, .F. ) ;
#9899=CARTESIAN_POINT ( 'NONE',  ( -15.47224238247604511, -13.54916519690201149, 56.85231026484398598 ) ) ;
#9901=EDGE_LOOP ( 'NONE', ( #12803, #4374, #9011, #3260 ) ) ;
#9905=ADVANCED_FACE ( 'NONE', ( #6492 ), #6645, .T. ) ;
#9907=CARTESIAN_POINT ( 'NONE',  ( -16.73644428586259636, -23.40541355628490550, 56.85231026484400019 ) ) ;
#9908=EDGE_CURVE ( 'NONE', #7829, #12833, #6570, .T. ) ;
#9910=DIRECTION ( 'NONE',  ( -8.018662683283438208E-16, 5.975035461963189015E-16, 1.000000000000000000 ) ) ;
#9911=DIRECTION ( 'NONE',  ( 8.018662683283438208E-16, -5.975035461963189015E-16, -1.000000000000000000 ) ) ;
#9912=ORIENTED_EDGE ( 'NONE', *, *, #11245, .F. ) ;
#9913=CARTESIAN_POINT ( 'NONE',  ( -12.93661424846659358, -15.26135318755250658, 57.00231026484399166 ) ) ;
#9914=PLANE ( 'NONE',  #1674 ) ;
#9917=AXIS2_PLACEMENT_3D ( 'NONE', #6399, #7551, #13680 ) ;
#9918=DIRECTION ( 'NONE',  ( -0.9354976265738682573, 0.3533329742249642913, -9.612616959383187437E-16 ) ) ;
#9919=VERTEX_POINT ( 'NONE', #11329 ) ;
#9921=EDGE_CURVE ( 'NONE', #5844, #8821, #13702, .T. ) ;
#9926=ORIENTED_EDGE ( 'NONE', *, *, #4106, .F. ) ;
#9927=CARTESIAN_POINT ( 'NONE',  ( -15.04562126104788966, -5.444807279564146896, 56.85231026484398598 ) ) ;
#9929=VERTEX_POINT ( 'NONE', #4220 ) ;
#9930=DIRECTION ( 'NONE',  ( -0.9316361277244830097, -0.3633925226508256667, -5.299192642332049884E-16 ) ) ;
#9932=VERTEX_POINT ( 'NONE', #854 ) ;
#9933=EDGE_CURVE ( 'NONE', #5474, #2549, #699, .T. ) ;
#9934=CARTESIAN_POINT ( 'NONE',  ( -11.55238169831532957, -21.67927775123549594, 56.85231026484400019 ) ) ;
#9935=ORIENTED_EDGE ( 'NONE', *, *, #1574, .T. ) ;
#9937=CARTESIAN_POINT ( 'NONE',  ( -21.29301345516119071, -7.881655252552254964, 56.85231026484398598 ) ) ;
#9943=VECTOR ( 'NONE', #10002, 1000.000000000000114 ) ;
#9948=ORIENTED_EDGE ( 'NONE', *, *, #5212, .T. ) ;
#9951=ORIENTED_EDGE ( 'NONE', *, *, #13293, .T. ) ;
#9953=PLANE ( 'NONE',  #6875 ) ;
#9955=ORIENTED_EDGE ( 'NONE', *, *, #8675, .F. ) ;
#9956=LINE ( 'NONE', #9813, #11468 ) ;
#9957=AXIS2_PLACEMENT_3D ( 'NONE', #3750, #4904, #13389 ) ;
#9958=CARTESIAN_POINT ( 'NONE',  ( -12.23206416678372932, -4.082773856353237640, 57.00231026484397745 ) ) ;
#9959=VECTOR ( 'NONE', #10496, 1000.000000000000227 ) ;
#9962=LINE ( 'NONE', #6511, #6367 ) ;
#9963=LINE ( 'NONE', #13426, #4249 ) ;
#9970=AXIS2_PLACEMENT_3D ( 'NONE', #6860, #9316, #2429 ) ;
#9972=ORIENTED_EDGE ( 'NONE', *, *, #7938, .T. ) ;
#9974=EDGE_CURVE ( 'NONE', #8450, #1455, #3374, .T. ) ;
#9975=VECTOR ( 'NONE', #12046, 1000.000000000000227 ) ;
#9977=DIRECTION ( 'NONE',  ( -8.018662683283438208E-16, 5.975035461963189015E-16, 1.000000000000000000 ) ) ;
#9979=DIRECTION ( 'NONE',  ( 8.018662683283438208E-16, -5.975035461963189015E-16, -1.000000000000000000 ) ) ;
#9981=ORIENTED_EDGE ( 'NONE', *, *, #5208, .T. ) ;
#9982=CARTESIAN_POINT ( 'NONE',  ( -7.426192534185826588, -13.67980128487994129, 56.85231026484400019 ) ) ;
#9983=AXIS2_PLACEMENT_3D ( 'NONE', #8802, #6777, #12619 ) ;
#9984=CARTESIAN_POINT ( 'NONE',  ( -22.54723635769173384, -9.564857042577559199, 57.00231026484397745 ) ) ;
#9986=EDGE_CURVE ( 'NONE', #13349, #1855, #4439, .T. ) ;
#9987=DIRECTION ( 'NONE',  ( -8.018662683283438208E-16, 5.975035461963189015E-16, 1.000000000000000000 ) ) ;
#9988=EDGE_CURVE ( 'NONE', #14495, #5451, #13489, .T. ) ;
#9989=DIRECTION ( 'NONE',  ( 0.5975035461963189576, 0.8018662683283437342, 0.000000000000000000 ) ) ;
#9992=VECTOR ( 'NONE', #538, 1000.000000000000000 ) ;
#9993=ADVANCED_FACE ( 'NONE', ( #8410 ), #8095, .T. ) ;
#9994=DIRECTION ( 'NONE',  ( -8.018662683283438208E-16, 5.975035461963189015E-16, 1.000000000000000000 ) ) ;
#9996=EDGE_CURVE ( 'NONE', #13839, #14554, #2380, .T. ) ;
#10000=CARTESIAN_POINT ( 'NONE',  ( -20.19618812003464470, -21.27295997720514720, 57.00231026484397745 ) ) ;
#10002=DIRECTION ( 'NONE',  ( 0.9983330752162417054, 0.05771543059946734194, 7.660444431189781397E-16 ) ) ;
#10004=ADVANCED_FACE ( 'NONE', ( #2225 ), #9410, .F. ) ;
#10006=ORIENTED_EDGE ( 'NONE', *, *, #10952, .T. ) ;
#10008=ORIENTED_EDGE ( 'NONE', *, *, #5462, .F. ) ;
#10010=DIRECTION ( 'NONE',  ( 0.7032868978765995926, 0.7109061395677416240, 1.391731009600651544E-16 ) ) ;
#10012=LINE ( 'NONE', #9872, #7378 ) ;
#10014=DIRECTION ( 'NONE',  ( 8.018662683283438208E-16, -5.975035461963189015E-16, -1.000000000000000000 ) ) ;
#10022=ORIENTED_EDGE ( 'NONE', *, *, #9847, .F. ) ;
#10023=ORIENTED_EDGE ( 'NONE', *, *, #7655, .T. ) ;
#10024=LINE ( 'NONE', #13415, #3476 ) ;
#10025=CARTESIAN_POINT ( 'NONE',  ( -15.49969986081092088, -13.50737899243822504, 56.85231026484398598 ) ) ;
#10030=EDGE_CURVE ( 'NONE', #3205, #9069, #14235, .T. ) ;
#10032=EDGE_CURVE ( 'NONE', #11873, #642, #11523, .T. ) ;
#10034=CARTESIAN_POINT ( 'NONE',  ( -22.42051587769119791, -8.443926053929422082, 56.85231026484398598 ) ) ;
#10037=FACE_OUTER_BOUND ( 'NONE', #11185, .T. ) ;
#10038=ORIENTED_EDGE ( 'NONE', *, *, #15052, .F. ) ;
#10039=ORIENTED_EDGE ( 'NONE', *, *, #9357, .F. ) ;
#10040=VECTOR ( 'NONE', #4929, 1000.000000000000000 ) ;
#10042=ORIENTED_EDGE ( 'NONE', *, *, #9529, .F. ) ;
#10043=LINE ( 'NONE', #8822, #11056 ) ;
#10045=AXIS2_PLACEMENT_3D ( 'NONE', #14874, #4395, #13724 ) ;
#10047=AXIS2_PLACEMENT_3D ( 'NONE', #10958, #3840, #12031 ) ;
#10048=ADVANCED_FACE ( 'NONE', ( #2527 ), #1301, .F. ) ;
#10053=EDGE_LOOP ( 'NONE', ( #2604, #7366, #7025, #501 ) ) ;
#10054=CARTESIAN_POINT ( 'NONE',  ( -22.67472226038933059, -17.21206232108429290, 56.85231026484398598 ) ) ;
#10056=VERTEX_POINT ( 'NONE', #6027 ) ;
#10060=AXIS2_PLACEMENT_3D ( 'NONE', #14985, #6480, #8083 ) ;
#10061=CARTESIAN_POINT ( 'NONE',  ( -6.424455519809837867, -13.54187755947681993, 56.85231026484400019 ) ) ;
#10062=ORIENTED_EDGE ( 'NONE', *, *, #9064, .T. ) ;
#10063=DIRECTION ( 'NONE',  ( 0.2301973227387160703, -0.9731439732146149879, 7.660444431189776467E-16 ) ) ;
#10064=VECTOR ( 'NONE', #8601, 1000.000000000000000 ) ;
#10065=VECTOR ( 'NONE', #7321, 1000.000000000000227 ) ;
#10066=DIRECTION ( 'NONE',  ( 0.5975035461963188466, 0.8018662683283437342, 0.000000000000000000 ) ) ;
#10067=EDGE_CURVE ( 'NONE', #572, #4418, #6374, .T. ) ;
#10069=VECTOR ( 'NONE', #12971, 1000.000000000000000 ) ;
#10071=DIRECTION ( 'NONE',  ( -8.018662683283439195E-16, 5.975035461963190001E-16, 1.000000000000000000 ) ) ;
#10073=ADVANCED_FACE ( 'NONE', ( #9487 ), #11701, .T. ) ;
#10074=ORIENTED_EDGE ( 'NONE', *, *, #9531, .F. ) ;
#10077=VERTEX_POINT ( 'NONE', #14158 ) ;
#10079=ORIENTED_EDGE ( 'NONE', *, *, #194, .T. ) ;
#10080=ORIENTED_EDGE ( 'NONE', *, *, #1952, .F. ) ;
#10081=PLANE ( 'NONE',  #7130 ) ;
#10084=AXIS2_PLACEMENT_3D ( 'NONE', #8252, #3520, #14156 ) ;
#10086=VECTOR ( 'NONE', #7906, 1000.000000000000000 ) ;
#10087=LINE ( 'NONE', #4284, #14297 ) ;
#10089=FACE_OUTER_BOUND ( 'NONE', #9582, .T. ) ;
#10093=DIRECTION ( 'NONE',  ( -0.4224988092984258703, -0.5670050759397237128, -0.7071067811865479058 ) ) ;
#10095=ORIENTED_EDGE ( 'NONE', *, *, #6848, .F. ) ;
#10096=CARTESIAN_POINT ( 'NONE',  ( -23.59621936791819863, -19.33378413377805671, 56.85231026484398598 ) ) ;
#10097=ORIENTED_EDGE ( 'NONE', *, *, #2874, .F. ) ;
#10107=ADVANCED_FACE ( 'NONE', ( #11222 ), #739, .F. ) ;
#10108=DIRECTION ( 'NONE',  ( 8.018662683283438208E-16, -5.975035461963189015E-16, -1.000000000000000000 ) ) ;
#10110=CARTESIAN_POINT ( 'NONE',  ( -15.49969986081092088, -13.50737899243822504, 57.00231026484397745 ) ) ;
#10111=VERTEX_POINT ( 'NONE', #14738 ) ;
#10113=ORIENTED_EDGE ( 'NONE', *, *, #7914, .T. ) ;
#10115=EDGE_LOOP ( 'NONE', ( #14608, #14908, #7535, #3319 ) ) ;
#10117=VECTOR ( 'NONE', #1877, 1000.000000000000227 ) ;
#10119=ORIENTED_EDGE ( 'NONE', *, *, #13819, .T. ) ;
#10121=ADVANCED_FACE ( 'NONE', ( #11291 ), #13093, .F. ) ;
#10123=DIRECTION ( 'NONE',  ( 0.5975035461963189576, 0.8018662683283437342, 0.000000000000000000 ) ) ;
#10126=UNCERTAINTY_MEASURE_WITH_UNIT (LENGTH_MEASURE( 1.000000000000000082E-05 ), #5799, 'distance_accuracy_value', 'NONE');
#10127=LINE ( 'NONE', #5250, #4503 ) ;
#10128=CARTESIAN_POINT ( 'NONE',  ( -12.87131257180735844, -22.19373785326158099, 57.00231026484399166 ) ) ;
#10130=ORIENTED_EDGE ( 'NONE', *, *, #11585, .T. ) ;
#10131=DIRECTION ( 'NONE',  ( 0.3533329742249643468, 0.9354976265738682573, -2.756373558169988945E-16 ) ) ;
#10132=CARTESIAN_POINT ( 'NONE',  ( -12.25471857405102405, -7.219983152459794162, 56.85231026484398598 ) ) ;
#10135=PLANE ( 'NONE',  #6391 ) ;
#10137=DIRECTION ( 'NONE',  ( -0.9673062255102924389, 0.2536112499260064768, -9.271838545667833343E-16 ) ) ;
#10138=EDGE_LOOP ( 'NONE', ( #11625, #4975, #12222, #14556 ) ) ;
#10140=EDGE_CURVE ( 'NONE', #1022, #6106, #14385, .T. ) ;
#10143=LINE ( 'NONE', #8999, #12391 ) ;
#10145=LINE ( 'NONE', #904, #14281 ) ;
#10146=ORIENTED_EDGE ( 'NONE', *, *, #11650, .F. ) ;
#10147=DIRECTION ( 'NONE',  ( 0.5975035461963189576, 0.8018662683283437342, 0.000000000000000000 ) ) ;
#10148=VECTOR ( 'NONE', #12687, 1000.000000000000114 ) ;
#10151=LINE ( 'NONE', #13613, #9610 ) ;
#10152=VERTEX_POINT ( 'NONE', #316 ) ;
#10154=ADVANCED_FACE ( 'NONE', ( #10867 ), #3105, .F. ) ;
#10155=LINE ( 'NONE', #11466, #13494 ) ;
#10157=ADVANCED_FACE ( 'NONE', ( #10936 ), #4259, .F. ) ;
#10159=DIRECTION ( 'NONE',  ( 0.5975035461963188466, 0.8018662683283438453, 0.000000000000000000 ) ) ;
#10164=CARTESIAN_POINT ( 'NONE',  ( -15.49969986081091733, -13.50737899243822682, 54.00231026484399166 ) ) ;
#10165=DIRECTION ( 'NONE',  ( -8.018662683283438208E-16, 5.975035461963189015E-16, 1.000000000000000000 ) ) ;
#10169=EDGE_LOOP ( 'NONE', ( #12900, #9447, #5394, #3305 ) ) ;
#10172=EDGE_LOOP ( 'NONE', ( #7158, #3373, #646, #6104 ) ) ;
#10173=EDGE_LOOP ( 'NONE', ( #6257, #9180, #14255, #1930 ) ) ;
#10174=EDGE_CURVE ( 'NONE', #11198, #11272, #783, .T. ) ;
#10175=CARTESIAN_POINT ( 'NONE',  ( -13.18491133144367211, -15.23222315862922827, 56.89875687425072215 ) ) ;
#10177=VERTEX_POINT ( 'NONE', #14812 ) ;
#10178=AXIS2_PLACEMENT_3D ( 'NONE', #873, #11646, #5679 ) ;
#10180=EDGE_CURVE ( 'NONE', #6478, #13190, #12448, .T. ) ;
#10181=VECTOR ( 'NONE', #6311, 1000.000000000000000 ) ;
#10185=ORIENTED_EDGE ( 'NONE', *, *, #11975, .F. ) ;
#10186=CARTESIAN_POINT ( 'NONE',  ( -22.04595456446742929, -18.23578246029658345, 56.85231026484398598 ) ) ;
#10188=CARTESIAN_POINT ( 'NONE',  ( -15.49969986081092088, -13.50737899243822504, 57.00231026484397745 ) ) ;
#10189=EDGE_LOOP ( 'NONE', ( #1211, #14860, #5547, #2364 ) ) ;
#10193=ORIENTED_EDGE ( 'NONE', *, *, #3115, .F. ) ;
#10194=VERTEX_POINT ( 'NONE', #8485 ) ;
#10196=ADVANCED_FACE ( 'NONE', ( #1965 ), #10135, .F. ) ;
#10200=VECTOR ( 'NONE', #7666, 1000.000000000000000 ) ;
#10201=CARTESIAN_POINT ( 'NONE',  ( -16.42437072798637843, -22.03270794722917714, 56.85231026484400019 ) ) ;
#10203=FACE_OUTER_BOUND ( 'NONE', #11381, .T. ) ;
#10204=CARTESIAN_POINT ( 'NONE',  ( -13.95777467540137806, -22.45074059323463089, 56.85231026484400019 ) ) ;
#10211=ORIENTED_EDGE ( 'NONE', *, *, #14593, .T. ) ;
#10212=CARTESIAN_POINT ( 'NONE',  ( -10.16926643994361967, -19.57302854922115287, 57.00231026484399166 ) ) ;
#10213=CARTESIAN_POINT ( 'NONE',  ( -19.38713143869018296, -6.429305403720261936, 56.85231026484398598 ) ) ;
#10216=DIRECTION ( 'NONE',  ( -0.3204693369899890287, -0.9472588896649093426, 3.090169943749498472E-16 ) ) ;
#10218=CARTESIAN_POINT ( 'NONE',  ( -18.15085299098534222, -14.64962258016358376, 51.25231026484399166 ) ) ;
#10219=LINE ( 'NONE', #14894, #3018 ) ;
#10222=VECTOR ( 'NONE', #3628, 1000.000000000000114 ) ;
#10223=AXIS2_PLACEMENT_3D ( 'NONE', #7538, #1729, #13594 ) ;
#10227=VECTOR ( 'NONE', #5789, 1000.000000000000000 ) ;
#10231=CARTESIAN_POINT ( 'NONE',  ( -15.49969986081091378, -13.50737899243822859, 51.00231026484399166 ) ) ;
#10235=DIRECTION ( 'NONE',  ( -0.1165201156931293391, -0.9931883319083343320, 4.999999999999998416E-16 ) ) ;
#10239=EDGE_LOOP ( 'NONE', ( #8079, #10487, #2171, #8897 ) ) ;
#10240=CARTESIAN_POINT ( 'NONE',  ( -15.49969986081092088, -13.50737899243822504, 56.85231026484398598 ) ) ;
#10242=VECTOR ( 'NONE', #6203, 1000.000000000000000 ) ;
#10245=DIRECTION ( 'NONE',  ( -0.9966498018049937402, 0.08178736187251965661, -8.480480961564258050E-16 ) ) ;
#10247=EDGE_CURVE ( 'NONE', #12486, #13092, #15035, .T. ) ;
#10253=DIRECTION ( 'NONE',  ( -0.8018662683283436232, 0.5975035461963189576, -9.999999999999998805E-16 ) ) ;
#10254=EDGE_LOOP ( 'NONE', ( #13059, #2621, #675, #49 ) ) ;
#10257=ORIENTED_EDGE ( 'NONE', *, *, #12945, .F. ) ;
#10261=VERTEX_POINT ( 'NONE', #12602 ) ;
#10263=CARTESIAN_POINT ( 'NONE',  ( -22.67472226038933059, -17.21206232108429290, 57.00231026484397745 ) ) ;
#10264=ADVANCED_FACE ( 'NONE', ( #11665 ), #3413, .F. ) ;
#10271=CARTESIAN_POINT ( 'NONE',  ( -17.05536012119625866, -6.605120582739408164, 57.00231026484397745 ) ) ;
#10272=ORIENTED_EDGE ( 'NONE', *, *, #13085, .F. ) ;
#10273=DIRECTION ( 'NONE',  ( -0.4177292884839972076, -0.9085715390340231012, 2.079116908177588539E-16 ) ) ;
#10276=LINE ( 'NONE', #2249, #12505 ) ;
#10277=ORIENTED_EDGE ( 'NONE', *, *, #11677, .T. ) ;
#10280=PLANE ( 'NONE',  #12219 ) ;
#10281=CARTESIAN_POINT ( 'NONE',  ( -15.49969986081092088, -13.50737899243822504, 57.00231026484397745 ) ) ;
#10283=ADVANCED_FACE ( 'NONE', ( #2038 ), #15110, .F. ) ;
#10284=AXIS2_PLACEMENT_3D ( 'NONE', #14336, #4565, #9217 ) ;
#10285=FACE_OUTER_BOUND ( 'NONE', #14875, .T. ) ;
#10287=ORIENTED_EDGE ( 'NONE', *, *, #568, .F. ) ;
#10291=VERTEX_POINT ( 'NONE', #3485 ) ;
#10292=CARTESIAN_POINT ( 'NONE',  ( -12.91190996461674168, -5.858263458394094236, 56.85231026484398598 ) ) ;
#10295=ORIENTED_EDGE ( 'NONE', *, *, #13526, .T. ) ;
#10298=VECTOR ( 'NONE', #4290, 1000.000000000000114 ) ;
#10299=DIRECTION ( 'NONE',  ( 0.9999272109403024578, -0.01206535623791937274, 8.090169943749475688E-16 ) ) ;
#10300=DIRECTION ( 'NONE',  ( -0.4587843131450244361, 0.8885476655824651182, -8.987940462991669572E-16 ) ) ;
#10302=CARTESIAN_POINT ( 'NONE',  ( -15.49969986081092088, -13.50737899243822504, 57.00231026484397745 ) ) ;
#10303=LINE ( 'NONE', #12611, #3780 ) ;
#10307=FACE_OUTER_BOUND ( 'NONE', #13, .T. ) ;
#10310=CIRCLE ( 'NONE', #3720, 9.974999999999999645 ) ;
#10312=DIRECTION ( 'NONE',  ( -8.018662683283439195E-16, 5.975035461963190001E-16, 1.000000000000000000 ) ) ;
#10313=ORIENTED_EDGE ( 'NONE', *, *, #7269, .T. ) ;
#10314=DIRECTION ( 'NONE',  ( 0.02283895005205794151, -0.9997391571607663341, 6.156614753256579139E-16 ) ) ;
#10315=ORIENTED_EDGE ( 'NONE', *, *, #8362, .T. ) ;
#10316=CARTESIAN_POINT ( 'NONE',  ( -22.08930316869620825, -18.17457871440291228, 57.00231026484397745 ) ) ;
#10321=AXIS2_PLACEMENT_3D ( 'NONE', #7081, #14065, #4510 ) ;
#10323=CARTESIAN_POINT ( 'NONE',  ( -12.38873450203231030, -7.152605626181999909, 56.85231026484398598 ) ) ;
#10333=VECTOR ( 'NONE', #2682, 1000.000000000000000 ) ;
#10334=PLANE ( 'NONE',  #1655 ) ;
#10338=LINE ( 'NONE', #10263, #256 ) ;
#10343=ORIENTED_EDGE ( 'NONE', *, *, #10894, .T. ) ;
#10345=ORIENTED_EDGE ( 'NONE', *, *, #5905, .F. ) ;
#10347=ORIENTED_EDGE ( 'NONE', *, *, #9802, .T. ) ;
#10350=ORIENTED_EDGE ( 'NONE', *, *, #13605, .T. ) ;
#10351=CARTESIAN_POINT ( 'NONE',  ( -9.251715890255169938, -8.391880844292892050, 56.85231026484398598 ) ) ;
#10353=ORIENTED_EDGE ( 'NONE', *, *, #6357, .T. ) ;
#10357=EDGE_CURVE ( 'NONE', #8706, #4315, #12834, .T. ) ;
#10359=VECTOR ( 'NONE', #586, 1000.000000000000000 ) ;
#10360=VECTOR ( 'NONE', #11235, 1000.000000000000114 ) ;
#10363=CARTESIAN_POINT ( 'NONE',  ( -8.701256315749452241, -15.46758698257906950, 56.85231026484400019 ) ) ;
#10364=ORIENTED_EDGE ( 'NONE', *, *, #6659, .T. ) ;
#10371=DIRECTION ( 'NONE',  ( 0.9437508163134050720, 0.3306575217771122732, 5.591929034707472732E-16 ) ) ;
#10373=PLANE ( 'NONE',  #1504 ) ;
#10375=ADVANCED_FACE ( 'NONE', ( #14275 ), #9376, .F. ) ;
#10381=EDGE_CURVE ( 'NONE', #7723, #8731, #14496, .T. ) ;
#10383=LINE ( 'NONE', #10531, #12553 ) ;
#10387=DIRECTION ( 'NONE',  ( 0.8018662683283437342, -0.5975035461963188466, 9.999999999999996833E-16 ) ) ;
#10388=LINE ( 'NONE', #2287, #8529 ) ;
#10393=DIRECTION ( 'NONE',  ( -8.018662683283438208E-16, 5.975035461963189015E-16, 1.000000000000000000 ) ) ;
#10397=PLANE ( 'NONE',  #178 ) ;
#10398=AXIS2_PLACEMENT_3D ( 'NONE', #11909, #1433, #3875 ) ;
#10399=DIRECTION ( 'NONE',  ( -8.018662683283438208E-16, 5.975035461963189015E-16, 1.000000000000000000 ) ) ;
#10401=ADVANCED_FACE ( 'NONE', ( #7600 ), #1023, .F. ) ;
#10402=CARTESIAN_POINT ( 'NONE',  ( -15.49969986081092088, -13.50737899243822504, 57.00231026484397745 ) ) ;
#10403=ORIENTED_EDGE ( 'NONE', *, *, #13424, .F. ) ;
#10404=DIRECTION ( 'NONE',  ( 0.5196486895212314439, -0.8543800322332368857, 9.271838545667882647E-16 ) ) ;
#10406=LINE ( 'NONE', #12483, #5301 ) ;
#10407=CARTESIAN_POINT ( 'NONE',  ( -18.50396719079564889, -6.011671700261853601, 56.85231026484398598 ) ) ;
#10408=ORIENTED_EDGE ( 'NONE', *, *, #1535, .F. ) ;
#10411=EDGE_LOOP ( 'NONE', ( #5636, #2526, #9411, #2567 ) ) ;
#10412=VECTOR ( 'NONE', #6791, 1000.000000000000000 ) ;
#10413=DIRECTION ( 'NONE',  ( -8.018662683283438208E-16, 5.975035461963189015E-16, 1.000000000000000000 ) ) ;
#10415=CARTESIAN_POINT ( 'NONE',  ( -8.525484111995742964, -7.700351810740323266, 56.85231026484400019 ) ) ;
#10417=VECTOR ( 'NONE', #8496, 1000.000000000000000 ) ;
#10422=VERTEX_POINT ( 'NONE', #13651 ) ;
#10423=DIRECTION ( 'NONE',  ( -8.018662683283438208E-16, 5.975035461963189015E-16, 1.000000000000000000 ) ) ;
#10424=ORIENTED_EDGE ( 'NONE', *, *, #5012, .F. ) ;
#10425=CIRCLE ( 'NONE', #10922, 9.974999999999999645 ) ;
#10426=ORIENTED_EDGE ( 'NONE', *, *, #4113, .T. ) ;
#10428=VERTEX_POINT ( 'NONE', #8275 ) ;
#10430=AXIS2_PLACEMENT_3D ( 'NONE', #10630, #13167, #6023 ) ;
#10434=CYLINDRICAL_SURFACE ( 'NONE', #8893, 4.499999999999999112 ) ;
#10436=DIRECTION ( 'NONE',  ( -8.018662683283439195E-16, 5.975035461963190001E-16, 1.000000000000000000 ) ) ;
#10437=DIRECTION ( 'NONE',  ( -0.9983330752162417054, -0.05771543059946733500, -7.660444431189782383E-16 ) ) ;
#10441=CARTESIAN_POINT ( 'NONE',  ( -15.49969986081091022, -13.50737899243823215, 46.00231026484398456 ) ) ;
#10442=ORIENTED_EDGE ( 'NONE', *, *, #8228, .T. ) ;
#10446=AXIS2_PLACEMENT_3D ( 'NONE', #6846, #12842, #11605 ) ;
#10448=EDGE_LOOP ( 'NONE', ( #12183, #5622, #13446, #11069 ) ) ;
#10450=ORIENTED_EDGE ( 'NONE', *, *, #9333, .F. ) ;
#10451=DIRECTION ( 'NONE',  ( -8.018662683283438208E-16, 5.975035461963189015E-16, 1.000000000000000000 ) ) ;
#10453=CARTESIAN_POINT ( 'NONE',  ( -25.24719169991952583, -11.38911842147176756, 57.00231026484397745 ) ) ;
#10458=DIRECTION ( 'NONE',  ( -8.018662683283438208E-16, 5.975035461963189015E-16, 1.000000000000000000 ) ) ;
#10459=EDGE_CURVE ( 'NONE', #5847, #964, #10024, .T. ) ;
#10462=CARTESIAN_POINT ( 'NONE',  ( -10.02446058099324588, -7.572113216692248017, 56.85231026484398598 ) ) ;
#10463=EDGE_CURVE ( 'NONE', #14564, #4445, #10310, .T. ) ;
#10464=LINE ( 'NONE', #8159, #11191 ) ;
#10465=PLANE ( 'NONE',  #4008 ) ;
#10469=DIRECTION ( 'NONE',  ( 8.018662683283438208E-16, -5.975035461963189015E-16, -1.000000000000000000 ) ) ;
#10470=ORIENTED_EDGE ( 'NONE', *, *, #13105, .T. ) ;
#10473=EDGE_CURVE ( 'NONE', #8967, #14193, #3147, .T. ) ;
#10475=( NAMED_UNIT ( * ) PLANE_ANGLE_UNIT ( ) SI_UNIT ( $, .RADIAN. ) );
#10477=LINE ( 'NONE', #3516, #12372 ) ;
#10479=CARTESIAN_POINT ( 'NONE',  ( -13.16883223745437448, -21.23902216335526916, 57.00231026484399166 ) ) ;
#10480=ADVANCED_FACE ( 'NONE', ( #6033 ), #10793, .F. ) ;
#10481=CARTESIAN_POINT ( 'NONE',  ( -7.902754534677060683, -18.47202114588016642, 56.85231026484400019 ) ) ;
#10484=DIRECTION ( 'NONE',  ( -8.018662683283438208E-16, 5.975035461963189015E-16, 1.000000000000000000 ) ) ;
#10487=ORIENTED_EDGE ( 'NONE', *, *, #14124, .F. ) ;
#10488=CARTESIAN_POINT ( 'NONE',  ( -8.569834614884436874, -19.36726104528708703, 56.85231026484400019 ) ) ;
#10490=ORIENTED_EDGE ( 'NONE', *, *, #8604, .T. ) ;
#10492=ORIENTED_EDGE ( 'NONE', *, *, #1118, .T. ) ;
#10493=CARTESIAN_POINT ( 'NONE',  ( -18.61476135779618346, -20.95734656753543845, 56.85231026484398598 ) ) ;
#10494=PLANE ( 'NONE',  #2817 ) ;
#10496=DIRECTION ( 'NONE',  ( 0.8018662683283436232, -0.5975035461963189576, 9.999999999999996833E-16 ) ) ;
#10498=CARTESIAN_POINT ( 'NONE',  ( -11.97987666612771207, -20.77526002325937782, 56.85231026484400019 ) ) ;
#10503=EDGE_LOOP ( 'NONE', ( #3804, #11205 ) ) ;
#10504=PLANE ( 'NONE',  #14590 ) ;
#10505=VERTEX_POINT ( 'NONE', #9647 ) ;
#10506=ORIENTED_EDGE ( 'NONE', *, *, #11461, .T. ) ;
#10508=ORIENTED_EDGE ( 'NONE', *, *, #5408, .F. ) ;
#10509=DIRECTION ( 'NONE',  ( 0.6251242923673534513, 0.7805252200231685977, 3.489949670250099574E-17 ) ) ;
#10510=EDGE_CURVE ( 'NONE', #14042, #4372, #9163, .T. ) ;
#10511=ADVANCED_FACE ( 'NONE', ( #1910 ), #9312, .T. ) ;
#10513=VECTOR ( 'NONE', #14632, 1000.000000000000000 ) ;
#10515=FACE_OUTER_BOUND ( 'NONE', #8729, .T. ) ;
#10517=ORIENTED_EDGE ( 'NONE', *, *, #3367, .T. ) ;
#10518=DIRECTION ( 'NONE',  ( 8.018662683283438208E-16, -5.975035461963189015E-16, -1.000000000000000000 ) ) ;
#10520=ORIENTED_EDGE ( 'NONE', *, *, #8872, .F. ) ;
#10523=DIRECTION ( 'NONE',  ( 0.5975035461963189576, 0.8018662683283437342, 0.000000000000000000 ) ) ;
#10524=EDGE_LOOP ( 'NONE', ( #13465, #3994, #70, #5031 ) ) ;
#10527=EDGE_CURVE ( 'NONE', #15014, #7674, #598, .T. ) ;
#10531=CARTESIAN_POINT ( 'NONE',  ( -10.90377457632059865, -6.867868786151726468, 56.85231026484398598 ) ) ;
#10537=ORIENTED_EDGE ( 'NONE', *, *, #7255, .F. ) ;
#10544=CARTESIAN_POINT ( 'NONE',  ( -21.12809094326923187, -9.219901432974651811, 56.85231026484398598 ) ) ;
#10545=SURFACE_STYLE_USAGE ( .BOTH. , #1217 ) ;
#10546=EDGE_CURVE ( 'NONE', #532, #7892, #8768, .T. ) ;
#10547=LINE ( 'NONE', #8322, #902 ) ;
#10551=CARTESIAN_POINT ( 'NONE',  ( -15.54961651457173488, -13.51026476396819831, 56.85231026484398598 ) ) ;
#10552=DIRECTION ( 'NONE',  ( -8.018662683283438208E-16, 5.975035461963189015E-16, 1.000000000000000000 ) ) ;
#10553=DIRECTION ( 'NONE',  ( -0.9755678736739583634, 0.2196982563774038943, -9.135454576426008610E-16 ) ) ;
#10559=VERTEX_POINT ( 'NONE', #7397 ) ;
#10561=CIRCLE ( 'NONE', #789, 9.974999999999999645 ) ;
#10564=AXIS2_PLACEMENT_3D ( 'NONE', #8524, #14195, #11821 ) ;
#10565=DIRECTION ( 'NONE',  ( -8.018662683283438208E-16, 5.975035461963189015E-16, 1.000000000000000000 ) ) ;
#10566=EDGE_CURVE ( 'NONE', #9137, #8638, #14227, .T. ) ;
#10568=DIRECTION ( 'NONE',  ( 0.9999272109403024578, -0.01206535623791937274, 8.090169943749475688E-16 ) ) ;
#10572=CARTESIAN_POINT ( 'NONE',  ( -12.51218212982932165, -9.498047650796509700, 54.00231026484399166 ) ) ;
#10574=VECTOR ( 'NONE', #10165, 1000.000000000000000 ) ;
#10576=EDGE_LOOP ( 'NONE', ( #10629, #11883, #11109, #11108 ) ) ;
#10578=ORIENTED_EDGE ( 'NONE', *, *, #8586, .T. ) ;
#10582=VERTEX_POINT ( 'NONE', #12002 ) ;
#10584=EDGE_CURVE ( 'NONE', #9118, #8928, #13267, .T. ) ;
#10585=EDGE_CURVE ( 'NONE', #1699, #6007, #6638, .T. ) ;
#10587=CARTESIAN_POINT ( 'NONE',  ( -15.49969986081091200, -13.50737899243823215, 48.00231026484398456 ) ) ;
#10588=EDGE_CURVE ( 'NONE', #11595, #10638, #67, .T. ) ;
#10589=CARTESIAN_POINT ( 'NONE',  ( -22.86200450971638531, -18.81376385001357932, 57.00231026484397745 ) ) ;
#10590=AXIS2_PLACEMENT_3D ( 'NONE', #12444, #6604, #3182 ) ;
#10595=CARTESIAN_POINT ( 'NONE',  ( -15.49969986081092088, -13.50737899243822504, 56.85231026484398598 ) ) ;
#10596=CARTESIAN_POINT ( 'NONE',  ( -6.726903101582546007, -11.18374239837452500, 56.85231026484400019 ) ) ;
#10597=ORIENTED_EDGE ( 'NONE', *, *, #8493, .T. ) ;
#10601=VECTOR ( 'NONE', #4966, 1000.000000000000000 ) ;
#10604=CARTESIAN_POINT ( 'NONE',  ( -13.28079301173263005, -15.16077777396758464, 51.00231026484399166 ) ) ;
#10606=DIRECTION ( 'NONE',  ( -0.9316361277244822325, -0.3633925226508277206, -5.299192642332030163E-16 ) ) ;
#10608=DIRECTION ( 'NONE',  ( -0.08178736187251967049, -0.9966498018049938512, 5.299192642332050870E-16 ) ) ;
#10609=DIRECTION ( 'NONE',  ( 0.5975035461963189576, 0.8018662683283437342, 0.000000000000000000 ) ) ;
#10610=CARTESIAN_POINT ( 'NONE',  ( -18.48721759179250412, -17.51671033407995282, 45.50231026484398456 ) ) ;
#10615=EDGE_LOOP ( 'NONE', ( #4200, #4162, #3756, #4728 ) ) ;
#10616=EDGE_CURVE ( 'NONE', #11595, #2901, #2816, .T. ) ;
#10619=PLANE ( 'NONE',  #4987 ) ;
#10624=LINE ( 'NONE', #11928, #7861 ) ;
#10628=DIRECTION ( 'NONE',  ( -8.018662683283438208E-16, 5.975035461963189015E-16, 1.000000000000000000 ) ) ;
#10629=ORIENTED_EDGE ( 'NONE', *, *, #115, .T. ) ;
#10630=CARTESIAN_POINT ( 'NONE',  ( -17.12834591918736749, -6.622385381944812188, 56.85231026484398598 ) ) ;
#10632=DIRECTION ( 'NONE',  ( 8.018662683283438208E-16, -5.975035461963189015E-16, -1.000000000000000000 ) ) ;
#10635=CARTESIAN_POINT ( 'NONE',  ( -8.162984683111186968, -16.88054299694650595, 57.00231026484399166 ) ) ;
#10638=VERTEX_POINT ( 'NONE', #8695 ) ;
#10640=EDGE_CURVE ( 'NONE', #14240, #34, #11057, .T. ) ;
#10646=CARTESIAN_POINT ( 'NONE',  ( -15.49969986081092088, -13.50737899243822504, 56.85231026484398598 ) ) ;
#10647=CARTESIAN_POINT ( 'NONE',  ( -6.766506000727597225, -11.03906478995046214, 56.85231026484400019 ) ) ;
#10649=VECTOR ( 'NONE', #129, 1000.000000000000000 ) ;
#10653=VECTOR ( 'NONE', #6849, 1000.000000000000227 ) ;
#10657=CARTESIAN_POINT ( 'NONE',  ( -21.68801466096620700, -19.44379288755867208, 56.85231026484398598 ) ) ;
#10660=EDGE_CURVE ( 'NONE', #9137, #7024, #898, .T. ) ;
#10663=CARTESIAN_POINT ( 'NONE',  ( -24.53816276005083452, -12.69040994830970703, 56.85231026484398598 ) ) ;
#10664=PLANE ( 'NONE',  #8655 ) ;
#10665=LINE ( 'NONE', #2636, #522 ) ;
#10667=ORIENTED_EDGE ( 'NONE', *, *, #8757, .T. ) ;
#10668=CARTESIAN_POINT ( 'NONE',  ( -15.19697172008446096, -10.92700001391350284, 51.00231026484399166 ) ) ;
#10676=ORIENTED_EDGE ( 'NONE', *, *, #7093, .T. ) ;
#10677=VECTOR ( 'NONE', #6738, 1000.000000000000000 ) ;
#10678=DIRECTION ( 'NONE',  ( 0.3633925226508277206, -0.9316361277244822325, 8.480480961564270869E-16 ) ) ;
#10679=AXIS2_PLACEMENT_3D ( 'NONE', #8618, #2731, #7157 ) ;
#10681=EDGE_CURVE ( 'NONE', #12259, #8545, #6397, .T. ) ;
#10682=VECTOR ( 'NONE', #7460, 1000.000000000000000 ) ;
#10683=FACE_OUTER_BOUND ( 'NONE', #2994, .T. ) ;
#10685=AXIS2_PLACEMENT_3D ( 'NONE', #1232, #2387, #14167 ) ;
#10686=ORIENTED_EDGE ( 'NONE', *, *, #14971, .F. ) ;
#10689=ORIENTED_EDGE ( 'NONE', *, *, #55, .T. ) ;
#10690=DIRECTION ( 'NONE',  ( 0.1272150336605032961, -0.9918751611018177261, 6.946583704589934213E-16 ) ) ;
#10691=CARTESIAN_POINT ( 'NONE',  ( -17.54662770128649285, -5.179934221328323929, 56.85231026484398598 ) ) ;
#10693=DIRECTION ( 'NONE',  ( 8.018662683283438208E-16, -5.975035461963189015E-16, -1.000000000000000000 ) ) ;
#10694=ORIENTED_EDGE ( 'NONE', *, *, #656, .T. ) ;
#10700=LINE ( 'NONE', #8397, #2493 ) ;
#10701=EDGE_CURVE ( 'NONE', #150, #5925, #6465, .T. ) ;
#10710=VECTOR ( 'NONE', #12471, 1000.000000000000000 ) ;
#10711=ORIENTED_EDGE ( 'NONE', *, *, #4092, .T. ) ;
#10713=ORIENTED_EDGE ( 'NONE', *, *, #2531, .F. ) ;
#10714=CARTESIAN_POINT ( 'NONE',  ( -17.91037007046713470, -11.71108944158557463, 57.00231026484397745 ) ) ;
#10717=CARTESIAN_POINT ( 'NONE',  ( -14.00164528647249007, -5.572553380472728968, 56.85231026484398598 ) ) ;
#10719=ORIENTED_EDGE ( 'NONE', *, *, #14499, .T. ) ;
#10722=VECTOR ( 'NONE', #660, 1000.000000000000000 ) ;
#10727=CARTESIAN_POINT ( 'NONE',  ( -15.49969986081092088, -13.50737899243822504, 57.00231026484397745 ) ) ;
#10728=VECTOR ( 'NONE', #8430, 1000.000000000000114 ) ;
#10730=LINE ( 'NONE', #408, #13255 ) ;
#10731=VERTEX_POINT ( 'NONE', #667 ) ;
#10735=ORIENTED_EDGE ( 'NONE', *, *, #11443, .F. ) ;
#10736=CARTESIAN_POINT ( 'NONE',  ( -23.54764701038621411, -12.84694604531765272, 56.85231026484398598 ) ) ;
#10740=ADVANCED_FACE ( 'NONE', ( #6692 ), #5333, .F. ) ;
#10741=DIRECTION ( 'NONE',  ( 0.5975035461963189576, 0.8018662683283437342, 0.000000000000000000 ) ) ;
#10742=CARTESIAN_POINT ( 'NONE',  ( -17.72286745096105065, -3.783277446994219417, 57.00231026484397745 ) ) ;
#10747=VERTEX_POINT ( 'NONE', #2959 ) ;
#10748=CARTESIAN_POINT ( 'NONE',  ( -8.639554752241616953, -9.247137322136806503, 56.85231026484400019 ) ) ;
#10751=ADVANCED_FACE ( 'NONE', ( #14744 ), #8840, .T. ) ;
#10752=CIRCLE ( 'NONE', #4154, 9.974999999999999645 ) ;
#10753=VERTEX_POINT ( 'NONE', #1894 ) ;
#10756=CARTESIAN_POINT ( 'NONE',  ( -7.145558396657058609, -18.95797028117975103, 56.85231026484400019 ) ) ;
#10761=EDGE_CURVE ( 'NONE', #9327, #6873, #4344, .T. ) ;
#10767=VECTOR ( 'NONE', #7261, 1000.000000000000000 ) ;
#10769=CARTESIAN_POINT ( 'NONE',  ( -7.731023390221355207, -11.30308411758414877, 56.85231026484400019 ) ) ;
#10783=ORIENTED_EDGE ( 'NONE', *, *, #8675, .T. ) ;
#10785=CARTESIAN_POINT ( 'NONE',  ( -15.49969986081091022, -13.50737899243823215, 45.50231026484398456 ) ) ;
#10786=DIRECTION ( 'NONE',  ( 8.018662683283439195E-16, -5.975035461963190987E-16, -1.000000000000000000 ) ) ;
#10787=VERTEX_POINT ( 'NONE', #12757 ) ;
#10788=DIRECTION ( 'NONE',  ( 0.8222303661035904598, -0.5691548339926103539, 9.993908270190959005E-16 ) ) ;
#10790=CARTESIAN_POINT ( 'NONE',  ( -23.59621936791820573, -19.33378413377806382, 57.00231026484397745 ) ) ;
#10791=ORIENTED_EDGE ( 'NONE', *, *, #1880, .T. ) ;
#10792=ORIENTED_EDGE ( 'NONE', *, *, #1065, .F. ) ;
#10793=PLANE ( 'NONE',  #12037 ) ;
#10794=EDGE_CURVE ( 'NONE', #6250, #2134, #10816, .T. ) ;
#10795=PLANE ( 'NONE',  #13263 ) ;
#10796=ORIENTED_EDGE ( 'NONE', *, *, #10030, .F. ) ;
#10800=CARTESIAN_POINT ( 'NONE',  ( -12.46042140754850003, -23.00808483377100089, 54.00231026484399166 ) ) ;
#10804=CIRCLE ( 'NONE', #2979, 9.974999999999999645 ) ;
#10805=DIRECTION ( 'NONE',  ( -0.04695496274984587576, -0.9988970074402868660, 5.591929034707467802E-16 ) ) ;
#10806=VECTOR ( 'NONE', #8674, 1000.000000000000000 ) ;
#10807=VERTEX_POINT ( 'NONE', #1048 ) ;
#10810=ORIENTED_EDGE ( 'NONE', *, *, #12328, .T. ) ;
#10812=AXIS2_PLACEMENT_3D ( 'NONE', #14147, #2669, #3669 ) ;
#10815=EDGE_CURVE ( 'NONE', #5023, #10505, #347, .T. ) ;
#10816=LINE ( 'NONE', #9299, #6127 ) ;
#10817=CARTESIAN_POINT ( 'NONE',  ( -21.23124220554638697, -20.54376104222092181, 56.85231026484398598 ) ) ;
#10820=VECTOR ( 'NONE', #4931, 1000.000000000000000 ) ;
#10821=AXIS2_PLACEMENT_3D ( 'NONE', #10647, #3839, #2544 ) ;
#10822=CARTESIAN_POINT ( 'NONE',  ( -25.44713467170207366, -12.76632185356751847, 56.85231026484398598 ) ) ;
#10825=DIRECTION ( 'NONE',  ( -8.018662683283438208E-16, 5.975035461963189015E-16, 1.000000000000000000 ) ) ;
#10826=FACE_OUTER_BOUND ( 'NONE', #5075, .T. ) ;
#10832=CARTESIAN_POINT ( 'NONE',  ( -25.24719169991952228, -11.38911842147176934, 54.00231026484397745 ) ) ;
#10833=VECTOR ( 'NONE', #9326, 1000.000000000000227 ) ;
#10834=ADVANCED_FACE ( 'NONE', ( #5007 ), #10373, .F. ) ;
#10835=VECTOR ( 'NONE', #9057, 1000.000000000000000 ) ;
#10836=CARTESIAN_POINT ( 'NONE',  ( -18.43409448121630945, -5.984417261063049942, 56.85231026484398598 ) ) ;
#10838=EDGE_CURVE ( 'NONE', #3312, #6835, #7280, .T. ) ;
#10840=CARTESIAN_POINT ( 'NONE',  ( -10.96544185377836911, -6.825182173602284408, 56.85231026484398598 ) ) ;
#10843=DIRECTION ( 'NONE',  ( -8.018662683283438208E-16, 5.975035461963189015E-16, 1.000000000000000000 ) ) ;
#10845=VERTEX_POINT ( 'NONE', #263 ) ;
#10846=EDGE_CURVE ( 'NONE', #11369, #560, #6054, .T. ) ;
#10848=EDGE_CURVE ( 'NONE', #551, #2842, #15039, .T. ) ;
#10849=DIRECTION ( 'NONE',  ( -8.018662683283438208E-16, 5.975035461963189015E-16, 1.000000000000000000 ) ) ;
#10851=DIRECTION ( 'NONE',  ( 8.018662683283438208E-16, -5.975035461963189015E-16, -1.000000000000000000 ) ) ;
#10853=ORIENTED_EDGE ( 'NONE', *, *, #2051, .F. ) ;
#10855=EDGE_CURVE ( 'NONE', #14217, #8353, #12680, .T. ) ;
#10856=VECTOR ( 'NONE', #7726, 1000.000000000000227 ) ;
#10858=EDGE_CURVE ( 'NONE', #4089, #8967, #11599, .T. ) ;
#10864=LINE ( 'NONE', #392, #14374 ) ;
#10866=ORIENTED_EDGE ( 'NONE', *, *, #7187, .T. ) ;
#10867=FACE_OUTER_BOUND ( 'NONE', #7968, .T. ) ;
#10869=EDGE_CURVE ( 'NONE', #7124, #9677, #4930, .T. ) ;
#10871=LINE ( 'NONE', #2605, #9114 ) ;
#10872=ORIENTED_EDGE ( 'NONE', *, *, #6272, .F. ) ;
#10873=ORIENTED_EDGE ( 'NONE', *, *, #8963, .F. ) ;
#10874=CARTESIAN_POINT ( 'NONE',  ( -15.36741682587554969, -22.58172476492607572, 57.00231026484399166 ) ) ;
#10880=DIRECTION ( 'NONE',  ( -0.8772189822852964891, 0.4800904676395363335, -9.902680687415702019E-16 ) ) ;
#10881=ADVANCED_FACE ( 'NONE', ( #3778 ), #7203, .F. ) ;
#10883=ORIENTED_EDGE ( 'NONE', *, *, #1808, .T. ) ;
#10884=EDGE_LOOP ( 'NONE', ( #10890, #5123, #3430, #7557 ) ) ;
#10886=ORIENTED_EDGE ( 'NONE', *, *, #4839, .F. ) ;
#10887=ORIENTED_EDGE ( 'NONE', *, *, #8035, .F. ) ;
#10888=CARTESIAN_POINT ( 'NONE',  ( -13.02562488396841900, -21.19439421350821817, 56.85231026484400019 ) ) ;
#10889=VERTEX_POINT ( 'NONE', #11964 ) ;
#10890=ORIENTED_EDGE ( 'NONE', *, *, #6848, .T. ) ;
#10891=CARTESIAN_POINT ( 'NONE',  ( -20.33437667196779586, -7.039214636791314206, 56.85231026484398598 ) ) ;
#10894=EDGE_CURVE ( 'NONE', #9624, #13913, #13642, .T. ) ;
#10895=VECTOR ( 'NONE', #1595, 1000.000000000000000 ) ;
#10896=CARTESIAN_POINT ( 'NONE',  ( -9.565488148413143321, -20.37370125056455095, 56.85231026484400019 ) ) ;
#10897=DIRECTION ( 'NONE',  ( 0.7582332219680881780, -0.6519834208811539078, 9.975640502598240034E-16 ) ) ;
#10899=ORIENTED_EDGE ( 'NONE', *, *, #14809, .F. ) ;
#10900=CARTESIAN_POINT ( 'NONE',  ( -11.97987666612771207, -20.77526002325937782, 57.00231026484399166 ) ) ;
#10904=CARTESIAN_POINT ( 'NONE',  ( -22.70654572567255158, -20.40389968624656802, 56.85231026484398598 ) ) ;
#10906=VECTOR ( 'NONE', #10399, 1000.000000000000000 ) ;
#10908=EDGE_CURVE ( 'NONE', #12295, #9104, #868, .T. ) ;
#10910=DIRECTION ( 'NONE',  ( -8.018662683283438208E-16, 5.975035461963189015E-16, 1.000000000000000000 ) ) ;
#10912=EDGE_CURVE ( 'NONE', #9643, #3619, #11697, .T. ) ;
#10915=CIRCLE ( 'NONE', #1631, 9.974999999999999645 ) ;
#10917=ORIENTED_EDGE ( 'NONE', *, *, #787, .T. ) ;
#10918=DIRECTION ( 'NONE',  ( -8.018662683283438208E-16, 5.975035461963189015E-16, 1.000000000000000000 ) ) ;
#10919=ORIENTED_EDGE ( 'NONE', *, *, #2248, .F. ) ;
#10920=CARTESIAN_POINT ( 'NONE',  ( -8.569834614884436874, -19.36726104528708703, 57.00231026484399166 ) ) ;
#10921=VERTEX_POINT ( 'NONE', #12421 ) ;
#10922=AXIS2_PLACEMENT_3D ( 'NONE', #13430, #3163, #6364 ) ;
#10924=CARTESIAN_POINT ( 'NONE',  ( -9.760873592531986276, -5.348549538251085700, 56.85231026484398598 ) ) ;
#10925=VECTOR ( 'NONE', #10843, 1000.000000000000000 ) ;
#10927=DIRECTION ( 'NONE',  ( 0.2536112499260171349, 0.9673062255102895524, -3.746065934159117949E-16 ) ) ;
#10928=AXIS2_PLACEMENT_3D ( 'NONE', #6314, #1440, #2812 ) ;
#10931=EDGE_CURVE ( 'NONE', #8222, #10056, #3592, .T. ) ;
#10935=VERTEX_POINT ( 'NONE', #10479 ) ;
#10936=FACE_OUTER_BOUND ( 'NONE', #13281, .T. ) ;
#10937=EDGE_LOOP ( 'NONE', ( #12218, #13326, #11628, #1233 ) ) ;
#10938=CIRCLE ( 'NONE', #8244, 9.974999999999999645 ) ;
#10939=CIRCLE ( 'NONE', #4595, 9.974999999999999645 ) ;
#10940=DIRECTION ( 'NONE',  ( -8.018662683283438208E-16, 5.975035461963189015E-16, 1.000000000000000000 ) ) ;
#10942=EDGE_CURVE ( 'NONE', #6707, #7319, #8, .T. ) ;
#10945=AXIS2_PLACEMENT_3D ( 'NONE', #14129, #13975, #8301 ) ;
#10946=LINE ( 'NONE', #5349, #3236 ) ;
#10947=EDGE_LOOP ( 'NONE', ( #3919, #10119, #11945, #10959 ) ) ;
#10949=ADVANCED_FACE ( 'NONE', ( #7885 ), #83, .T. ) ;
#10952=EDGE_CURVE ( 'NONE', #8100, #9600, #6662, .T. ) ;
#10955=DIRECTION ( 'NONE',  ( -0.8018662683283436232, 0.5975035461963189576, -9.999999999999996833E-16 ) ) ;
#10958=CARTESIAN_POINT ( 'NONE',  ( -15.49969986081092088, -13.50737899243822504, 57.00231026484397745 ) ) ;
#10959=ORIENTED_EDGE ( 'NONE', *, *, #7914, .F. ) ;
#10961=DIRECTION ( 'NONE',  ( 8.018662683283438208E-16, -5.975035461963189015E-16, -1.000000000000000000 ) ) ;
#10963=VERTEX_POINT ( 'NONE', #8174 ) ;
#10968=CARTESIAN_POINT ( 'NONE',  ( -8.162984683111186968, -16.88054299694650595, 56.85231026484400019 ) ) ;
#10969=CARTESIAN_POINT ( 'NONE',  ( -15.51120972694785749, -13.45872179377749589, 56.85231026484398598 ) ) ;
#10970=DIRECTION ( 'NONE',  ( 0.5975035461963188466, 0.8018662683283437342, 0.000000000000000000 ) ) ;
#10973=DIRECTION ( 'NONE',  ( -8.018662683283438208E-16, 5.975035461963189015E-16, 1.000000000000000000 ) ) ;
#10975=LINE ( 'NONE', #12351, #15065 ) ;
#10976=ORIENTED_EDGE ( 'NONE', *, *, #3830, .T. ) ;
#10979=ORIENTED_EDGE ( 'NONE', *, *, #12935, .T. ) ;
#10980=VECTOR ( 'NONE', #14212, 1000.000000000000000 ) ;
#10983=PLANE ( 'NONE',  #2561 ) ;
#10986=AXIS2_PLACEMENT_3D ( 'NONE', #5337, #748, #14746 ) ;
#10991=DIRECTION ( 'NONE',  ( 0.5975035461963188466, 0.8018662683283437342, 0.000000000000000000 ) ) ;
#10992=ORIENTED_EDGE ( 'NONE', *, *, #9017, .F. ) ;
#10994=LINE ( 'NONE', #2587, #4577 ) ;
#10996=DIRECTION ( 'NONE',  ( -0.9673062255102896634, 0.2536112499260171904, -9.271838545667876730E-16 ) ) ;
#10997=ORIENTED_EDGE ( 'NONE', *, *, #934, .T. ) ;
#10998=EDGE_CURVE ( 'NONE', #6817, #14904, #14861, .T. ) ;
#11000=CARTESIAN_POINT ( 'NONE',  ( -15.49969986081092088, -13.50737899243822504, 57.00231026484397745 ) ) ;
#11002=LINE ( 'NONE', #13088, #11876 ) ;
#11006=DIRECTION ( 'NONE',  ( 0.9931883319083343320, -0.1165201156931293391, 8.660254037844386422E-16 ) ) ;
#11008=ORIENTED_EDGE ( 'NONE', *, *, #9145, .T. ) ;
#11010=ORIENTED_EDGE ( 'NONE', *, *, #3284, .T. ) ;
#11012=ADVANCED_FACE ( 'NONE', ( #4235 ), #7733, .T. ) ;
#11013=FACE_OUTER_BOUND ( 'NONE', #8547, .T. ) ;
#11016=CARTESIAN_POINT ( 'NONE',  ( -24.28571865450477674, -8.784403367172062715, 57.00231026484397745 ) ) ;
#11020=DIRECTION ( 'NONE',  ( 0.5975035461963188466, 0.8018662683283437342, 0.000000000000000000 ) ) ;
#11021=LINE ( 'NONE', #6420, #9592 ) ;
#11022=VERTEX_POINT ( 'NONE', #355 ) ;
#11023=CARTESIAN_POINT ( 'NONE',  ( -15.14850084941412511, -4.438867027711355107, 56.85231026484398598 ) ) ;
#11028=EDGE_CURVE ( 'NONE', #2807, #7478, #10665, .T. ) ;
#11030=ADVANCED_FACE ( 'NONE', ( #7135 ), #7364, .F. ) ;
#11032=VECTOR ( 'NONE', #2077, 1000.000000000000000 ) ;
#11033=DIRECTION ( 'NONE',  ( -8.018662683283438208E-16, 5.975035461963189015E-16, 1.000000000000000000 ) ) ;
#11034=LINE ( 'NONE', #8734, #10513 ) ;
#11035=CARTESIAN_POINT ( 'NONE',  ( -7.506093261461533217, -14.65346081099998088, 56.85231026484400019 ) ) ;
#11038=VECTOR ( 'NONE', #8202, 1000.000000000000000 ) ;
#11042=CARTESIAN_POINT ( 'NONE',  ( -12.51218212982931810, -9.498047650796513253, 45.50231026484398456 ) ) ;
#11043=DIRECTION ( 'NONE',  ( -0.8719950447285823580, -0.4895147004624046394, -4.067366430758000189E-16 ) ) ;
#11044=ORIENTED_EDGE ( 'NONE', *, *, #12874, .T. ) ;
#11045=DIRECTION ( 'NONE',  ( -8.018662683283438208E-16, 5.975035461963189015E-16, 1.000000000000000000 ) ) ;
#11048=ORIENTED_EDGE ( 'NONE', *, *, #4995, .F. ) ;
#11049=EDGE_LOOP ( 'NONE', ( #5238, #1696, #13357, #3823 ) ) ;
#11052=ORIENTED_EDGE ( 'NONE', *, *, #14764, .F. ) ;
#11053=DIRECTION ( 'NONE',  ( 0.2196982563774082797, 0.9755678736739573642, -4.067366430757958773E-16 ) ) ;
#11054=CIRCLE ( 'NONE', #4457, 9.974999999999999645 ) ;
#11056=VECTOR ( 'NONE', #2592, 1000.000000000000000 ) ;
#11057=CIRCLE ( 'NONE', #14968, 9.974999999999999645 ) ;
#11063=EDGE_CURVE ( 'NONE', #4396, #10787, #196, .T. ) ;
#11066=VERTEX_POINT ( 'NONE', #11974 ) ;
#11068=LINE ( 'NONE', #591, #4862 ) ;
#11069=ORIENTED_EDGE ( 'NONE', *, *, #7186, .F. ) ;
#11070=VECTOR ( 'NONE', #5961, 1000.000000000000000 ) ;
#11071=DIRECTION ( 'NONE',  ( 0.08178736187250883194, 0.9966498018049948504, -5.299192642332142575E-16 ) ) ;
#11072=VERTEX_POINT ( 'NONE', #9672 ) ;
#11073=CARTESIAN_POINT ( 'NONE',  ( -21.11416342254291934, -20.63752968607602867, 57.00231026484397745 ) ) ;
#11074=EDGE_LOOP ( 'NONE', ( #738, #9554, #3545, #14081 ) ) ;
#11076=CARTESIAN_POINT ( 'NONE',  ( -18.48721759179251123, -17.51671033407994926, 51.00031026484398922 ) ) ;
#11079=EDGE_CURVE ( 'NONE', #2590, #5603, #3856, .T. ) ;
#11081=CARTESIAN_POINT ( 'NONE',  ( -15.53608329785963527, -13.54167542823733328, 56.85231026484398598 ) ) ;
#11088=EDGE_LOOP ( 'NONE', ( #2952, #8686, #11802, #5657 ) ) ;
#11089=ORIENTED_EDGE ( 'NONE', *, *, #729, .F. ) ;
#11091=DIRECTION ( 'NONE',  ( -8.018662683283438208E-16, 5.975035461963189015E-16, 1.000000000000000000 ) ) ;
#11093=DIRECTION ( 'NONE',  ( 0.9805849309054470719, 0.1960948578651654506, 6.691306063588581484E-16 ) ) ;
#11096=CARTESIAN_POINT ( 'NONE',  ( -24.21370508435883551, -8.652820519829271362, 54.00231026484397745 ) ) ;
#11097=FACE_OUTER_BOUND ( 'NONE', #13043, .T. ) ;
#11098=CIRCLE ( 'NONE', #6677, 9.974999999999999645 ) ;
#11099=EDGE_CURVE ( 'NONE', #4500, #3108, #9055, .T. ) ;
#11100=LINE ( 'NONE', #12477, #6998 ) ;
#11103=ORIENTED_EDGE ( 'NONE', *, *, #13153, .T. ) ;
#11104=DIRECTION ( 'NONE',  ( -0.8415927028326163351, 0.5401126942952662047, -9.975640502598247923E-16 ) ) ;
#11107=CARTESIAN_POINT ( 'NONE',  ( -14.15531688186919723, -11.70317988869945580, 51.00231026484399166 ) ) ;
#11108=ORIENTED_EDGE ( 'NONE', *, *, #14021, .F. ) ;
#11109=ORIENTED_EDGE ( 'NONE', *, *, #656, .F. ) ;
#11111=DIRECTION ( 'NONE',  ( -8.018662683283438208E-16, 5.975035461963189015E-16, 1.000000000000000000 ) ) ;
#11112=EDGE_LOOP ( 'NONE', ( #5217, #1443, #6012, #9261 ) ) ;
#11114=VECTOR ( 'NONE', #3832, 1000.000000000000000 ) ;
#11116=LINE ( 'NONE', #13274, #11946 ) ;
#11120=DIRECTION ( 'NONE',  ( -0.2196982563774038943, -0.9755678736739584744, 4.067366430757998709E-16 ) ) ;
#11122=ADVANCED_FACE ( 'NONE', ( #8962 ), #5378, .T. ) ;
#11124=LINE ( 'NONE', #719, #14604 ) ;
#11127=ORIENTED_EDGE ( 'NONE', *, *, #1865, .T. ) ;
#11130=CARTESIAN_POINT ( 'NONE',  ( -15.49969986081092088, -13.50737899243822504, 56.85231026484398598 ) ) ;
#11132=ADVANCED_FACE ( 'NONE', ( #497 ), #4009, .F. ) ;
#11136=EDGE_CURVE ( 'NONE', #3490, #13967, #14443, .T. ) ;
#11138=EDGE_CURVE ( 'NONE', #9794, #337, #9962, .T. ) ;
#11144=DIRECTION ( 'NONE',  ( 0.5975035461963188466, 0.8018662683283437342, 0.000000000000000000 ) ) ;
#11145=EDGE_LOOP ( 'NONE', ( #1478, #9063, #10783, #14353 ) ) ;
#11147=VECTOR ( 'NONE', #11154, 1000.000000000000000 ) ;
#11148=DIRECTION ( 'NONE',  ( 0.1617534816134024167, -0.9868311969055004740, 7.193398003386505973E-16 ) ) ;
#11149=ORIENTED_EDGE ( 'NONE', *, *, #12346, .F. ) ;
#11151=EDGE_CURVE ( 'NONE', #10963, #10056, #9821, .T. ) ;
#11154=DIRECTION ( 'NONE',  ( -8.018662683283438208E-16, 5.975035461963189015E-16, 1.000000000000000000 ) ) ;
#11155=CARTESIAN_POINT ( 'NONE',  ( -7.223083447440863836, -17.23012942000294245, 57.00231026484399166 ) ) ;
#11160=ORIENTED_EDGE ( 'NONE', *, *, #13100, .F. ) ;
#11161=DIRECTION ( 'NONE',  ( -8.018662683283438208E-16, 5.975035461963189015E-16, 1.000000000000000000 ) ) ;
#11162=ORIENTED_EDGE ( 'NONE', *, *, #2264, .T. ) ;
#11163=VERTEX_POINT ( 'NONE', #11042 ) ;
#11165=VECTOR ( 'NONE', #7240, 1000.000000000000000 ) ;
#11166=LINE ( 'NONE', #11389, #10710 ) ;
#11167=EDGE_CURVE ( 'NONE', #14533, #4396, #3701, .T. ) ;
#11168=EDGE_CURVE ( 'NONE', #8839, #9541, #13573, .T. ) ;
#11169=CARTESIAN_POINT ( 'NONE',  ( -16.41401162527548507, -4.478243707298169340, 56.85231026484398598 ) ) ;
#11174=DIRECTION ( 'NONE',  ( -0.6519834208811554621, -0.7582332219680868457, -6.975647374412761332E-17 ) ) ;
#11178=AXIS2_PLACEMENT_3D ( 'NONE', #6948, #10608, #11831 ) ;
#11181=VERTEX_POINT ( 'NONE', #7593 ) ;
#11182=DIRECTION ( 'NONE',  ( -0.8934395198752397294, 0.4491835085186243748, -9.848077530122081084E-16 ) ) ;
#11184=VERTEX_POINT ( 'NONE', #6438 ) ;
#11185=EDGE_LOOP ( 'NONE', ( #5776, #13907, #13706, #2081 ) ) ;
#11186=LINE ( 'NONE', #7876, #15085 ) ;
#11187=LINE ( 'NONE', #3871, #8153 ) ;
#11188=ORIENTED_EDGE ( 'NONE', *, *, #4963, .T. ) ;
#11189=CARTESIAN_POINT ( 'NONE',  ( -7.691420491076302213, -11.44776172600821340, 56.85231026484400019 ) ) ;
#11191=VECTOR ( 'NONE', #12849, 999.9999999999998863 ) ;
#11192=VECTOR ( 'NONE', #7909, 1000.000000000000000 ) ;
#11194=CIRCLE ( 'NONE', #4598, 9.974999999999999645 ) ;
#11195=LINE ( 'NONE', #564, #705 ) ;
#11198=VERTEX_POINT ( 'NONE', #8894 ) ;
#11199=DIRECTION ( 'NONE',  ( 0.6780482080269577549, 0.7350174335289139105, 1.045284632676540317E-16 ) ) ;
#11205=ORIENTED_EDGE ( 'NONE', *, *, #11311, .F. ) ;
#11208=ADVANCED_FACE ( 'NONE', ( #12272 ), #5450, .F. ) ;
#11210=VECTOR ( 'NONE', #420, 1000.000000000000000 ) ;
#11211=ADVANCED_FACE ( 'NONE', ( #9894 ), #8738, .F. ) ;
#11212=DIRECTION ( 'NONE',  ( 0.9354976265738677021, -0.3533329742249661232, 9.612616959383195326E-16 ) ) ;
#11213=CARTESIAN_POINT ( 'NONE',  ( -23.39388780995641781, -11.80648316271623877, 56.85231026484398598 ) ) ;
#11220=FACE_OUTER_BOUND ( 'NONE', #3218, .T. ) ;
#11221=VERTEX_POINT ( 'NONE', #14788 ) ;
#11222=FACE_OUTER_BOUND ( 'NONE', #5154, .T. ) ;
#11227=ADVANCED_FACE ( 'NONE', ( #13498 ), #3008, .F. ) ;
#11230=VECTOR ( 'NONE', #3151, 1000.000000000000000 ) ;
#11235=DIRECTION ( 'NONE',  ( -0.9547156899063192759, -0.2975196656469966672, -5.877852522924767272E-16 ) ) ;
#11236=VERTEX_POINT ( 'NONE', #3458 ) ;
#11238=DIRECTION ( 'NONE',  ( -0.7109061395677416240, 0.7032868978765995926, -9.902680687415702019E-16 ) ) ;
#11239=ORIENTED_EDGE ( 'NONE', *, *, #747, .T. ) ;
#11240=LINE ( 'NONE', #1907, #1802 ) ;
#11243=DIRECTION ( 'NONE',  ( 8.018662683283438208E-16, -5.975035461963189015E-16, -1.000000000000000000 ) ) ;
#11245=EDGE_CURVE ( 'NONE', #4906, #13839, #12808, .T. ) ;
#11247=DIRECTION ( 'NONE',  ( -0.5975035461963187355, -0.8018662683283438453, 0.000000000000000000 ) ) ;
#11249=LINE ( 'NONE', #921, #5773 ) ;
#11251=CARTESIAN_POINT ( 'NONE',  ( -8.162984683111186968, -16.88054299694650595, 56.85231026484400019 ) ) ;
#11253=CARTESIAN_POINT ( 'NONE',  ( -7.594860258898399330, -10.18326093375929631, 56.85231026484400019 ) ) ;
#11255=VECTOR ( 'NONE', #329, 1000.000000000000000 ) ;
#11257=DIRECTION ( 'NONE',  ( -8.018662683283438208E-16, 5.975035461963189015E-16, 1.000000000000000000 ) ) ;
#11259=ORIENTED_EDGE ( 'NONE', *, *, #619, .F. ) ;
#11264=DIRECTION ( 'NONE',  ( -8.018662683283438208E-16, 5.975035461963189015E-16, 1.000000000000000000 ) ) ;
#11266=EDGE_CURVE ( 'NONE', #1475, #14941, #557, .T. ) ;
#11267=DIRECTION ( 'NONE',  ( 8.018662683283438208E-16, -5.975035461963189015E-16, -1.000000000000000000 ) ) ;
#11272=VERTEX_POINT ( 'NONE', #12729 ) ;
#11274=VECTOR ( 'NONE', #13206, 1000.000000000000227 ) ;
#11276=ORIENTED_EDGE ( 'NONE', *, *, #3647, .T. ) ;
#11278=CARTESIAN_POINT ( 'NONE',  ( -23.05384319539488658, -10.65421522557165623, 56.85231026484398598 ) ) ;
#11281=VECTOR ( 'NONE', #3522, 1000.000000000000000 ) ;
#11284=EDGE_CURVE ( 'NONE', #8725, #7674, #12655, .T. ) ;
#11285=CARTESIAN_POINT ( 'NONE',  ( -16.39856880423293006, -20.52544743201270450, 56.85231026484400019 ) ) ;
#11288=CARTESIAN_POINT ( 'NONE',  ( -24.93814746875458610, -16.73481322911949931, 56.85231026484398598 ) ) ;
#11291=FACE_OUTER_BOUND ( 'NONE', #5294, .T. ) ;
#11293=VECTOR ( 'NONE', #6980, 1000.000000000000114 ) ;
#11295=VECTOR ( 'NONE', #12855, 1000.000000000000000 ) ;
#11301=DIRECTION ( 'NONE',  ( -0.3633925226508256667, 0.9316361277244830097, -8.480480961564259036E-16 ) ) ;
#11304=CARTESIAN_POINT ( 'NONE',  ( -15.51120972694785749, -13.45872179377749589, 56.85231026484398598 ) ) ;
#11308=CARTESIAN_POINT ( 'NONE',  ( -24.06473463808513813, -13.92741382918746496, 56.85231026484398598 ) ) ;
#11311=EDGE_CURVE ( 'NONE', #7355, #13071, #2998, .T. ) ;
#11316=CARTESIAN_POINT ( 'NONE',  ( -15.21745595230144232, -22.57829892241827352, 56.85231026484400019 ) ) ;
#11317=ADVANCED_FACE ( 'NONE', ( #4387 ), #9040, .F. ) ;
#11319=DIRECTION ( 'NONE',  ( 0.9472588896649092316, -0.3204693369899889732, 9.510565162951523791E-16 ) ) ;
#11321=DIRECTION ( 'NONE',  ( -8.018662683283438208E-16, 5.975035461963189015E-16, 1.000000000000000000 ) ) ;
#11323=CARTESIAN_POINT ( 'NONE',  ( -17.81448839017816965, -11.78253482624722182, 56.75231026484397745 ) ) ;
#11324=EDGE_CURVE ( 'NONE', #14274, #9541, #7346, .T. ) ;
#11327=LINE ( 'NONE', #14844, #12533 ) ;
#11329=CARTESIAN_POINT ( 'NONE',  ( -5.966797098401854349, -16.44411015522000241, 57.00231026484399166 ) ) ;
#11333=VERTEX_POINT ( 'NONE', #3615 ) ;
#11334=ORIENTED_EDGE ( 'NONE', *, *, #1501, .T. ) ;
#11336=CARTESIAN_POINT ( 'NONE',  ( -20.65541546412893226, -22.04665423204159325, 54.00231026484399166 ) ) ;
#11337=ORIENTED_EDGE ( 'NONE', *, *, #1952, .T. ) ;
#11338=LINE ( 'NONE', #6727, #6079 ) ;
#11343=( BOUNDED_CURVE ( )  B_SPLINE_CURVE ( 3, ( #3438, #4666, #156, #13998 ),
 .UNSPECIFIED., .F., .F. ) 
 B_SPLINE_CURVE_WITH_KNOTS ( ( 4, 4 ),
 ( 3.141592653589792228, 4.712388980384688786 ),
 .UNSPECIFIED. ) 
 CURVE ( )  GEOMETRIC_REPRESENTATION_ITEM ( )  RATIONAL_B_SPLINE_CURVE ( ( 1.000000000000000000, 0.8047378541243649375, 0.8047378541243649375, 1.000000000000000000 ) ) 
 REPRESENTATION_ITEM ( '' )  );
#11344=CARTESIAN_POINT ( 'NONE',  ( -6.517576446443361426, -14.80457171870128974, 56.85231026484400019 ) ) ;
#11345=AXIS2_PLACEMENT_3D ( 'NONE', #6214, #1562, #6062 ) ;
#11347=ORIENTED_EDGE ( 'NONE', *, *, #3938, .T. ) ;
#11349=ORIENTED_EDGE ( 'NONE', *, *, #2708, .F. ) ;
#11350=LINE ( 'NONE', #3245, #10677 ) ;
#11351=ORIENTED_EDGE ( 'NONE', *, *, #2573, .F. ) ;
#11352=ORIENTED_EDGE ( 'NONE', *, *, #159, .T. ) ;
#11365=ORIENTED_EDGE ( 'NONE', *, *, #9404, .F. ) ;
#11369=VERTEX_POINT ( 'NONE', #8348 ) ;
#11371=DIRECTION ( 'NONE',  ( 8.018662683283438208E-16, -5.975035461963189015E-16, -1.000000000000000000 ) ) ;
#11372=CARTESIAN_POINT ( 'NONE',  ( -17.54761070396351741, -21.31837676343380750, 56.85231026484400019 ) ) ;
#11373=ORIENTED_EDGE ( 'NONE', *, *, #10588, .F. ) ;
#11375=EDGE_CURVE ( 'NONE', #8725, #5040, #13110, .T. ) ;
#11376=DIRECTION ( 'NONE',  ( 8.018662683283438208E-16, -5.975035461963189015E-16, -1.000000000000000000 ) ) ;
#11377=CARTESIAN_POINT ( 'NONE',  ( -23.59767874945767119, -17.60420555931063902, 57.00231026484397745 ) ) ;
#11378=CARTESIAN_POINT ( 'NONE',  ( -17.54761070396351741, -21.31837676343380750, 56.85231026484400019 ) ) ;
#11379=DIRECTION ( 'NONE',  ( 0.3533329742249663452, 0.9354976265738675911, -2.756373558169968730E-16 ) ) ;
#11380=VECTOR ( 'NONE', #799, 1000.000000000000000 ) ;
#11381=EDGE_LOOP ( 'NONE', ( #3809, #14256, #14182, #4069 ) ) ;
#11384=ORIENTED_EDGE ( 'NONE', *, *, #5632, .T. ) ;
#11387=ORIENTED_EDGE ( 'NONE', *, *, #11908, .T. ) ;
#11388=CARTESIAN_POINT ( 'NONE',  ( -15.49969986081092088, -13.50737899243822504, 56.85231026484398598 ) ) ;
#11389=CARTESIAN_POINT ( 'NONE',  ( -10.02446058099324766, -7.572113216692248017, 57.00231026484397745 ) ) ;
#11390=ADVANCED_FACE ( 'NONE', ( #1323 ), #3692, .T. ) ;
#11391=CARTESIAN_POINT ( 'NONE',  ( -12.91190996461674168, -5.858263458394094236, 56.85231026484398598 ) ) ;
#11393=CIRCLE ( 'NONE', #14329, 9.974999999999999645 ) ;
#11395=CARTESIAN_POINT ( 'NONE',  ( -21.05979293892203330, -6.334749421441233430, 57.00231026484397745 ) ) ;
#11396=DIRECTION ( 'NONE',  ( -0.5975035461963188466, -0.8018662683283439563, 0.000000000000000000 ) ) ;
#11399=CARTESIAN_POINT ( 'NONE',  ( -23.54290256004220439, -7.607589560680598773, 56.85231026484398598 ) ) ;
#11402=VECTOR ( 'NONE', #7011, 1000.000000000000000 ) ;
#11403=ORIENTED_EDGE ( 'NONE', *, *, #11866, .F. ) ;
#11404=CARTESIAN_POINT ( 'NONE',  ( -8.972439834930606040, -10.77678811232731348, 57.00231026484399166 ) ) ;
#11405=ORIENTED_EDGE ( 'NONE', *, *, #4296, .T. ) ;
#11406=ORIENTED_EDGE ( 'NONE', *, *, #1603, .F. ) ;
#11408=ORIENTED_EDGE ( 'NONE', *, *, #13881, .F. ) ;
#11409=AXIS2_PLACEMENT_3D ( 'NONE', #8898, #3085, #8742 ) ;
#11410=CARTESIAN_POINT ( 'NONE',  ( -15.54961651457173488, -13.51026476396819831, 56.85231026484398598 ) ) ;
#11415=DIRECTION ( 'NONE',  ( -0.4587843131450204948, 0.8885476655824671166, -8.987940462991649850E-16 ) ) ;
#11418=DIRECTION ( 'NONE',  ( 0.8357240892757724637, 0.5491495666976171641, 3.420201433256690644E-16 ) ) ;
#11420=VERTEX_POINT ( 'NONE', #6200 ) ;
#11421=FACE_OUTER_BOUND ( 'NONE', #11145, .T. ) ;
#11423=PLANE ( 'NONE',  #10178 ) ;
#11424=ORIENTED_EDGE ( 'NONE', *, *, #13542, .T. ) ;
#11429=AXIS2_PLACEMENT_3D ( 'NONE', #1416, #10518, #5916 ) ;
#11431=ADVANCED_FACE ( 'NONE', ( #6045 ), #7038, .F. ) ;
#11433=VECTOR ( 'NONE', #6867, 1000.000000000000000 ) ;
#11434=FACE_OUTER_BOUND ( 'NONE', #6123, .T. ) ;
#11440=ORIENTED_EDGE ( 'NONE', *, *, #8527, .T. ) ;
#11443=EDGE_CURVE ( 'NONE', #8638, #9137, #7145, .T. ) ;
#11446=ORIENTED_EDGE ( 'NONE', *, *, #1666, .F. ) ;
#11448=AXIS2_PLACEMENT_3D ( 'NONE', #6291, #14413, #9745 ) ;
#11449=VECTOR ( 'NONE', #5396, 1000.000000000000000 ) ;
#11457=ORIENTED_EDGE ( 'NONE', *, *, #5391, .F. ) ;
#11459=DIRECTION ( 'NONE',  ( 0.4800904676395346127, 0.8772189822852974883, -1.391731009600680140E-16 ) ) ;
#11460=CARTESIAN_POINT ( 'NONE',  ( -15.49969986081092088, -13.50737899243822504, 57.00231026484397745 ) ) ;
#11461=EDGE_CURVE ( 'NONE', #8254, #12986, #11872, .T. ) ;
#11463=VERTEX_POINT ( 'NONE', #8426 ) ;
#11464=CARTESIAN_POINT ( 'NONE',  ( -15.12969879992303746, -10.35358246313022335, 57.00231026484397745 ) ) ;
#11465=EDGE_LOOP ( 'NONE', ( #3263, #14419, #14449, #12145 ) ) ;
#11466=CARTESIAN_POINT ( 'NONE',  ( -13.26502611401716081, -13.76954925274777253, 51.00231026484399166 ) ) ;
#11467=CARTESIAN_POINT ( 'NONE',  ( -15.49969986081091378, -13.50737899243822859, 51.00231026484399166 ) ) ;
#11468=VECTOR ( 'NONE', #14410, 1000.000000000000000 ) ;
#11469=AXIS2_PLACEMENT_3D ( 'NONE', #8458, #4798, #5928 ) ;
#11475=CARTESIAN_POINT ( 'NONE',  ( -23.41792317787242084, -15.09084496969942535, 56.85231026484398598 ) ) ;
#11476=ADVANCED_FACE ( 'NONE', ( #2617 ), #6652, .T. ) ;
#11477=VERTEX_POINT ( 'NONE', #407 ) ;
#11479=ORIENTED_EDGE ( 'NONE', *, *, #13016, .T. ) ;
#11480=CARTESIAN_POINT ( 'NONE',  ( -17.62015867087677634, -21.29935591968936137, 56.85231026484400019 ) ) ;
#11481=LINE ( 'NONE', #1999, #13768 ) ;
#11482=ORIENTED_EDGE ( 'NONE', *, *, #8312, .T. ) ;
#11483=ORIENTED_EDGE ( 'NONE', *, *, #1407, .T. ) ;
#11486=CARTESIAN_POINT ( 'NONE',  ( -10.95221305062249684, -4.629260458021021485, 57.00231026484397745 ) ) ;
#11487=ORIENTED_EDGE ( 'NONE', *, *, #11952, .T. ) ;
#11489=LINE ( 'NONE', #12725, #2946 ) ;
#11496=EDGE_CURVE ( 'NONE', #5981, #10261, #11743, .T. ) ;
#11497=EDGE_LOOP ( 'NONE', ( #7587, #15114 ) ) ;
#11500=ORIENTED_EDGE ( 'NONE', *, *, #7905, .T. ) ;
#11502=ORIENTED_EDGE ( 'NONE', *, *, #1632, .T. ) ;
#11504=EDGE_CURVE ( 'NONE', #2864, #1781, #12105, .T. ) ;
#11505=DIRECTION ( 'NONE',  ( 0.9316361277244830097, 0.3633925226508256667, 5.299192642332049884E-16 ) ) ;
#11507=VECTOR ( 'NONE', #3158, 1000.000000000000000 ) ;
#11509=DIRECTION ( 'NONE',  ( 0.5975035461963188466, 0.8018662683283437342, 0.000000000000000000 ) ) ;
#11511=ORIENTED_EDGE ( 'NONE', *, *, #7971, .T. ) ;
#11512=DIRECTION ( 'NONE',  ( -8.018662683283438208E-16, 5.975035461963189015E-16, 1.000000000000000000 ) ) ;
#11513=EDGE_CURVE ( 'NONE', #1909, #13227, #1767, .T. ) ;
#11514=EDGE_CURVE ( 'NONE', #4715, #9010, #13260, .T. ) ;
#11515=LINE ( 'NONE', #12750, #7883 ) ;
#11518=ADVANCED_FACE ( 'NONE', ( #4142 ), #6347, .T. ) ;
#11519=LINE ( 'NONE', #893, #3968 ) ;
#11520=CARTESIAN_POINT ( 'NONE',  ( -24.03943920472178775, -16.57887731378902885, 56.85231026484398598 ) ) ;
#11521=ORIENTED_EDGE ( 'NONE', *, *, #3746, .F. ) ;
#11523=CIRCLE ( 'NONE', #1253, 9.974999999999999645 ) ;
#11526=EDGE_CURVE ( 'NONE', #6877, #2831, #4063, .T. ) ;
#11528=DIRECTION ( 'NONE',  ( 0.5975035461963189576, 0.8018662683283437342, 0.000000000000000000 ) ) ;
#11532=ORIENTED_EDGE ( 'NONE', *, *, #4947, .F. ) ;
#11535=CARTESIAN_POINT ( 'NONE',  ( -10.90377457632059865, -6.867868786151726468, 56.85231026484398598 ) ) ;
#11537=VECTOR ( 'NONE', #1927, 1000.000000000000114 ) ;
#11538=AXIS2_PLACEMENT_3D ( 'NONE', #15125, #6936, #11545 ) ;
#11539=LINE ( 'NONE', #15054, #10227 ) ;
#11541=CARTESIAN_POINT ( 'NONE',  ( -7.490307934913750465, -12.48011759562962020, 56.85231026484400019 ) ) ;
#11543=CARTESIAN_POINT ( 'NONE',  ( -7.887638505697306179, -19.95386229157006497, 57.00231026484399166 ) ) ;
#11544=LINE ( 'NONE', #7082, #685 ) ;
#11545=DIRECTION ( 'NONE',  ( 0.5975035461963188466, 0.8018662683283437342, 0.000000000000000000 ) ) ;
#11547=VECTOR ( 'NONE', #12390, 1000.000000000000000 ) ;
#11548=EDGE_CURVE ( 'NONE', #12614, #1349, #11021, .T. ) ;
#11551=CARTESIAN_POINT ( 'NONE',  ( -15.24029490235350259, -21.57855976525750563, 56.85231026484400019 ) ) ;
#11552=LINE ( 'NONE', #2221, #4114 ) ;
#11553=LINE ( 'NONE', #7866, #3491 ) ;
#11555=DIRECTION ( 'NONE',  ( 0.5975035461963189576, 0.8018662683283437342, 0.000000000000000000 ) ) ;
#11562=PLANE ( 'NONE',  #4349 ) ;
#11563=AXIS2_PLACEMENT_3D ( 'NONE', #43, #13887, #8055 ) ;
#11571=EDGE_LOOP ( 'NONE', ( #13858, #13480, #949, #7443 ) ) ;
#11574=AXIS2_PLACEMENT_3D ( 'NONE', #6598, #14655, #7756 ) ;
#11578=ORIENTED_EDGE ( 'NONE', *, *, #8138, .F. ) ;
#11582=LINE ( 'NONE', #10204, #8263 ) ;
#11583=ADVANCED_FACE ( 'NONE', ( #772 ), #14693, .F. ) ;
#11585=EDGE_CURVE ( 'NONE', #11857, #4102, #13926, .T. ) ;
#11586=VECTOR ( 'NONE', #4572, 1000.000000000000114 ) ;
#11587=CARTESIAN_POINT ( 'NONE',  ( -6.468284635389320414, -17.74225372801456757, 56.85231026484400019 ) ) ;
#11589=DIRECTION ( 'NONE',  ( -8.018662683283438208E-16, 5.975035461963189015E-16, 1.000000000000000000 ) ) ;
#11590=EDGE_LOOP ( 'NONE', ( #1472, #2111, #704, #13307 ) ) ;
#11593=ORIENTED_EDGE ( 'NONE', *, *, #3386, .T. ) ;
#11594=EDGE_CURVE ( 'NONE', #7160, #7645, #9249, .T. ) ;
#11595=VERTEX_POINT ( 'NONE', #3217 ) ;
#11597=DIRECTION ( 'NONE',  ( 0.9316361277244821215, 0.3633925226508276651, 5.299192642332029177E-16 ) ) ;
#11598=EDGE_LOOP ( 'NONE', ( #5719, #3775, #9948, #13793 ) ) ;
#11599=LINE ( 'NONE', #1116, #12012 ) ;
#11600=ADVANCED_FACE ( 'NONE', ( #5508 ), #3441, .F. ) ;
#11602=EDGE_CURVE ( 'NONE', #551, #6428, #11553, .T. ) ;
#11603=DIRECTION ( 'NONE',  ( 0.5104125104778984845, 0.8599296884906632021, -1.045284632676530333E-16 ) ) ;
#11604=ADVANCED_FACE ( 'NONE', ( #2075 ), #13625, .F. ) ;
#11605=DIRECTION ( 'NONE',  ( -0.9918751611018171710, -0.1272150336605082366, -7.193398003386512876E-16 ) ) ;
#11608=VERTEX_POINT ( 'NONE', #11399 ) ;
#11611=DIRECTION ( 'NONE',  ( 0.5975035461963189576, 0.8018662683283437342, 0.000000000000000000 ) ) ;
#11613=ORIENTED_EDGE ( 'NONE', *, *, #4422, .F. ) ;
#11615=ORIENTED_EDGE ( 'NONE', *, *, #4497, .F. ) ;
#11624=CARTESIAN_POINT ( 'NONE',  ( -9.401538680480957311, -6.786242167561306715, 56.85231026484398598 ) ) ;
#11625=ORIENTED_EDGE ( 'NONE', *, *, #13195, .T. ) ;
#11626=CARTESIAN_POINT ( 'NONE',  ( -10.72806301968316411, -20.63252684047564500, 56.85231026484400019 ) ) ;
#11628=ORIENTED_EDGE ( 'NONE', *, *, #7217, .T. ) ;
#11629=EDGE_CURVE ( 'NONE', #12982, #8725, #7793, .T. ) ;
#11630=ORIENTED_EDGE ( 'NONE', *, *, #2819, .T. ) ;
#11632=DIRECTION ( 'NONE',  ( -8.018662683283439195E-16, 5.975035461963190001E-16, 1.000000000000000000 ) ) ;
#11633=ORIENTED_EDGE ( 'NONE', *, *, #6273, .F. ) ;
#11634=CIRCLE ( 'NONE', #6245, 4.500000000000000000 ) ;
#11640=VECTOR ( 'NONE', #2122, 1000.000000000000114 ) ;
#11641=CARTESIAN_POINT ( 'NONE',  ( -16.58783302151896777, -10.98181643637917304, 56.75231026484397745 ) ) ;
#11645=ORIENTED_EDGE ( 'NONE', *, *, #6844, .F. ) ;
#11646=DIRECTION ( 'NONE',  ( -0.6601155939154574881, 0.7511640317997414495, -9.781476007338062700E-16 ) ) ;
#11649=ORIENTED_EDGE ( 'NONE', *, *, #6558, .F. ) ;
#11650=EDGE_CURVE ( 'NONE', #11072, #5306, #4442, .T. ) ;
#11655=DIRECTION ( 'NONE',  ( 0.5975035461963189576, 0.8018662683283437342, 0.000000000000000000 ) ) ;
#11657=LINE ( 'NONE', #8134, #2772 ) ;
#11659=VERTEX_POINT ( 'NONE', #12479 ) ;
#11661=CIRCLE ( 'NONE', #7981, 9.974999999999999645 ) ;
#11662=DIRECTION ( 'NONE',  ( -8.018662683283438208E-16, 5.975035461963189015E-16, 1.000000000000000000 ) ) ;
#11663=ORIENTED_EDGE ( 'NONE', *, *, #15072, .T. ) ;
#11664=VERTEX_POINT ( 'NONE', #3297 ) ;
#11665=FACE_OUTER_BOUND ( 'NONE', #9901, .T. ) ;
#11666=EDGE_CURVE ( 'NONE', #13942, #7657, #5203, .T. ) ;
#11667=VECTOR ( 'NONE', #9223, 1000.000000000000000 ) ;
#11668=DIRECTION ( 'NONE',  ( 8.018662683283438208E-16, -5.975035461963189015E-16, -1.000000000000000000 ) ) ;
#11669=ORIENTED_EDGE ( 'NONE', *, *, #3176, .T. ) ;
#11674=AXIS2_PLACEMENT_3D ( 'NONE', #10595, #11817, #2340 ) ;
#11676=VECTOR ( 'NONE', #693, 1000.000000000000000 ) ;
#11677=EDGE_CURVE ( 'NONE', #1582, #2365, #1995, .T. ) ;
#11679=CARTESIAN_POINT ( 'NONE',  ( -20.39403028972282428, -7.084672814149619136, 56.85231026484398598 ) ) ;
#11681=CARTESIAN_POINT ( 'NONE',  ( -6.507973901336479017, -12.27851192488648024, 57.00231026484399166 ) ) ;
#11682=CARTESIAN_POINT ( 'NONE',  ( -20.44787060326519423, -4.846187890544671362, 56.85231026484398598 ) ) ;
#11685=CARTESIAN_POINT ( 'NONE',  ( -12.32172653804166096, -7.186294389320899256, 57.00231026484397745 ) ) ;
#11686=EDGE_CURVE ( 'NONE', #8808, #13353, #11327, .T. ) ;
#11687=ORIENTED_EDGE ( 'NONE', *, *, #9889, .T. ) ;
#11688=DIRECTION ( 'NONE',  ( 0.9673062255102897744, -0.2536112499260168573, 9.271838545667874758E-16 ) ) ;
#11689=ORIENTED_EDGE ( 'NONE', *, *, #10908, .F. ) ;
#11690=DIRECTION ( 'NONE',  ( 0.5975035461963188466, 0.8018662683283437342, 0.000000000000000000 ) ) ;
#11691=LINE ( 'NONE', #12782, #2407 ) ;
#11692=CARTESIAN_POINT ( 'NONE',  ( -21.45979773411920277, -21.50599501901345434, 57.00231026484397745 ) ) ;
#11694=VECTOR ( 'NONE', #14483, 999.9999999999998863 ) ;
#11695=LINE ( 'NONE', #1218, #11165 ) ;
#11697=LINE ( 'NONE', #12492, #7095 ) ;
#11700=EDGE_LOOP ( 'NONE', ( #6445, #135, #1245, #11424 ) ) ;
#11701=PLANE ( 'NONE',  #7362 ) ;
#11703=EDGE_CURVE ( 'NONE', #3333, #7744, #2222, .T. ) ;
#11704=VECTOR ( 'NONE', #7259, 1000.000000000000000 ) ;
#11708=VERTEX_POINT ( 'NONE', #1075 ) ;
#11710=CARTESIAN_POINT ( 'NONE',  ( -16.99345872630171428, -15.51204466325908982, 51.00231026484399166 ) ) ;
#11713=DIRECTION ( 'NONE',  ( 0.5975035461963188466, 0.8018662683283437342, 0.000000000000000000 ) ) ;
#11714=( LENGTH_UNIT ( ) NAMED_UNIT ( * ) SI_UNIT ( .MILLI., .METRE. ) );
#11719=CARTESIAN_POINT ( 'NONE',  ( -14.41156670010287577, -16.03294154849727704, 56.75231026484399166 ) ) ;
#11720=ORIENTED_EDGE ( 'NONE', *, *, #6485, .F. ) ;
#11721=CARTESIAN_POINT ( 'NONE',  ( -23.14528701667493849, -16.10665716956490812, 57.00231026484397745 ) ) ;
#11722=ORIENTED_EDGE ( 'NONE', *, *, #3080, .F. ) ;
#11724=ORIENTED_EDGE ( 'NONE', *, *, #5160, .F. ) ;
#11727=DIRECTION ( 'NONE',  ( 8.018662683283438208E-16, -5.975035461963189015E-16, -1.000000000000000000 ) ) ;
#11730=EDGE_CURVE ( 'NONE', #1022, #6280, #13037, .T. ) ;
#11735=VERTEX_POINT ( 'NONE', #7096 ) ;
#11739=VERTEX_POINT ( 'NONE', #315 ) ;
#11741=CARTESIAN_POINT ( 'NONE',  ( -9.539601987502637215, -5.508762965862999295, 54.00231026484399166 ) ) ;
#11742=ORIENTED_EDGE ( 'NONE', *, *, #7449, .T. ) ;
#11743=( BOUNDED_CURVE ( )  B_SPLINE_CURVE ( 3, ( #13479, #5433, #12401, #12254 ),
 .UNSPECIFIED., .F., .F. ) 
 B_SPLINE_CURVE_WITH_KNOTS ( ( 4, 4 ),
 ( 3.141592653589793560, 4.712388980384691450 ),
 .UNSPECIFIED. ) 
 CURVE ( )  GEOMETRIC_REPRESENTATION_ITEM ( )  RATIONAL_B_SPLINE_CURVE ( ( 1.000000000000000000, 0.8047378541243646044, 0.8047378541243646044, 1.000000000000000000 ) ) 
 REPRESENTATION_ITEM ( '' )  );
#11749=DIRECTION ( 'NONE',  ( -8.018662683283438208E-16, 5.975035461963189015E-16, 1.000000000000000000 ) ) ;
#11756=CARTESIAN_POINT ( 'NONE',  ( -15.10625462230756000, -3.540141368888815254, 54.00231026484397745 ) ) ;
#11757=VERTEX_POINT ( 'NONE', #9408 ) ;
#11758=DIRECTION ( 'NONE',  ( 0.5975035461963189576, 0.8018662683283437342, 0.000000000000000000 ) ) ;
#11761=LINE ( 'NONE', #1285, #2503 ) ;
#11762=CARTESIAN_POINT ( 'NONE',  ( -8.744338604334316756, -15.61126689213601360, 56.85231026484400019 ) ) ;
#11766=ADVANCED_FACE ( 'NONE', ( #6101 ), #14233, .T. ) ;
#11767=DIRECTION ( 'NONE',  ( -8.018662683283438208E-16, 5.975035461963189015E-16, 1.000000000000000000 ) ) ;
#11769=EDGE_CURVE ( 'NONE', #6348, #8564, #2525, .T. ) ;
#11773=EDGE_CURVE ( 'NONE', #6233, #6946, #7331, .T. ) ;
#11776=LINE ( 'NONE', #6940, #4855 ) ;
#11777=FACE_OUTER_BOUND ( 'NONE', #8860, .T. ) ;
#11778=ORIENTED_EDGE ( 'NONE', *, *, #474, .T. ) ;
#11780=EDGE_LOOP ( 'NONE', ( #13634, #450, #6947, #5898 ) ) ;
#11783=ADVANCED_FACE ( 'NONE', ( #2378 ), #7177, .T. ) ;
#11788=VECTOR ( 'NONE', #8565, 1000.000000000000000 ) ;
#11790=DIRECTION ( 'NONE',  ( -8.018662683283438208E-16, 5.975035461963189015E-16, 1.000000000000000000 ) ) ;
#11791=DIRECTION ( 'NONE',  ( -8.018662683283438208E-16, 5.975035461963189015E-16, 1.000000000000000000 ) ) ;
#11792=CARTESIAN_POINT ( 'NONE',  ( -20.60611791317904107, -19.76323582219775687, 57.00231026484397745 ) ) ;
#11794=ADVANCED_FACE ( 'NONE', ( #11777 ), #9484, .F. ) ;
#11796=LINE ( 'NONE', #14675, #3288 ) ;
#11801=DIRECTION ( 'NONE',  ( 8.018662683283438208E-16, -5.975035461963189015E-16, -1.000000000000000000 ) ) ;
#11802=ORIENTED_EDGE ( 'NONE', *, *, #13237, .F. ) ;
#11804=DIRECTION ( 'NONE',  ( 0.5975035461963188466, 0.8018662683283437342, 0.000000000000000000 ) ) ;
#11805=ORIENTED_EDGE ( 'NONE', *, *, #4626, .F. ) ;
#11808=VECTOR ( 'NONE', #7246, 1000.000000000000000 ) ;
#11810=DIRECTION ( 'NONE',  ( -8.018662683283438208E-16, 5.975035461963189015E-16, 1.000000000000000000 ) ) ;
#11811=VECTOR ( 'NONE', #3023, 1000.000000000000114 ) ;
#11813=CARTESIAN_POINT ( 'NONE',  ( -15.24029490235350259, -21.57855976525750563, 56.85231026484400019 ) ) ;
#11817=DIRECTION ( 'NONE',  ( 8.018662683283438208E-16, -5.975035461963189015E-16, -1.000000000000000000 ) ) ;
#11821=DIRECTION ( 'NONE',  ( 8.018662683283438208E-16, -5.975035461963189015E-16, -1.000000000000000000 ) ) ;
#11825=CARTESIAN_POINT ( 'NONE',  ( -24.05607732349520234, -14.07716379046991584, 56.85231026484398598 ) ) ;
#11826=EDGE_CURVE ( 'NONE', #10111, #6762, #1299, .T. ) ;
#11828=VECTOR ( 'NONE', #5786, 1000.000000000000114 ) ;
#11831=DIRECTION ( 'NONE',  ( -0.9966498018049937402, 0.08178736187251965661, -8.480480961564258050E-16 ) ) ;
#11832=CARTESIAN_POINT ( 'NONE',  ( -22.00391959472895209, -7.178368354675633611, 56.85231026484398598 ) ) ;
#11834=ORIENTED_EDGE ( 'NONE', *, *, #10067, .T. ) ;
#11835=CARTESIAN_POINT ( 'NONE',  ( -11.55178736972959896, -19.37894070656198764, 56.85231026484400019 ) ) ;
#11838=ORIENTED_EDGE ( 'NONE', *, *, #14864, .T. ) ;
#11839=LINE ( 'NONE', #11756, #13667 ) ;
#11840=ORIENTED_EDGE ( 'NONE', *, *, #11063, .F. ) ;
#11842=ORIENTED_EDGE ( 'NONE', *, *, #1201, .T. ) ;
#11843=VECTOR ( 'NONE', #14990, 1000.000000000000000 ) ;
#11844=ADVANCED_FACE ( 'NONE', ( #13091 ), #1454, .T. ) ;
#11846=PLANE ( 'NONE',  #9970 ) ;
#11849=DIRECTION ( 'NONE',  ( -0.6519834208811554621, -0.7582332219680868457, -6.975647374412761332E-17 ) ) ;
#11851=AXIS2_PLACEMENT_3D ( 'NONE', #2834, #2912, #13180 ) ;
#11856=DIRECTION ( 'NONE',  ( 0.9983330752162417054, 0.05771543059946734194, 7.660444431189781397E-16 ) ) ;
#11857=VERTEX_POINT ( 'NONE', #12013 ) ;
#11858=CARTESIAN_POINT ( 'NONE',  ( -15.49969986081092088, -13.50737899243822504, 57.00231026484397745 ) ) ;
#11866=EDGE_CURVE ( 'NONE', #4633, #12536, #12863, .T. ) ;
#11871=DIRECTION ( 'NONE',  ( 0.1165201156931293391, 0.9931883319083343320, -4.999999999999998416E-16 ) ) ;
#11872=LINE ( 'NONE', #254, #13997 ) ;
#11873=VERTEX_POINT ( 'NONE', #10096 ) ;
#11876=VECTOR ( 'NONE', #6097, 1000.000000000000000 ) ;
#11877=LINE ( 'NONE', #8431, #2853 ) ;
#11879=ORIENTED_EDGE ( 'NONE', *, *, #12415, .T. ) ;
#11881=LINE ( 'NONE', #6051, #3459 ) ;
#11882=EDGE_CURVE ( 'NONE', #12018, #10291, #9883, .T. ) ;
#11883=ORIENTED_EDGE ( 'NONE', *, *, #3273, .F. ) ;
#11884=CARTESIAN_POINT ( 'NONE',  ( -6.726903101582546007, -11.18374239837452500, 57.00231026484399166 ) ) ;
#11885=CARTESIAN_POINT ( 'NONE',  ( -9.539601987502633662, -5.508762965863001071, 51.00231026484399166 ) ) ;
#11887=LINE ( 'NONE', #10589, #10222 ) ;
#11888=VECTOR ( 'NONE', #12638, 1000.000000000000114 ) ;
#11891=CARTESIAN_POINT ( 'NONE',  ( -22.56290636796585503, -13.91571566392944526, 56.85231026484398598 ) ) ;
#11893=CARTESIAN_POINT ( 'NONE',  ( -13.09722856071139496, -21.21670818843173478, 56.85231026484400019 ) ) ;
#11894=LINE ( 'NONE', #14272, #9854 ) ;
#11895=ORIENTED_EDGE ( 'NONE', *, *, #12561, .F. ) ;
#11901=ORIENTED_EDGE ( 'NONE', *, *, #5778, .F. ) ;
#11907=VECTOR ( 'NONE', #2583, 1000.000000000000000 ) ;
#11908=EDGE_CURVE ( 'NONE', #6605, #6877, #14502, .T. ) ;
#11909=CARTESIAN_POINT ( 'NONE',  ( -15.53608329785963527, -13.54167542823733328, 56.85231026484398598 ) ) ;
#11913=FACE_OUTER_BOUND ( 'NONE', #6309, .T. ) ;
#11919=DIRECTION ( 'NONE',  ( 0.5975035461963189576, 0.8018662683283437342, 0.000000000000000000 ) ) ;
#11920=ORIENTED_EDGE ( 'NONE', *, *, #12500, .F. ) ;
#11921=CARTESIAN_POINT ( 'NONE',  ( -15.49969986081086226, -13.50737899243826767, -13.99768973515600301 ) ) ;
#11924=VECTOR ( 'NONE', #11006, 1000.000000000000000 ) ;
#11928=CARTESIAN_POINT ( 'NONE',  ( -22.64031343690345111, -17.27870339600297811, 56.85231026484398598 ) ) ;
#11929=LINE ( 'NONE', #2447, #7719 ) ;
#11930=( BOUNDED_CURVE ( )  B_SPLINE_CURVE ( 3, ( #2589, #7001, #9396, #14063 ),
 .UNSPECIFIED., .F., .T. ) 
 B_SPLINE_CURVE_WITH_KNOTS ( ( 4, 4 ),
 ( 1.570796326794896114, 3.141592653589792672 ),
 .UNSPECIFIED. ) 
 CURVE ( )  GEOMETRIC_REPRESENTATION_ITEM ( )  RATIONAL_B_SPLINE_CURVE ( ( 1.000000000000000000, 0.8047378541243649375, 0.8047378541243649375, 1.000000000000000000 ) ) 
 REPRESENTATION_ITEM ( '' )  );
#11931=EDGE_CURVE ( 'NONE', #3714, #11739, #13411, .T. ) ;
#11933=VERTEX_POINT ( 'NONE', #8803 ) ;
#11936=CARTESIAN_POINT ( 'NONE',  ( -24.05607732349520234, -14.07716379046991584, 57.00231026484397745 ) ) ;
#11943=ORIENTED_EDGE ( 'NONE', *, *, #7637, .F. ) ;
#11944=CARTESIAN_POINT ( 'NONE',  ( -22.86200450971638531, -18.81376385001357932, 56.85231026484398598 ) ) ;
#11945=ORIENTED_EDGE ( 'NONE', *, *, #13313, .T. ) ;
#11946=VECTOR ( 'NONE', #13492, 1000.000000000000114 ) ;
#11947=LINE ( 'NONE', #12873, #1948 ) ;
#11949=DIRECTION ( 'NONE',  ( -8.018662683283439195E-16, 5.975035461963190001E-16, 1.000000000000000000 ) ) ;
#11952=EDGE_CURVE ( 'NONE', #6007, #11221, #13630, .T. ) ;
#11955=CARTESIAN_POINT ( 'NONE',  ( -15.04562126104788966, -5.444807279564146896, 56.85231026484398598 ) ) ;
#11956=EDGE_CURVE ( 'NONE', #2788, #2864, #7581, .T. ) ;
#11958=ORIENTED_EDGE ( 'NONE', *, *, #3088, .T. ) ;
#11960=VERTEX_POINT ( 'NONE', #7722 ) ;
#11963=ORIENTED_EDGE ( 'NONE', *, *, #13475, .F. ) ;
#11964=CARTESIAN_POINT ( 'NONE',  ( -25.46211945451987191, -14.00819915864900800, 56.85231026484398598 ) ) ;
#11965=DIRECTION ( 'NONE',  ( -8.018662683283438208E-16, 5.975035461963189015E-16, 1.000000000000000000 ) ) ;
#11967=EDGE_CURVE ( 'NONE', #6204, #8466, #628, .T. ) ;
#11969=DIRECTION ( 'NONE',  ( -0.9931883319083343320, 0.1165201156931293391, -8.660254037844387408E-16 ) ) ;
#11970=DIRECTION ( 'NONE',  ( -0.7582332219680868457, 0.6519834208811555731, -9.975640502598242007E-16 ) ) ;
#11971=ADVANCED_FACE ( 'NONE', ( #7950 ), #14924, .F. ) ;
#11974=CARTESIAN_POINT ( 'NONE',  ( -11.16775676328319200, -22.49263881059494707, 57.00231026484399166 ) ) ;
#11975=EDGE_CURVE ( 'NONE', #7684, #2792, #8026, .T. ) ;
#11977=CARTESIAN_POINT ( 'NONE',  ( -15.14850084941412511, -4.438867027711355107, 57.00231026484397745 ) ) ;
#11984=EDGE_CURVE ( 'NONE', #8987, #3406, #11481, .T. ) ;
#11985=AXIS2_PLACEMENT_3D ( 'NONE', #10587, #7127, #14263 ) ;
#11986=FACE_OUTER_BOUND ( 'NONE', #11571, .T. ) ;
#11989=ADVANCED_FACE ( 'NONE', ( #2079 ), #6412, .T. ) ;
#11991=CARTESIAN_POINT ( 'NONE',  ( -19.41680297924232690, -22.68108752059492517, 57.00231026484399166 ) ) ;
#11993=VERTEX_POINT ( 'NONE', #856 ) ;
#11999=ORIENTED_EDGE ( 'NONE', *, *, #9333, .T. ) ;
#12000=DIRECTION ( 'NONE',  ( -8.018662683283438208E-16, 5.975035461963189015E-16, 1.000000000000000000 ) ) ;
#12001=ORIENTED_EDGE ( 'NONE', *, *, #3812, .T. ) ;
#12002=CARTESIAN_POINT ( 'NONE',  ( -9.884208147447518300, -5.263176313152190922, 56.85231026484398598 ) ) ;
#12003=CARTESIAN_POINT ( 'NONE',  ( -6.309378268457435546, -9.629413800598410234, 56.85231026484400019 ) ) ;
#12009=VERTEX_POINT ( 'NONE', #11404 ) ;
#12012=VECTOR ( 'NONE', #9664, 1000.000000000000000 ) ;
#12013=CARTESIAN_POINT ( 'NONE',  ( -23.40321606353253614, -15.16438883951732741, 56.85231026484398598 ) ) ;
#12014=ORIENTED_EDGE ( 'NONE', *, *, #12527, .T. ) ;
#12018=VERTEX_POINT ( 'NONE', #4376 ) ;
#12025=AXIS2_PLACEMENT_3D ( 'NONE', #5398, #5053, #4980 ) ;
#12028=DIRECTION ( 'NONE',  ( -8.018662683283438208E-16, 5.975035461963189015E-16, 1.000000000000000000 ) ) ;
#12031=DIRECTION ( 'NONE',  ( 0.5975035461963189576, 0.8018662683283437342, 0.000000000000000000 ) ) ;
#12034=CARTESIAN_POINT ( 'NONE',  ( -5.650856670168516338, -15.08880645082409622, 54.00231026484399166 ) ) ;
#12036=VERTEX_POINT ( 'NONE', #4447 ) ;
#12037=AXIS2_PLACEMENT_3D ( 'NONE', #10717, #320, #8101 ) ;
#12039=LINE ( 'NONE', #10888, #12769 ) ;
#12040=VERTEX_POINT ( 'NONE', #10407 ) ;
#12042=CARTESIAN_POINT ( 'NONE',  ( -7.654212976755197850, -10.04550297615607768, 56.85231026484400019 ) ) ;
#12043=EDGE_CURVE ( 'NONE', #10505, #11993, #1005, .T. ) ;
#12046=DIRECTION ( 'NONE',  ( 0.1855175943453168941, 0.9826409426582662920, -4.383711467890769768E-16 ) ) ;
#12047=CIRCLE ( 'NONE', #6162, 9.974999999999999645 ) ;
#12050=DIRECTION ( 'NONE',  ( 8.018662683283438208E-16, -5.975035461963189015E-16, -1.000000000000000000 ) ) ;
#12051=CARTESIAN_POINT ( 'NONE',  ( -12.72810521832141362, -22.14910990341453001, 57.00231026484399166 ) ) ;
#12052=ORIENTED_EDGE ( 'NONE', *, *, #2963, .T. ) ;
#12054=EDGE_LOOP ( 'NONE', ( #2473, #8915, #683, #11689 ) ) ;
#12058=LINE ( 'NONE', #7672, #1512 ) ;
#12060=VECTOR ( 'NONE', #1773, 1000.000000000000000 ) ;
#12061=ADVANCED_FACE ( 'NONE', ( #1305 ), #13095, .T. ) ;
#12062=AXIS2_PLACEMENT_3D ( 'NONE', #13663, #5469, #1811 ) ;
#12063=EDGE_CURVE ( 'NONE', #14661, #12770, #10871, .T. ) ;
#12064=ADVANCED_FACE ( 'NONE', ( #9412 ), #2382, .F. ) ;
#12067=EDGE_CURVE ( 'NONE', #1451, #5453, #3904, .T. ) ;
#12071=ORIENTED_EDGE ( 'NONE', *, *, #9266, .F. ) ;
#12072=DIRECTION ( 'NONE',  ( 0.1165201156931293391, 0.9931883319083343320, -4.999999999999998416E-16 ) ) ;
#12082=PLANE ( 'NONE',  #8356 ) ;
#12084=AXIS2_PLACEMENT_3D ( 'NONE', #353, #3783, #4784 ) ;
#12086=CARTESIAN_POINT ( 'NONE',  ( -23.08034316846174150, -10.72437754756471762, 57.00231026484397745 ) ) ;
#12088=CARTESIAN_POINT ( 'NONE',  ( -24.39712111458419130, -18.01698208283363556, 57.00231026484397745 ) ) ;
#12090=AXIS2_PLACEMENT_3D ( 'NONE', #2143, #11321, #10159 ) ;
#12093=ORIENTED_EDGE ( 'NONE', *, *, #6544, .F. ) ;
#12095=ORIENTED_EDGE ( 'NONE', *, *, #6770, .T. ) ;
#12096=EDGE_LOOP ( 'NONE', ( #6915, #1926, #2432, #9106, #3150, #14794, #5125, #6138, #4085, #7072, #1511, #3072, #5705, #4967, #4792, #3681, #7539, #11387, #15091, #4526, #8274, #9871, #8262, #13249, #3063, #10211, #7091, #3997, #1345, #6031, #9162, #9465, #9793, #11687, #12364, #9426, #6956, #6328, #13409, #291, #12739, #5940, #4310, #943, #14940, #8614, #6405, #1889, #4850, #4337, #12482, #956, #8185, #8883, #8933, #11613, #11615, #4617, #2349, #6160, #10042, #14230, #870, #2097, #6202, #13671, #294, #5966, #4468, #6893, #6312, #6671, #13762, #11010, #12818, #5749, #4240, #14961, #502, #14457, #8506, #629, #10074, #9775, #4940, #188, #2895, #13002, #14667, #7926, #9120, #6964 ) ) ;
#12100=VECTOR ( 'NONE', #11791, 1000.000000000000000 ) ;
#12105=LINE ( 'NONE', #5211, #3732 ) ;
#12106=DIRECTION ( 'NONE',  ( -0.5975035461963187355, -0.8018662683283439563, 0.000000000000000000 ) ) ;
#12108=CARTESIAN_POINT ( 'NONE',  ( -15.19690733689918183, -23.47778227853769550, 54.00231026484399166 ) ) ;
#12109=ORIENTED_EDGE ( 'NONE', *, *, #14124, .T. ) ;
#12110=ORIENTED_EDGE ( 'NONE', *, *, #11167, .F. ) ;
#12111=CARTESIAN_POINT ( 'NONE',  ( -17.95685260396766125, -23.17500669507537836, 56.85231026484400019 ) ) ;
#12116=VECTOR ( 'NONE', #2281, 1000.000000000000114 ) ;
#12121=ORIENTED_EDGE ( 'NONE', *, *, #1824, .T. ) ;
#12122=CARTESIAN_POINT ( 'NONE',  ( -12.60362876103445373, -23.05271278361805543, 56.85231026484400019 ) ) ;
#12124=CARTESIAN_POINT ( 'NONE',  ( -21.29301345516119071, -7.881655252552254964, 56.85231026484398598 ) ) ;
#12126=ORIENTED_EDGE ( 'NONE', *, *, #5360, .F. ) ;
#12133=DIRECTION ( 'NONE',  ( -8.018662683283438208E-16, 5.975035461963189015E-16, 1.000000000000000000 ) ) ;
#12134=EDGE_CURVE ( 'NONE', #3679, #1866, #8334, .T. ) ;
#12135=DIRECTION ( 'NONE',  ( 0.3533329742249663452, 0.9354976265738675911, -2.756373558169968730E-16 ) ) ;
#12136=ORIENTED_EDGE ( 'NONE', *, *, #6658, .T. ) ;
#12137=DIRECTION ( 'NONE',  ( -0.9578660637129379207, 0.2872152572324145892, -9.396926207859088029E-16 ) ) ;
#12138=VECTOR ( 'NONE', #3590, 1000.000000000000000 ) ;
#12139=DIRECTION ( 'NONE',  ( 8.018662683283438208E-16, -5.975035461963189015E-16, -1.000000000000000000 ) ) ;
#12140=EDGE_LOOP ( 'NONE', ( #8045, #14781, #8259, #4451 ) ) ;
#12141=EDGE_CURVE ( 'NONE', #221, #11420, #3680, .T. ) ;
#12144=DIRECTION ( 'NONE',  ( -8.018662683283438208E-16, 5.975035461963189015E-16, 1.000000000000000000 ) ) ;
#12145=ORIENTED_EDGE ( 'NONE', *, *, #8493, .F. ) ;
#12149=AXIS2_PLACEMENT_3D ( 'NONE', #7073, #3575, #14365 ) ;
#12153=DIRECTION ( 'NONE',  ( -0.8543800322332368857, -0.5196486895212314439, -3.746065934159101186E-16 ) ) ;
#12154=VERTEX_POINT ( 'NONE', #10790 ) ;
#12158=EDGE_CURVE ( 'NONE', #8821, #11659, #2529, .T. ) ;
#12159=ORIENTED_EDGE ( 'NONE', *, *, #3571, .F. ) ;
#12161=CIRCLE ( 'NONE', #7754, 4.999999999999999112 ) ;
#12165=EDGE_LOOP ( 'NONE', ( #4643, #10979, #11901, #9190 ) ) ;
#12168=CARTESIAN_POINT ( 'NONE',  ( -15.53979317422733786, -13.47750381512840967, 56.85231026484398598 ) ) ;
#12171=DIRECTION ( 'NONE',  ( -0.7032868978765923762, -0.7109061395677488404, -1.391731009600549731E-16 ) ) ;
#12172=CARTESIAN_POINT ( 'NONE',  ( -15.50552586659557797, -13.55703840903364288, 56.85231026484398598 ) ) ;
#12174=EDGE_CURVE ( 'NONE', #2842, #2678, #1476, .T. ) ;
#12177=ORIENTED_EDGE ( 'NONE', *, *, #7, .T. ) ;
#12178=EDGE_CURVE ( 'NONE', #11708, #4294, #4127, .T. ) ;
#12181=LINE ( 'NONE', #14551, #10728 ) ;
#12183=ORIENTED_EDGE ( 'NONE', *, *, #3359, .T. ) ;
#12184=CIRCLE ( 'NONE', #8015, 9.974999999999999645 ) ;
#12187=DIRECTION ( 'NONE',  ( 8.018662683283438208E-16, -5.975035461963189015E-16, -1.000000000000000000 ) ) ;
#12190=DIRECTION ( 'NONE',  ( 8.018662683283438208E-16, -5.975035461963189015E-16, -1.000000000000000000 ) ) ;
#12192=CIRCLE ( 'NONE', #5582, 9.974999999999999645 ) ;
#12196=ORIENTED_EDGE ( 'NONE', *, *, #1118, .F. ) ;
#12198=EDGE_LOOP ( 'NONE', ( #4603, #13000, #3464, #13876 ) ) ;
#12200=ORIENTED_EDGE ( 'NONE', *, *, #14035, .F. ) ;
#12204=EDGE_LOOP ( 'NONE', ( #10917, #5345, #7045, #7741 ) ) ;
#12209=FACE_OUTER_BOUND ( 'NONE', #1098, .T. ) ;
#12210=CARTESIAN_POINT ( 'NONE',  ( -15.24029490235350259, -21.57855976525750563, 57.00231026484399166 ) ) ;
#12215=DIRECTION ( 'NONE',  ( 0.1165201156931293391, 0.9931883319083343320, -4.999999999999998416E-16 ) ) ;
#12216=ADVANCED_FACE ( 'NONE', ( #7559 ), #3049, .F. ) ;
#12217=LINE ( 'NONE', #5254, #10722 ) ;
#12218=ORIENTED_EDGE ( 'NONE', *, *, #12158, .T. ) ;
#12219=AXIS2_PLACEMENT_3D ( 'NONE', #14878, #4400, #4475 ) ;
#12221=CARTESIAN_POINT ( 'NONE',  ( -14.60940909295887913, -15.57374835648654532, 51.00231026484399166 ) ) ;
#12222=ORIENTED_EDGE ( 'NONE', *, *, #2479, .T. ) ;
#12232=DIRECTION ( 'NONE',  ( -8.018662683283438208E-16, 5.975035461963189015E-16, 1.000000000000000000 ) ) ;
#12243=FACE_OUTER_BOUND ( 'NONE', #14179, .T. ) ;
#12244=EDGE_CURVE ( 'NONE', #3602, #6022, #11240, .T. ) ;
#12245=DIRECTION ( 'NONE',  ( 8.018662683283438208E-16, -5.975035461963189015E-16, -1.000000000000000000 ) ) ;
#12247=DIRECTION ( 'NONE',  ( -8.018662683283438208E-16, 5.975035461963189015E-16, 1.000000000000000000 ) ) ;
#12250=DIRECTION ( 'NONE',  ( 0.8018662683283436232, -0.5975035461963189576, 9.999999999999998805E-16 ) ) ;
#12251=VECTOR ( 'NONE', #7517, 1000.000000000000000 ) ;
#12253=EDGE_CURVE ( 'NONE', #8358, #8353, #4021, .T. ) ;
#12254=CARTESIAN_POINT ( 'NONE',  ( -15.86970092169881141, -16.66117552174622318, 57.00231026484397745 ) ) ;
#12255=CARTESIAN_POINT ( 'NONE',  ( -12.98295438134161195, -5.834228258119843247, 56.85231026484398598 ) ) ;
#12259=VERTEX_POINT ( 'NONE', #12466 ) ;
#12263=ORIENTED_EDGE ( 'NONE', *, *, #9386, .F. ) ;
#12264=VECTOR ( 'NONE', #5959, 1000.000000000000114 ) ;
#12267=CARTESIAN_POINT ( 'NONE',  ( -14.07534335717186202, -5.558639560896826204, 57.00231026484397745 ) ) ;
#12268=LINE ( 'NONE', #1706, #9975 ) ;
#12269=VECTOR ( 'NONE', #9358, 999.9999999999998863 ) ;
#12272=FACE_OUTER_BOUND ( 'NONE', #2326, .T. ) ;
#12273=DIRECTION ( 'NONE',  ( -8.018662683283438208E-16, 5.975035461963189015E-16, 1.000000000000000000 ) ) ;
#12276=ORIENTED_EDGE ( 'NONE', *, *, #10140, .T. ) ;
#12277=DIRECTION ( 'NONE',  ( -8.018662683283438208E-16, 5.975035461963189015E-16, 1.000000000000000000 ) ) ;
#12285=VECTOR ( 'NONE', #6933, 1000.000000000000000 ) ;
#12286=VECTOR ( 'NONE', #8797, 1000.000000000000114 ) ;
#12288=CARTESIAN_POINT ( 'NONE',  ( -22.00391959472895209, -7.178368354675633611, 56.85231026484398598 ) ) ;
#12290=LINE ( 'NONE', #1810, #13536 ) ;
#12291=DIRECTION ( 'NONE',  ( -0.9931883319083342210, 0.1165201156931306992, 0.000000000000000000 ) ) ;
#12295=VERTEX_POINT ( 'NONE', #3203 ) ;
#12297=AXIS2_PLACEMENT_3D ( 'NONE', #8727, #10961, #7650 ) ;
#12298=DIRECTION ( 'NONE',  ( 0.5975035461963187355, 0.8018662683283439563, 0.000000000000000000 ) ) ;
#12299=DIRECTION ( 'NONE',  ( -0.7582332219680880669, 0.6519834208811540188, -9.975640502598240034E-16 ) ) ;
#12301=DIRECTION ( 'NONE',  ( 0.5975035461963189576, 0.8018662683283437342, 0.000000000000000000 ) ) ;
#12303=CIRCLE ( 'NONE', #8873, 9.974999999999999645 ) ;
#12305=CIRCLE ( 'NONE', #822, 9.974999999999999645 ) ;
#12306=DIRECTION ( 'NONE',  ( 0.5975035461963187355, 0.8018662683283439563, 0.000000000000000000 ) ) ;
#12308=ORIENTED_EDGE ( 'NONE', *, *, #1501, .F. ) ;
#12310=DIRECTION ( 'NONE',  ( 8.018662683283438208E-16, -5.975035461963189015E-16, -1.000000000000000000 ) ) ;
#12312=ORIENTED_EDGE ( 'NONE', *, *, #2986, .T. ) ;
#12317=LINE ( 'NONE', #14911, #1525 ) ;
#12324=CARTESIAN_POINT ( 'NONE',  ( -16.24959055444668365, -20.54292544936667397, 56.85231026484400019 ) ) ;
#12327=DIRECTION ( 'NONE',  ( -0.9183863840214729901, -0.3956847857120157075, -4.999999999999999402E-16 ) ) ;
#12328=EDGE_CURVE ( 'NONE', #13264, #5925, #10151, .T. ) ;
#12330=EDGE_LOOP ( 'NONE', ( #10694, #9291, #14027, #4039 ) ) ;
#12331=DIRECTION ( 'NONE',  ( 0.7109061395677416240, -0.7032868978765995926, 9.902680687415702019E-16 ) ) ;
#12336=CARTESIAN_POINT ( 'NONE',  ( -6.517576446443361426, -14.80457171870128974, 56.85231026484400019 ) ) ;
#12338=ORIENTED_EDGE ( 'NONE', *, *, #3387, .F. ) ;
#12339=CARTESIAN_POINT ( 'NONE',  ( -22.53804163936502647, -6.438972523632135569, 57.00231026484397745 ) ) ;
#12341=ADVANCED_FACE ( 'NONE', ( #14982 ), #13761, .T. ) ;
#12346=EDGE_CURVE ( 'NONE', #4983, #5733, #4507, .T. ) ;
#12348=CARTESIAN_POINT ( 'NONE',  ( -13.02562488396841900, -21.19439421350821817, 56.85231026484400019 ) ) ;
#12349=ADVANCED_FACE ( 'NONE', ( #9235 ), #13838, .F. ) ;
#12351=CARTESIAN_POINT ( 'NONE',  ( -7.821737630532772378, -18.34578224045527151, 56.85231026484400019 ) ) ;
#12354=ADVANCED_FACE ( 'NONE', ( #15057 ), #149, .F. ) ;
#12357=CARTESIAN_POINT ( 'NONE',  ( -23.43263029221230198, -15.01730109988151440, 56.85231026484398598 ) ) ;
#12360=VECTOR ( 'NONE', #141, 1000.000000000000000 ) ;
#12361=DIRECTION ( 'NONE',  ( -8.018662683283438208E-16, 5.975035461963189015E-16, 1.000000000000000000 ) ) ;
#12363=CYLINDRICAL_SURFACE ( 'NONE', #9820, 0.2499999999999997502 ) ;
#12364=ORIENTED_EDGE ( 'NONE', *, *, #4767, .F. ) ;
#12367=DIRECTION ( 'NONE',  ( 8.018662683283438208E-16, -5.975035461963189015E-16, -1.000000000000000000 ) ) ;
#12368=ORIENTED_EDGE ( 'NONE', *, *, #5160, .T. ) ;
#12372=VECTOR ( 'NONE', #9169, 1000.000000000000000 ) ;
#12373=CARTESIAN_POINT ( 'NONE',  ( -23.96284084890188382, -10.23071992935364527, 56.85231026484398598 ) ) ;
#12375=DIRECTION ( 'NONE',  ( 0.5975035461963188466, 0.8018662683283437342, 0.000000000000000000 ) ) ;
#12378=CARTESIAN_POINT ( 'NONE',  ( -15.39025577592761174, -21.58198560776530783, 57.00231026484399166 ) ) ;
#12379=VECTOR ( 'NONE', #13549, 1000.000000000000000 ) ;
#12385=AXIS2_PLACEMENT_3D ( 'NONE', #12813, #10273, #14939 ) ;
#12387=CARTESIAN_POINT ( 'NONE',  ( -18.86735971344653962, -5.080035572537331845, 56.85231026484398598 ) ) ;
#12389=ORIENTED_EDGE ( 'NONE', *, *, #5260, .T. ) ;
#12390=DIRECTION ( 'NONE',  ( -8.018662683283438208E-16, 5.975035461963189015E-16, 1.000000000000000000 ) ) ;
#12391=VECTOR ( 'NONE', #5556, 1000.000000000000114 ) ;
#12393=DIRECTION ( 'NONE',  ( 0.5975035461963188466, 0.8018662683283437342, 0.000000000000000000 ) ) ;
#12394=CIRCLE ( 'NONE', #3605, 9.974999999999999645 ) ;
#12398=CARTESIAN_POINT ( 'NONE',  ( -17.88573767796789582, -14.53539822139104842, 51.00231026484399166 ) ) ;
#12400=DIRECTION ( 'NONE',  ( 0.5975035461963189576, 0.8018662683283437342, 0.000000000000000000 ) ) ;
#12401=CARTESIAN_POINT ( 'NONE',  ( -15.84999713957374645, -16.49322540957318495, 57.00231026484398456 ) ) ;
#12403=ORIENTED_EDGE ( 'NONE', *, *, #9064, .F. ) ;
#12406=CARTESIAN_POINT ( 'NONE',  ( -7.425287632467987287, -13.60480674405941492, 57.00231026484399166 ) ) ;
#12408=EDGE_LOOP ( 'NONE', ( #9527, #536, #12689, #11373 ) ) ;
#12415=EDGE_CURVE ( 'NONE', #2536, #4202, #12930, .T. ) ;
#12419=DIRECTION ( 'NONE',  ( 0.000000000000000000, 0.000000000000000000, 1.000000000000000000 ) ) ;
#12420=EDGE_CURVE ( 'NONE', #413, #9544, #8379, .T. ) ;
#12421=CARTESIAN_POINT ( 'NONE',  ( -16.17213342976032209, -5.460076146431361188, 56.85231026484398598 ) ) ;
#12422=DIRECTION ( 'NONE',  ( -0.8018662683283437342, 0.5975035461963188466, -1.000000000000000078E-15 ) ) ;
#12423=EDGE_LOOP ( 'NONE', ( #527, #9502, #11879, #4697 ) ) ;
#12425=EDGE_LOOP ( 'NONE', ( #1532, #4866, #4394, #10257 ) ) ;
#12426=CARTESIAN_POINT ( 'NONE',  ( -22.61924992783766797, -9.696439889920343447, 56.85231026484398598 ) ) ;
#12427=VERTEX_POINT ( 'NONE', #13157 ) ;
#12429=CARTESIAN_POINT ( 'NONE',  ( -24.41321522311770664, -15.21339595774672127, 57.00231026484397745 ) ) ;
#12430=VERTEX_POINT ( 'NONE', #5941 ) ;
#12434=LINE ( 'NONE', #12288, #8773 ) ;
#12435=EDGE_CURVE ( 'NONE', #15030, #14193, #1363, .T. ) ;
#12436=LINE ( 'NONE', #3096, #8982 ) ;
#12437=ADVANCED_FACE ( 'NONE', ( #4875 ), #4657, .F. ) ;
#12441=ORIENTED_EDGE ( 'NONE', *, *, #6004, .T. ) ;
#12442=CARTESIAN_POINT ( 'NONE',  ( -9.002116193859002635, -10.70790913352571927, 56.85231026484400019 ) ) ;
#12443=VECTOR ( 'NONE', #2698, 999.9999999999998863 ) ;
#12444=CARTESIAN_POINT ( 'NONE',  ( -8.430459378593662123, -7.816413432484393020, 56.85231026484400019 ) ) ;
#12446=ADVANCED_FACE ( 'NONE', ( #14142 ), #10619, .T. ) ;
#12447=CARTESIAN_POINT ( 'NONE',  ( -15.49969986081092088, -13.50737899243822504, 57.00231026484397745 ) ) ;
#12448=LINE ( 'NONE', #9790, #7377 ) ;
#12449=DIRECTION ( 'NONE',  ( -8.018662683283438208E-16, 5.975035461963189015E-16, 1.000000000000000000 ) ) ;
#12450=FACE_OUTER_BOUND ( 'NONE', #14586, .T. ) ;
#12451=ORIENTED_EDGE ( 'NONE', *, *, #4682, .T. ) ;
#12452=CARTESIAN_POINT ( 'NONE',  ( -15.34686821047329808, -23.48120812104550481, 54.00231026484399166 ) ) ;
#12454=CARTESIAN_POINT ( 'NONE',  ( -22.86200450971638531, -18.81376385001357932, 56.85231026484398598 ) ) ;
#12466=CARTESIAN_POINT ( 'NONE',  ( -7.016473591028808521, -8.259951331604913349, 57.00231026484399166 ) ) ;
#12469=EDGE_CURVE ( 'NONE', #2788, #4722, #11930, .T. ) ;
#12471=DIRECTION ( 'NONE',  ( 0.7350174335289111349, -0.6780482080269607525, 9.945218953682729003E-16 ) ) ;
#12473=LINE ( 'NONE', #6482, #14715 ) ;
#12474=LINE ( 'NONE', #995, #4027 ) ;
#12476=CARTESIAN_POINT ( 'NONE',  ( -12.51218212982932165, -9.498047650796509700, 51.00231026484399166 ) ) ;
#12477=CARTESIAN_POINT ( 'NONE',  ( -17.20133171717847631, -6.639650181150215325, 56.85231026484398598 ) ) ;
#12478=LINE ( 'NONE', #14692, #5480 ) ;
#12479=CARTESIAN_POINT ( 'NONE',  ( -13.96026682931439211, -23.36287344688023992, 56.85231026484400019 ) ) ;
#12482=ORIENTED_EDGE ( 'NONE', *, *, #1754, .F. ) ;
#12483=CARTESIAN_POINT ( 'NONE',  ( -24.55043086433169819, -12.83990741858047357, 57.00231026484397745 ) ) ;
#12486=VERTEX_POINT ( 'NONE', #3581 ) ;
#12487=EDGE_CURVE ( 'NONE', #5474, #4089, #12303, .T. ) ;
#12488=DIRECTION ( 'NONE',  ( -8.018662683283438208E-16, 5.975035461963189015E-16, 1.000000000000000000 ) ) ;
#12489=ORIENTED_EDGE ( 'NONE', *, *, #10616, .T. ) ;
#12491=DIRECTION ( 'NONE',  ( 0.5975035461963187355, 0.8018662683283439563, 0.000000000000000000 ) ) ;
#12492=CARTESIAN_POINT ( 'NONE',  ( -10.16926643994361967, -19.57302854922115287, 56.85231026484400019 ) ) ;
#12496=ORIENTED_EDGE ( 'NONE', *, *, #4578, .F. ) ;
#12500=EDGE_CURVE ( 'NONE', #3416, #2925, #298, .T. ) ;
#12503=DIRECTION ( 'NONE',  ( -0.9997391571607664451, -0.02283895005205794498, -7.880107536067222722E-16 ) ) ;
#12504=FACE_BOUND ( 'NONE', #3505, .T. ) ;
#12505=VECTOR ( 'NONE', #5458, 1000.000000000000227 ) ;
#12507=VECTOR ( 'NONE', #9189, 1000.000000000000227 ) ;
#12518=EDGE_CURVE ( 'NONE', #626, #8256, #6389, .T. ) ;
#12519=VECTOR ( 'NONE', #11071, 999.9999999999998863 ) ;
#12521=VECTOR ( 'NONE', #2832, 1000.000000000000114 ) ;
#12527=EDGE_CURVE ( 'NONE', #3602, #11369, #13299, .T. ) ;
#12528=DIRECTION ( 'NONE',  ( 0.6061090314442014737, -0.7953815700667020705, 9.612616959383187437E-16 ) ) ;
#12529=EDGE_CURVE ( 'NONE', #14910, #951, #382, .T. ) ;
#12532=VECTOR ( 'NONE', #11965, 1000.000000000000000 ) ;
#12533=VECTOR ( 'NONE', #10093, 1000.000000000000114 ) ;
#12536=VERTEX_POINT ( 'NONE', #664 ) ;
#12538=ADVANCED_FACE ( 'NONE', ( #1663 ), #6463, .F. ) ;
#12540=CARTESIAN_POINT ( 'NONE',  ( -21.89842656004739396, -7.071732433740530510, 56.85231026484398598 ) ) ;
#12541=ADVANCED_FACE ( 'NONE', ( #6316 ), #1588, .T. ) ;
#12550=AXIS2_PLACEMENT_3D ( 'NONE', #3409, #8059, #11662 ) ;
#12551=AXIS2_PLACEMENT_3D ( 'NONE', #3595, #8176, #4978 ) ;
#12552=PLANE ( 'NONE',  #5668 ) ;
#12553=VECTOR ( 'NONE', #12922, 999.9999999999998863 ) ;
#12556=DIRECTION ( 'NONE',  ( -0.9085715390340278752, 0.4177292884839868825, -9.781476007338035090E-16 ) ) ;
#12557=VECTOR ( 'NONE', #12000, 1000.000000000000000 ) ;
#12558=DIRECTION ( 'NONE',  ( 0.9183863840214729901, 0.3956847857120157075, 4.999999999999999402E-16 ) ) ;
#12561=EDGE_CURVE ( 'NONE', #1793, #13470, #7395, .T. ) ;
#12562=ORIENTED_EDGE ( 'NONE', *, *, #7865, .T. ) ;
#12565=ORIENTED_EDGE ( 'NONE', *, *, #918, .T. ) ;
#12566=VERTEX_POINT ( 'NONE', #3033 ) ;
#12576=DIRECTION ( 'NONE',  ( 8.018662683283438208E-16, -5.975035461963189015E-16, -1.000000000000000000 ) ) ;
#12578=CARTESIAN_POINT ( 'NONE',  ( -8.131654986474892155, -16.81240013151894530, 56.85231026484400019 ) ) ;
#12581=ORIENTED_EDGE ( 'NONE', *, *, #7673, .T. ) ;
#12583=EDGE_LOOP ( 'NONE', ( #8903, #10062, #5831, #8859 ) ) ;
#12584=EDGE_LOOP ( 'NONE', ( #6706, #2758, #4558, #817 ) ) ;
#12586=PLANE ( 'NONE',  #10045 ) ;
#12588=LINE ( 'NONE', #2101, #13996 ) ;
#12589=DIRECTION ( 'NONE',  ( 0.1960948578651655061, -0.9805849309054471830, 7.431448254773943634E-16 ) ) ;
#12592=ADVANCED_FACE ( 'NONE', ( #7469 ), #595, .F. ) ;
#12593=CARTESIAN_POINT ( 'NONE',  ( -12.51218212982931810, -9.498047650796513253, 45.50231026484398456 ) ) ;
#12595=LINE ( 'NONE', #5692, #14478 ) ;
#12598=DIRECTION ( 'NONE',  ( -0.7276687409742212953, -0.6859287159822015090, -1.736481776669299976E-16 ) ) ;
#12600=VERTEX_POINT ( 'NONE', #7543 ) ;
#12601=EDGE_LOOP ( 'NONE', ( #4018, #7598, #8900, #3770 ) ) ;
#12602=CARTESIAN_POINT ( 'NONE',  ( -15.86970092169881141, -16.66117552174622318, 57.00231026484397745 ) ) ;
#12610=LINE ( 'NONE', #3421, #4797 ) ;
#12611=CARTESIAN_POINT ( 'NONE',  ( -12.52039621090187893, -4.935039769003430443, 56.85231026484398598 ) ) ;
#12612=EDGE_CURVE ( 'NONE', #10845, #6478, #14588, .T. ) ;
#12614=VERTEX_POINT ( 'NONE', #13452 ) ;
#12616=CIRCLE ( 'NONE', #6002, 9.974999999999999645 ) ;
#12618=DIRECTION ( 'NONE',  ( 0.5975035461963188466, 0.8018662683283437342, 0.000000000000000000 ) ) ;
#12619=DIRECTION ( 'NONE',  ( 0.5975035461963188466, 0.8018662683283437342, 0.000000000000000000 ) ) ;
#12620=ORIENTED_EDGE ( 'NONE', *, *, #3346, .T. ) ;
#12625=EDGE_CURVE ( 'NONE', #3870, #1460, #2957, .T. ) ;
#12626=LINE ( 'NONE', #2142, #9584 ) ;
#12628=EDGE_CURVE ( 'NONE', #6762, #11659, #519, .T. ) ;
#12632=FACE_OUTER_BOUND ( 'NONE', #11598, .T. ) ;
#12633=CARTESIAN_POINT ( 'NONE',  ( -15.49969986081092088, -13.50737899243822504, 56.85231026484398598 ) ) ;
#12635=DIRECTION ( 'NONE',  ( -8.018662683283438208E-16, 5.975035461963189015E-16, 1.000000000000000000 ) ) ;
#12638=DIRECTION ( 'NONE',  ( -0.5491495666976170531, 0.8357240892757724637, -9.396926207859082113E-16 ) ) ;
#12640=EDGE_LOOP ( 'NONE', ( #10006, #2015, #15004, #4459 ) ) ;
#12641=EDGE_CURVE ( 'NONE', #9932, #2536, #744, .T. ) ;
#12643=CARTESIAN_POINT ( 'NONE',  ( -12.95343247850694723, -15.40470757524832912, 57.00231026484399166 ) ) ;
#12652=CIRCLE ( 'NONE', #4843, 9.974999999999999645 ) ;
#12653=EDGE_CURVE ( 'NONE', #1455, #13413, #10219, .T. ) ;
#12654=ORIENTED_EDGE ( 'NONE', *, *, #8050, .T. ) ;
#12655=LINE ( 'NONE', #5748, #14485 ) ;
#12662=VECTOR ( 'NONE', #11045, 1000.000000000000000 ) ;
#12663=LINE ( 'NONE', #8127, #14484 ) ;
#12664=EDGE_CURVE ( 'NONE', #5453, #2941, #3190, .T. ) ;
#12666=CARTESIAN_POINT ( 'NONE',  ( -15.49969986081092088, -13.50737899243822504, 56.85231026484398598 ) ) ;
#12672=DIRECTION ( 'NONE',  ( 8.018662683283438208E-16, -5.975035461963189015E-16, -1.000000000000000000 ) ) ;
#12673=PLANE ( 'NONE',  #3268 ) ;
#12674=EDGE_LOOP ( 'NONE', ( #10146, #12109, #8411, #1421 ) ) ;
#12675=ORIENTED_EDGE ( 'NONE', *, *, #9986, .T. ) ;
#12678=DIRECTION ( 'NONE',  ( 0.6859287159822015090, -0.7276687409742212953, 9.848077530122081084E-16 ) ) ;
#12679=ORIENTED_EDGE ( 'NONE', *, *, #10855, .F. ) ;
#12680=LINE ( 'NONE', #7990, #1738 ) ;
#12684=PLANE ( 'NONE',  #10945 ) ;
#12687=DIRECTION ( 'NONE',  ( -0.7805252200231699300, 0.6251242923673516749, -9.993908270190957033E-16 ) ) ;
#12688=CARTESIAN_POINT ( 'NONE',  ( -15.39025577592761174, -21.58198560776530783, 56.85231026484400019 ) ) ;
#12689=ORIENTED_EDGE ( 'NONE', *, *, #1065, .T. ) ;
#12692=DIRECTION ( 'NONE',  ( 0.8719950447285833572, 0.4895147004624025300, 4.067366430758019417E-16 ) ) ;
#12694=ORIENTED_EDGE ( 'NONE', *, *, #10908, .T. ) ;
#12695=CARTESIAN_POINT ( 'NONE',  ( -15.14940258204810242, -10.52153257530326158, 57.00231026484397745 ) ) ;
#12699=LINE ( 'NONE', #13616, #7759 ) ;
#12701=VECTOR ( 'NONE', #11603, 1000.000000000000000 ) ;
#12704=LINE ( 'NONE', #9241, #8420 ) ;
#12709=VECTOR ( 'NONE', #9200, 1000.000000000000114 ) ;
#12710=DIRECTION ( 'NONE',  ( 0.5975035461963189576, 0.8018662683283437342, 0.000000000000000000 ) ) ;
#12712=CARTESIAN_POINT ( 'NONE',  ( -22.70654572567255158, -20.40389968624656802, 54.00231026484399166 ) ) ;
#12716=ORIENTED_EDGE ( 'NONE', *, *, #4755, .F. ) ;
#12717=EDGE_CURVE ( 'NONE', #8073, #7447, #6689, .T. ) ;
#12723=ADVANCED_FACE ( 'NONE', ( #12450 ), #13821, .T. ) ;
#12725=CARTESIAN_POINT ( 'NONE',  ( -12.11547932532413263, -20.83938426843124603, 56.85231026484400019 ) ) ;
#12726=EDGE_CURVE ( 'NONE', #15030, #2398, #7988, .T. ) ;
#12729=CARTESIAN_POINT ( 'NONE',  ( -6.938526287600617515, -8.388108336439909607, 56.85231026484400019 ) ) ;
#12730=EDGE_LOOP ( 'NONE', ( #5077, #13113, #13871, #14928 ) ) ;
#12736=ADVANCED_FACE ( 'NONE', ( #2195 ), #6841, .F. ) ;
#12738=EDGE_CURVE ( 'NONE', #12036, #1378, #1968, .T. ) ;
#12739=ORIENTED_EDGE ( 'NONE', *, *, #3176, .F. ) ;
#12740=DIRECTION ( 'NONE',  ( -8.018662683283438208E-16, 5.975035461963189015E-16, 1.000000000000000000 ) ) ;
#12741=DIRECTION ( 'NONE',  ( -8.018662683283439195E-16, 5.975035461963190001E-16, 1.000000000000000000 ) ) ;
#12743=VECTOR ( 'NONE', #10063, 1000.000000000000000 ) ;
#12744=EDGE_CURVE ( 'NONE', #12430, #11072, #5572, .T. ) ;
#12745=CARTESIAN_POINT ( 'NONE',  ( -16.24959055444668365, -20.54292544936667042, 57.00231026484399166 ) ) ;
#12746=DIRECTION ( 'NONE',  ( 0.7737441449604661736, 0.6334982226805353500, 2.419218955996689845E-16 ) ) ;
#12750=CARTESIAN_POINT ( 'NONE',  ( -22.94870171817393256, -18.69135635822624053, 57.00231026484397745 ) ) ;
#12752=ORIENTED_EDGE ( 'NONE', *, *, #14236, .F. ) ;
#12757=CARTESIAN_POINT ( 'NONE',  ( -21.48581293389291247, -5.528213918555015205, 56.85231026484398598 ) ) ;
#12760=AXIS2_PLACEMENT_3D ( 'NONE', #15070, #4829, #9251 ) ;
#12763=CARTESIAN_POINT ( 'NONE',  ( -9.969334273478565933, -7.622966832294271633, 56.85231026484398598 ) ) ;
#12765=ADVANCED_FACE ( 'NONE', ( #3644 ), #9528, .F. ) ;
#12766=EDGE_CURVE ( 'NONE', #1165, #13612, #14050, .T. ) ;
#12769=VECTOR ( 'NONE', #9739, 1000.000000000000000 ) ;
#12770=VERTEX_POINT ( 'NONE', #4946 ) ;
#12772=VECTOR ( 'NONE', #7416, 1000.000000000000114 ) ;
#12774=DIRECTION ( 'NONE',  ( -8.018662683283439195E-16, 5.975035461963190001E-16, 1.000000000000000000 ) ) ;
#12777=DIRECTION ( 'NONE',  ( -8.018662683283438208E-16, 5.975035461963189015E-16, 1.000000000000000000 ) ) ;
#12778=ORIENTED_EDGE ( 'NONE', *, *, #11769, .T. ) ;
#12780=VERTEX_POINT ( 'NONE', #7220 ) ;
#12781=DIRECTION ( 'NONE',  ( -8.018662683283439195E-16, 5.975035461963190001E-16, 1.000000000000000000 ) ) ;
#12782=CARTESIAN_POINT ( 'NONE',  ( -11.71495923925436955, -5.812446346369147143, 56.85231026484398598 ) ) ;
#12784=DIRECTION ( 'NONE',  ( 0.9957106782009863544, 0.09252159378508258147, 7.431448254773871651E-16 ) ) ;
#12785=VECTOR ( 'NONE', #11053, 1000.000000000000114 ) ;
#12786=AXIS2_PLACEMENT_3D ( 'NONE', #8650, #13336, #2839 ) ;
#12789=CARTESIAN_POINT ( 'NONE',  ( -15.49969986081092088, -13.50737899243822504, 56.85231026484398598 ) ) ;
#12792=ORIENTED_EDGE ( 'NONE', *, *, #7076, .F. ) ;
#12793=CARTESIAN_POINT ( 'NONE',  ( -15.47224238247604511, -13.54916519690201149, 56.85231026484398598 ) ) ;
#12794=PRODUCT_DEFINITION_CONTEXT ( 'detailed design', #1660, 'design' ) ;
#12795=VERTEX_POINT ( 'NONE', #1114 ) ;
#12796=LINE ( 'NONE', #11626, #11888 ) ;
#12800=AXIS2_PLACEMENT_3D ( 'NONE', #14076, #10786, #4827 ) ;
#12803=ORIENTED_EDGE ( 'NONE', *, *, #482, .T. ) ;
#12804=LINE ( 'NONE', #8342, #14052 ) ;
#12805=LINE ( 'NONE', #7191, #14672 ) ;
#12808=LINE ( 'NONE', #12578, #9349 ) ;
#12810=VERTEX_POINT ( 'NONE', #9380 ) ;
#12813=CARTESIAN_POINT ( 'NONE',  ( -7.285742840713465007, -17.36641515085804599, 56.85231026484400019 ) ) ;
#12818=ORIENTED_EDGE ( 'NONE', *, *, #10701, .F. ) ;
#12820=VECTOR ( 'NONE', #3415, 1000.000000000000114 ) ;
#12822=DIRECTION ( 'NONE',  ( 8.018662683283438208E-16, -5.975035461963189015E-16, -1.000000000000000000 ) ) ;
#12823=EDGE_CURVE ( 'NONE', #13829, #9275, #6431, .T. ) ;
#12824=EDGE_CURVE ( 'NONE', #745, #12770, #1074, .T. ) ;
#12826=DIRECTION ( 'NONE',  ( -0.5196486895212294455, 0.8543800322332379960, -9.271838545667872786E-16 ) ) ;
#12827=CARTESIAN_POINT ( 'NONE',  ( -12.66248504435161948, -4.886969368454929352, 57.00231026484397745 ) ) ;
#12832=ORIENTED_EDGE ( 'NONE', *, *, #9123, .F. ) ;
#12833=VERTEX_POINT ( 'NONE', #7302 ) ;
#12834=LINE ( 'NONE', #1190, #8355 ) ;
#12836=EDGE_LOOP ( 'NONE', ( #11669, #14921, #9912, #9884 ) ) ;
#12842=DIRECTION ( 'NONE',  ( 0.1272150336605082366, -0.9918751611018171710, 6.946583704589972670E-16 ) ) ;
#12845=LINE ( 'NONE', #11679, #11586 ) ;
#12846=EDGE_CURVE ( 'NONE', #3186, #6946, #11187, .T. ) ;
#12849=DIRECTION ( 'NONE',  ( -0.9183863840214729901, -0.3956847857120157075, -4.999999999999999402E-16 ) ) ;
#12851=DIRECTION ( 'NONE',  ( -0.5975035461963188466, -0.8018662683283437342, 0.000000000000000000 ) ) ;
#12854=ORIENTED_EDGE ( 'NONE', *, *, #503, .F. ) ;
#12855=DIRECTION ( 'NONE',  ( -0.1511109077013120527, -0.9885168150181793401, 4.694715627858928842E-16 ) ) ;
#12858=DIRECTION ( 'NONE',  ( -0.6780482080269578660, -0.7350174335289137995, -1.045284632676540194E-16 ) ) ;
#12859=AXIS2_PLACEMENT_3D ( 'NONE', #7696, #1742, #8926 ) ;
#12863=LINE ( 'NONE', #7018, #4972 ) ;
#12865=DIRECTION ( 'NONE',  ( 0.7511640317997426708, 0.6601155939154560448, 2.079116908177589032E-16 ) ) ;
#12867=DIRECTION ( 'NONE',  ( 0.5975035461963188466, 0.8018662683283437342, 0.000000000000000000 ) ) ;
#12868=ORIENTED_EDGE ( 'NONE', *, *, #10459, .T. ) ;
#12869=ORIENTED_EDGE ( 'NONE', *, *, #13659, .T. ) ;
#12871=ORIENTED_EDGE ( 'NONE', *, *, #3136, .T. ) ;
#12872=AXIS2_PLACEMENT_3D ( 'NONE', #5871, #4591, #8173 ) ;
#12873=CARTESIAN_POINT ( 'NONE',  ( -16.39856880423293006, -20.52544743201270450, 56.85231026484400019 ) ) ;
#12874=EDGE_CURVE ( 'NONE', #3314, #13132, #6146, .T. ) ;
#12875=DIRECTION ( 'NONE',  ( -8.018662683283439195E-16, 5.975035461963190001E-16, 1.000000000000000000 ) ) ;
#12876=DIRECTION ( 'NONE',  ( 0.9085715390340232123, -0.4177292884839972631, 9.781476007338056784E-16 ) ) ;
#12885=AXIS2_PLACEMENT_3D ( 'NONE', #9025, #13704, #3221 ) ;
#12889=AXIS2_PLACEMENT_3D ( 'NONE', #13226, #7462, #10991 ) ;
#12890=CARTESIAN_POINT ( 'NONE',  ( -16.42437072798637843, -22.03270794722917714, 56.85231026484400019 ) ) ;
#12891=EDGE_CURVE ( 'NONE', #9717, #14495, #7656, .T. ) ;
#12893=EDGE_CURVE ( 'NONE', #5733, #8005, #3000, .T. ) ;
#12894=LINE ( 'NONE', #1408, #3423 ) ;
#12895=CARTESIAN_POINT ( 'NONE',  ( -15.49969986081092088, -13.50737899243822504, 56.85231026484398598 ) ) ;
#12897=DIRECTION ( 'NONE',  ( 0.6601155939154559338, -0.7511640317997426708, 9.781476007338054812E-16 ) ) ;
#12900=ORIENTED_EDGE ( 'NONE', *, *, #11882, .F. ) ;
#12901=CARTESIAN_POINT ( 'NONE',  ( -17.72286745096104355, -3.783277446994210536, 56.85231026484398598 ) ) ;
#12903=VECTOR ( 'NONE', #5472, 1000.000000000000000 ) ;
#12906=ORIENTED_EDGE ( 'NONE', *, *, #11099, .T. ) ;
#12908=VECTOR ( 'NONE', #1310, 1000.000000000000227 ) ;
#12909=DIRECTION ( 'NONE',  ( 0.8415927028326188886, -0.5401126942952620968, 9.975640502598240034E-16 ) ) ;
#12911=CARTESIAN_POINT ( 'NONE',  ( -13.18491133144367211, -15.23222315862922827, 51.10586365543726117 ) ) ;
#12912=ORIENTED_EDGE ( 'NONE', *, *, #10931, .T. ) ;
#12917=CARTESIAN_POINT ( 'NONE',  ( -12.87131257180735844, -22.19373785326158099, 56.85231026484400019 ) ) ;
#12919=DIRECTION ( 'NONE',  ( -8.018662683283438208E-16, 5.975035461963189015E-16, 1.000000000000000000 ) ) ;
#12922=DIRECTION ( 'NONE',  ( 0.8222303661035966771, -0.5691548339926011391, 9.993908270190953088E-16 ) ) ;
#12923=ORIENTED_EDGE ( 'NONE', *, *, #13561, .T. ) ;
#12925=DIRECTION ( 'NONE',  ( -8.018662683283438208E-16, 5.975035461963189015E-16, 1.000000000000000000 ) ) ;
#12927=CARTESIAN_POINT ( 'NONE',  ( -24.93814746875458610, -16.73481322911949931, 57.00231026484397745 ) ) ;
#12929=AXIS2_PLACEMENT_3D ( 'NONE', #5173, #14514, #12996 ) ;
#12930=LINE ( 'NONE', #7161, #12557 ) ;
#12932=FACE_OUTER_BOUND ( 'NONE', #11112, .T. ) ;
#12933=DIRECTION ( 'NONE',  ( -8.018662683283438208E-16, 5.975035461963189015E-16, 1.000000000000000000 ) ) ;
#12935=EDGE_CURVE ( 'NONE', #9275, #2405, #7405, .T. ) ;
#12945=EDGE_CURVE ( 'NONE', #8690, #11659, #11098, .T. ) ;
#12947=CARTESIAN_POINT ( 'NONE',  ( -8.722797460041883610, -15.53942693735753444, 56.85231026484400019 ) ) ;
#12949=ORIENTED_EDGE ( 'NONE', *, *, #3916, .F. ) ;
#12956=LINE ( 'NONE', #2463, #5595 ) ;
#12957=CARTESIAN_POINT ( 'NONE',  ( -7.785174720008381399, -8.727488632615573394, 57.00231026484399166 ) ) ;
#12958=DIRECTION ( 'NONE',  ( 0.5975035461963189576, 0.8018662683283437342, 0.000000000000000000 ) ) ;
#12959=CARTESIAN_POINT ( 'NONE',  ( -6.368730986314239395, -9.491655842995189829, 56.85231026484400019 ) ) ;
#12960=CIRCLE ( 'NONE', #14862, 9.974999999999999645 ) ;
#12965=ORIENTED_EDGE ( 'NONE', *, *, #11028, .T. ) ;
#12971=DIRECTION ( 'NONE',  ( -8.018662683283438208E-16, 5.975035461963189015E-16, 1.000000000000000000 ) ) ;
#12974=AXIS2_PLACEMENT_3D ( 'NONE', #7283, #11969, #3075 ) ;
#12979=ORIENTED_EDGE ( 'NONE', *, *, #9826, .T. ) ;
#12981=DIRECTION ( 'NONE',  ( -0.9885168150181790070, 0.1511109077013141622, -8.829475928589267021E-16 ) ) ;
#12982=VERTEX_POINT ( 'NONE', #4046 ) ;
#12983=ORIENTED_EDGE ( 'NONE', *, *, #4947, .T. ) ;
#12985=CARTESIAN_POINT ( 'NONE',  ( -15.49969986081092088, -13.50737899243822504, 56.85231026484398598 ) ) ;
#12986=VERTEX_POINT ( 'NONE', #12086 ) ;
#12987=DIRECTION ( 'NONE',  ( 0.05771543059946733500, -0.9983330752162417054, 6.427876096865391919E-16 ) ) ;
#12989=AXIS2_PLACEMENT_3D ( 'NONE', #2936, #5150, #10970 ) ;
#12990=LINE ( 'NONE', #12763, #2151 ) ;
#12991=CARTESIAN_POINT ( 'NONE',  ( -21.68801466096620700, -19.44379288755867208, 56.85231026484398598 ) ) ;
#12993=CARTESIAN_POINT ( 'NONE',  ( -7.821737630532772378, -18.34578224045527151, 56.85231026484400019 ) ) ;
#12996=DIRECTION ( 'NONE',  ( 0.5975035461963189576, 0.8018662683283437342, 0.000000000000000000 ) ) ;
#12998=EDGE_CURVE ( 'NONE', #8928, #9118, #6435, .T. ) ;
#12999=CARTESIAN_POINT ( 'NONE',  ( -7.691420491076302213, -11.44776172600821340, 57.00231026484399166 ) ) ;
#13000=ORIENTED_EDGE ( 'NONE', *, *, #4454, .F. ) ;
#13002=ORIENTED_EDGE ( 'NONE', *, *, #934, .F. ) ;
#13003=AXIS2_PLACEMENT_3D ( 'NONE', #2452, #12865, #239 ) ;
#13005=LINE ( 'NONE', #2443, #4115 ) ;
#13006=CARTESIAN_POINT ( 'NONE',  ( -22.33089034576175180, -8.323646113680169378, 56.85231026484398598 ) ) ;
#13009=LINE ( 'NONE', #3437, #7679 ) ;
#13011=VECTOR ( 'NONE', #12909, 1000.000000000000114 ) ;
#13016=EDGE_CURVE ( 'NONE', #6590, #4359, #3973, .T. ) ;
#13019=ADVANCED_FACE ( 'NONE', ( #9423 ), #1239, .T. ) ;
#13022=ORIENTED_EDGE ( 'NONE', *, *, #6985, .F. ) ;
#13023=DIRECTION ( 'NONE',  ( -8.018662683283438208E-16, 5.975035461963189015E-16, 1.000000000000000000 ) ) ;
#13024=ORIENTED_EDGE ( 'NONE', *, *, #2855, .F. ) ;
#13025=DIRECTION ( 'NONE',  ( 8.018662683283438208E-16, -5.975035461963189015E-16, -1.000000000000000000 ) ) ;
#13027=EDGE_LOOP ( 'NONE', ( #8964, #14364, #6335, #5754 ) ) ;
#13029=EDGE_LOOP ( 'NONE', ( #7232, #9867, #8313, #4768 ) ) ;
#13033=FACE_OUTER_BOUND ( 'NONE', #11074, .T. ) ;
#13034=LINE ( 'NONE', #10800, #11255 ) ;
#13036=EDGE_CURVE ( 'NONE', #186, #9490, #8555, .T. ) ;
#13037=CIRCLE ( 'NONE', #3496, 9.974999999999999645 ) ;
#13039=ADVANCED_FACE ( 'NONE', ( #2750 ), #1596, .F. ) ;
#13041=ORIENTED_EDGE ( 'NONE', *, *, #1865, .F. ) ;
#13042=ORIENTED_EDGE ( 'NONE', *, *, #12141, .F. ) ;
#13043=EDGE_LOOP ( 'NONE', ( #4985, #9621, #12071, #1441 ) ) ;
#13044=FACE_OUTER_BOUND ( 'NONE', #3394, .T. ) ;
#13045=EDGE_LOOP ( 'NONE', ( #9926, #12095, #4613, #983 ) ) ;
#13056=LINE ( 'NONE', #10748, #6288 ) ;
#13057=PLANE ( 'NONE',  #7880 ) ;
#13059=ORIENTED_EDGE ( 'NONE', *, *, #4928, .F. ) ;
#13060=VECTOR ( 'NONE', #3896, 1000.000000000000000 ) ;
#13065=EDGE_CURVE ( 'NONE', #3452, #3490, #7112, .T. ) ;
#13071=VERTEX_POINT ( 'NONE', #10572 ) ;
#13073=CARTESIAN_POINT ( 'NONE',  ( -11.30335942247960546, -22.55676305576680818, 57.00231026484399166 ) ) ;
#13079=ORIENTED_EDGE ( 'NONE', *, *, #9532, .F. ) ;
#13081=CARTESIAN_POINT ( 'NONE',  ( -22.58324314276470091, -9.630648466248954875, 57.00231026484397745 ) ) ;
#13083=EDGE_CURVE ( 'NONE', #4089, #15030, #11796, .T. ) ;
#13084=DIRECTION ( 'NONE',  ( 0.8357240892757724637, 0.5491495666976170531, 3.420201433256690644E-16 ) ) ;
#13085=EDGE_CURVE ( 'NONE', #10077, #13839, #832, .T. ) ;
#13086=CARTESIAN_POINT ( 'NONE',  ( -15.12969879992303746, -10.35358246313022335, 57.00231026484397745 ) ) ;
#13087=AXIS2_PLACEMENT_3D ( 'NONE', #5278, #3911, #8567 ) ;
#13088=CARTESIAN_POINT ( 'NONE',  ( -12.66248504435161948, -4.886969368454929352, 56.85231026484398598 ) ) ;
#13089=CARTESIAN_POINT ( 'NONE',  ( -5.615565924346643811, -12.16405426399944112, 54.00231026484399166 ) ) ;
#13091=FACE_OUTER_BOUND ( 'NONE', #2793, .T. ) ;
#13092=VERTEX_POINT ( 'NONE', #1901 ) ;
#13093=PLANE ( 'NONE',  #8089 ) ;
#13095=PLANE ( 'NONE',  #4725 ) ;
#13096=EDGE_LOOP ( 'NONE', ( #8354, #14168, #3677, #9538 ) ) ;
#13097=ORIENTED_EDGE ( 'NONE', *, *, #2103, .T. ) ;
#13098=DIRECTION ( 'NONE',  ( -0.8160499452489514693, -0.5779813897169900905, -3.090169943749478258E-16 ) ) ;
#13099=ORIENTED_EDGE ( 'NONE', *, *, #4117, .F. ) ;
#13100=EDGE_CURVE ( 'NONE', #1960, #8293, #1826, .T. ) ;
#13102=DIRECTION ( 'NONE',  ( 0.7350174335289111349, -0.6780482080269607525, 9.945218953682729003E-16 ) ) ;
#13103=( BOUNDED_CURVE ( )  B_SPLINE_CURVE ( 3, ( #7790, #694, #1920, #4440 ),
 .UNSPECIFIED., .F., .T. ) 
 B_SPLINE_CURVE_WITH_KNOTS ( ( 4, 4 ),
 ( 1.570796326794896114, 3.141592653589792672 ),
 .UNSPECIFIED. ) 
 CURVE ( )  GEOMETRIC_REPRESENTATION_ITEM ( )  RATIONAL_B_SPLINE_CURVE ( ( 1.000000000000000000, 0.8047378541243649375, 0.8047378541243649375, 1.000000000000000000 ) ) 
 REPRESENTATION_ITEM ( '' )  );
#13105=EDGE_CURVE ( 'NONE', #6446, #626, #674, .T. ) ;
#13106=CARTESIAN_POINT ( 'NONE',  ( -15.47724068538499154, -13.46270701644446177, 56.85231026484398598 ) ) ;
#13110=LINE ( 'NONE', #11955, #326 ) ;
#13113=ORIENTED_EDGE ( 'NONE', *, *, #7126, .T. ) ;
#13114=CIRCLE ( 'NONE', #9429, 9.974999999999999645 ) ;
#13115=CARTESIAN_POINT ( 'NONE',  ( -12.91190996461674168, -5.858263458394094236, 57.00231026484397745 ) ) ;
#13117=VERTEX_POINT ( 'NONE', #3119 ) ;
#13119=LINE ( 'NONE', #2625, #14461 ) ;
#13120=ORIENTED_EDGE ( 'NONE', *, *, #3690, .F. ) ;
#13122=DIRECTION ( 'NONE',  ( 0.7737441449604661736, 0.6334982226805353500, 2.419218955996689845E-16 ) ) ;
#13124=EDGE_CURVE ( 'NONE', #9738, #2929, #6699, .T. ) ;
#13129=FACE_OUTER_BOUND ( 'NONE', #3061, .T. ) ;
#13130=DIRECTION ( 'NONE',  ( 8.018662683283438208E-16, -5.975035461963189015E-16, -1.000000000000000000 ) ) ;
#13131=CARTESIAN_POINT ( 'NONE',  ( -11.08622897860377954, -4.561882931743225456, 57.00231026484397745 ) ) ;
#13132=VERTEX_POINT ( 'NONE', #4193 ) ;
#13133=LINE ( 'NONE', #11977, #14375 ) ;
#13135=VERTEX_POINT ( 'NONE', #8852 ) ;
#13136=ORIENTED_EDGE ( 'NONE', *, *, #14468, .F. ) ;
#13137=EDGE_CURVE ( 'NONE', #8177, #2827, #2966, .T. ) ;
#13141=DIRECTION ( 'NONE',  ( 0.5975035461963189576, 0.8018662683283437342, 0.000000000000000000 ) ) ;
#13149=ORIENTED_EDGE ( 'NONE', *, *, #14971, .T. ) ;
#13153=EDGE_CURVE ( 'NONE', #10559, #3186, #13532, .T. ) ;
#13157=CARTESIAN_POINT ( 'NONE',  ( -19.05456510292772876, -4.187316862259577555, 57.00231026484397745 ) ) ;
#13159=CARTESIAN_POINT ( 'NONE',  ( -15.49969986081092088, -13.50737899243822504, 56.85231026484398598 ) ) ;
#13166=EDGE_LOOP ( 'NONE', ( #12979, #3347, #14498, #3338 ) ) ;
#13167=DIRECTION ( 'NONE',  ( -0.2301973227387161258, 0.9731439732146150989, -7.660444431189777453E-16 ) ) ;
#13168=DIRECTION ( 'NONE',  ( -0.3956847857120157075, 0.9183863840214729901, -8.660254037844387408E-16 ) ) ;
#13170=EDGE_CURVE ( 'NONE', #12295, #13665, #4425, .T. ) ;
#13171=ORIENTED_EDGE ( 'NONE', *, *, #13835, .F. ) ;
#13172=CARTESIAN_POINT ( 'NONE',  ( -16.26465502354534465, -4.464365468230401923, 56.85231026484398598 ) ) ;
#13177=EDGE_CURVE ( 'NONE', #1021, #10935, #6471, .T. ) ;
#13178=CARTESIAN_POINT ( 'NONE',  ( -10.22560374232860347, -19.62253721876480483, 56.85231026484400019 ) ) ;
#13179=VERTEX_POINT ( 'NONE', #754 ) ;
#13180=DIRECTION ( 'NONE',  ( 0.5975035461963188466, 0.8018662683283438453, 0.000000000000000000 ) ) ;
#13183=CARTESIAN_POINT ( 'NONE',  ( -18.15085299098534577, -14.64962258016358199, 56.75231026484397745 ) ) ;
#13184=VECTOR ( 'NONE', #325, 1000.000000000000114 ) ;
#13188=CARTESIAN_POINT ( 'NONE',  ( -7.654212976755197850, -10.04550297615607768, 57.00231026484399166 ) ) ;
#13189=EDGE_CURVE ( 'NONE', #14941, #9624, #10145, .T. ) ;
#13190=VERTEX_POINT ( 'NONE', #4352 ) ;
#13191=CARTESIAN_POINT ( 'NONE',  ( -7.711221940648826489, -11.37542292179617753, 57.00231026484399166 ) ) ;
#13193=ORIENTED_EDGE ( 'NONE', *, *, #9548, .T. ) ;
#13195=EDGE_CURVE ( 'NONE', #1146, #13135, #13681, .T. ) ;
#13197=VERTEX_POINT ( 'NONE', #9076 ) ;
#13198=ORIENTED_EDGE ( 'NONE', *, *, #12998, .F. ) ;
#13199=CARTESIAN_POINT ( 'NONE',  ( -12.81093390292747536, -9.898980784960684787, 48.00231026484398456 ) ) ;
#13206=DIRECTION ( 'NONE',  ( 0.6601155939154559338, -0.7511640317997426708, 9.781476007338054812E-16 ) ) ;
#13208=ADVANCED_FACE ( 'NONE', ( #1743 ), #6400, .T. ) ;
#13211=ADVANCED_FACE ( 'NONE', ( #15046 ), #1272, .F. ) ;
#13220=CARTESIAN_POINT ( 'NONE',  ( -15.80242800153736837, -16.08775797096295435, 51.00231026484399166 ) ) ;
#13221=DIRECTION ( 'NONE',  ( -0.7276687409742212953, -0.6859287159822015090, -1.736481776669299976E-16 ) ) ;
#13222=CARTESIAN_POINT ( 'NONE',  ( -15.49969986081092088, -13.50737899243822504, 57.00231026484397745 ) ) ;
#13224=ORIENTED_EDGE ( 'NONE', *, *, #10180, .F. ) ;
#13226=CARTESIAN_POINT ( 'NONE',  ( -15.53979317422733786, -13.47750381512840967, 56.85231026484398598 ) ) ;
#13227=VERTEX_POINT ( 'NONE', #1123 ) ;
#13231=CARTESIAN_POINT ( 'NONE',  ( -15.51120972694785749, -13.45872179377749589, 56.85231026484398598 ) ) ;
#13233=DIRECTION ( 'NONE',  ( 8.018662683283438208E-16, -5.975035461963189015E-16, -1.000000000000000000 ) ) ;
#13234=LINE ( 'NONE', #4814, #618 ) ;
#13237=EDGE_CURVE ( 'NONE', #11236, #12600, #12845, .T. ) ;
#13243=CARTESIAN_POINT ( 'NONE',  ( -18.68395610307571530, -20.92841410781112899, 57.00231026484397745 ) ) ;
#13247=ORIENTED_EDGE ( 'NONE', *, *, #14282, .F. ) ;
#13249=ORIENTED_EDGE ( 'NONE', *, *, #3539, .F. ) ;
#13251=CARTESIAN_POINT ( 'NONE',  ( -22.56290636796585503, -13.91571566392944526, 57.00231026484397745 ) ) ;
#13255=VECTOR ( 'NONE', #8799, 1000.000000000000227 ) ;
#13260=LINE ( 'NONE', #4218, #5674 ) ;
#13261=AXIS2_PLACEMENT_3D ( 'NONE', #7831, #3267, #8065 ) ;
#13262=DIRECTION ( 'NONE',  ( -0.9885168150181788960, 0.1511109077013150503, -8.829475928589270966E-16 ) ) ;
#13263=AXIS2_PLACEMENT_3D ( 'NONE', #9648, #9870, #2609 ) ;
#13264=VERTEX_POINT ( 'NONE', #12688 ) ;
#13266=ORIENTED_EDGE ( 'NONE', *, *, #14393, .F. ) ;
#13267=CIRCLE ( 'NONE', #3230, 9.974999999999999645 ) ;
#13268=CIRCLE ( 'NONE', #1280, 4.499999999999998224 ) ;
#13269=DIRECTION ( 'NONE',  ( 0.5975035461963188466, 0.8018662683283437342, 0.000000000000000000 ) ) ;
#13271=DIRECTION ( 'NONE',  ( 0.3956847857120158740, -0.9183863840214728791, 0.000000000000000000 ) ) ;
#13274=CARTESIAN_POINT ( 'NONE',  ( -23.52886110248590867, -17.73748770914800943, 56.85231026484398598 ) ) ;
#13276=VECTOR ( 'NONE', #7114, 1000.000000000000114 ) ;
#13277=EDGE_CURVE ( 'NONE', #14554, #8561, #2201, .T. ) ;
#13278=CYLINDRICAL_SURFACE ( 'NONE', #9482, 5.000000000000000000 ) ;
#13280=CARTESIAN_POINT ( 'NONE',  ( -15.49969986081092088, -13.50737899243822504, 57.00231026484397745 ) ) ;
#13281=EDGE_LOOP ( 'NONE', ( #2003, #7519, #14644, #2681 ) ) ;
#13285=ORIENTED_EDGE ( 'NONE', *, *, #2855, .T. ) ;
#13288=ORIENTED_EDGE ( 'NONE', *, *, #5850, .F. ) ;
#13289=EDGE_CURVE ( 'NONE', #14240, #7684, #4650, .T. ) ;
#13293=EDGE_CURVE ( 'NONE', #3663, #8391, #6850, .T. ) ;
#13295=CARTESIAN_POINT ( 'NONE',  ( -13.16883223745437448, -21.23902216335526916, 56.85231026484400019 ) ) ;
#13299=CIRCLE ( 'NONE', #585, 9.974999999999999645 ) ;
#13301=CARTESIAN_POINT ( 'NONE',  ( -16.26465502354534465, -4.464365468230401923, 57.00231026484397745 ) ) ;
#13307=ORIENTED_EDGE ( 'NONE', *, *, #11666, .F. ) ;
#13309=EDGE_LOOP ( 'NONE', ( #8563, #3604, #10796, #13868 ) ) ;
#13310=CARTESIAN_POINT ( 'NONE',  ( -14.95642007119148076, -3.547184613301321399, 54.00231026484397745 ) ) ;
#13313=EDGE_CURVE ( 'NONE', #7829, #8731, #10303, .T. ) ;
#13318=ORIENTED_EDGE ( 'NONE', *, *, #2319, .T. ) ;
#13320=DIRECTION ( 'NONE',  ( 8.018662683283438208E-16, -5.975035461963189015E-16, -1.000000000000000000 ) ) ;
#13321=VECTOR ( 'NONE', #8051, 1000.000000000000000 ) ;
#13322=ORIENTED_EDGE ( 'NONE', *, *, #2223, .T. ) ;
#13325=ORIENTED_EDGE ( 'NONE', *, *, #13682, .F. ) ;
#13326=ORIENTED_EDGE ( 'NONE', *, *, #12628, .F. ) ;
#13328=DIRECTION ( 'NONE',  ( 0.5975035461963189576, 0.8018662683283437342, 0.000000000000000000 ) ) ;
#13329=PLANE ( 'NONE',  #9000 ) ;
#13330=( BOUNDED_CURVE ( )  B_SPLINE_CURVE ( 3, ( #14043, #3859, #46, #10668 ),
 .UNSPECIFIED., .F., .F. ) 
 B_SPLINE_CURVE_WITH_KNOTS ( ( 4, 4 ),
 ( -8.881784197001252323E-16, 1.570796326794896114 ),
 .UNSPECIFIED. ) 
 CURVE ( )  GEOMETRIC_REPRESENTATION_ITEM ( )  RATIONAL_B_SPLINE_CURVE ( ( 1.000000000000000000, 0.8047378541243649375, 0.8047378541243649375, 1.000000000000000000 ) ) 
 REPRESENTATION_ITEM ( '' )  );
#13331=DIRECTION ( 'NONE',  ( -8.018662683283438208E-16, 5.975035461963189015E-16, 1.000000000000000000 ) ) ;
#13332=VECTOR ( 'NONE', #5818, 1000.000000000000114 ) ;
#13336=DIRECTION ( 'NONE',  ( -0.9868311969055004740, -0.1617534816134024167, -6.946583704589977600E-16 ) ) ;
#13337=CARTESIAN_POINT ( 'NONE',  ( -6.540243082598547808, -14.95284924095401458, 56.85231026484400019 ) ) ;
#13338=ORIENTED_EDGE ( 'NONE', *, *, #2611, .F. ) ;
#13340=ORIENTED_EDGE ( 'NONE', *, *, #9974, .T. ) ;
#13342=EDGE_CURVE ( 'NONE', #13608, #2908, #10383, .T. ) ;
#13343=ORIENTED_EDGE ( 'NONE', *, *, #11686, .T. ) ;
#13345=CARTESIAN_POINT ( 'NONE',  ( -17.20133171717847631, -6.639650181150215325, 56.85231026484398598 ) ) ;
#13348=DIRECTION ( 'NONE',  ( 0.5975035461963189576, 0.8018662683283437342, 0.000000000000000000 ) ) ;
#13349=VERTEX_POINT ( 'NONE', #61 ) ;
#13351=CARTESIAN_POINT ( 'NONE',  ( -5.524802968312264362, -13.55273297815671008, 54.00231026484399166 ) ) ;
#13353=VERTEX_POINT ( 'NONE', #10610 ) ;
#13355=ADVANCED_FACE ( 'NONE', ( #14975 ), #9389, .F. ) ;
#13357=ORIENTED_EDGE ( 'NONE', *, *, #3431, .F. ) ;
#13358=DIRECTION ( 'NONE',  ( -8.018662683283438208E-16, 5.975035461963189015E-16, 1.000000000000000000 ) ) ;
#13364=CARTESIAN_POINT ( 'NONE',  ( -12.84854673063650132, -12.36513540471286454, 56.75231026484397745 ) ) ;
#13369=EDGE_LOOP ( 'NONE', ( #9770, #2955, #4810, #5699 ) ) ;
#13370=ADVANCED_FACE ( 'NONE', ( #3800 ), #1355, .F. ) ;
#13373=EDGE_LOOP ( 'NONE', ( #7522, #4885, #5515, #5078 ) ) ;
#13374=CARTESIAN_POINT ( 'NONE',  ( -16.42437072798637843, -22.03270794722917714, 57.00231026484399166 ) ) ;
#13379=EDGE_CURVE ( 'NONE', #5071, #9234, #2581, .T. ) ;
#13382=VECTOR ( 'NONE', #12072, 1000.000000000000000 ) ;
#13383=EDGE_CURVE ( 'NONE', #1146, #1022, #8381, .T. ) ;
#13387=EDGE_LOOP ( 'NONE', ( #13874, #14210, #15, #8971 ) ) ;
#13389=DIRECTION ( 'NONE',  ( 0.5975035461963189576, 0.8018662683283437342, 0.000000000000000000 ) ) ;
#13390=ORIENTED_EDGE ( 'NONE', *, *, #2990, .T. ) ;
#13391=EDGE_CURVE ( 'NONE', #13854, #8839, #12305, .T. ) ;
#13392=ORIENTED_EDGE ( 'NONE', *, *, #11099, .F. ) ;
#13394=ORIENTED_EDGE ( 'NONE', *, *, #159, .F. ) ;
#13395=ORIENTED_EDGE ( 'NONE', *, *, #5790, .F. ) ;
#13396=AXIS2_PLACEMENT_3D ( 'NONE', #7799, #12488, #2002 ) ;
#13397=CARTESIAN_POINT ( 'NONE',  ( -22.64353467404651354, -6.545608444567307949, 54.00231026484397745 ) ) ;
#13399=DIRECTION ( 'NONE',  ( 0.8885476655824671166, 0.4587843131450204393, 4.383711467890819071E-16 ) ) ;
#13409=ORIENTED_EDGE ( 'NONE', *, *, #1383, .T. ) ;
#13411=LINE ( 'NONE', #6279, #3989 ) ;
#13413=VERTEX_POINT ( 'NONE', #11991 ) ;
#13414=AXIS2_PLACEMENT_3D ( 'NONE', #14633, #4156, #8736 ) ;
#13415=CARTESIAN_POINT ( 'NONE',  ( -17.86883904694317238, -3.817807045405071431, 54.00231026484397745 ) ) ;
#13416=DIRECTION ( 'NONE',  ( -8.018662683283439195E-16, 5.975035461963190001E-16, 1.000000000000000000 ) ) ;
#13417=ORIENTED_EDGE ( 'NONE', *, *, #3080, .T. ) ;
#13418=CARTESIAN_POINT ( 'NONE',  ( -9.760873592531980947, -5.348549538251076818, 57.00231026484397745 ) ) ;
#13419=AXIS2_PLACEMENT_3D ( 'NONE', #11891, #10437, #15104 ) ;
#13420=CARTESIAN_POINT ( 'NONE',  ( -5.966797098401854349, -16.44411015522000241, 56.85231026484400019 ) ) ;
#13424=EDGE_CURVE ( 'NONE', #1349, #13936, #5029, .T. ) ;
#13425=DIRECTION ( 'NONE',  ( -8.018662683283438208E-16, 5.975035461963189015E-16, 1.000000000000000000 ) ) ;
#13426=CARTESIAN_POINT ( 'NONE',  ( -13.72291223624743139, -3.691898834178109379, 54.00231026484399166 ) ) ;
#13428=ORIENTED_EDGE ( 'NONE', *, *, #638, .T. ) ;
#13430=CARTESIAN_POINT ( 'NONE',  ( -15.49969986081092088, -13.50737899243822504, 57.00231026484397745 ) ) ;
#13432=ORIENTED_EDGE ( 'NONE', *, *, #6320, .T. ) ;
#13435=ORIENTED_EDGE ( 'NONE', *, *, #5850, .T. ) ;
#13436=AXIS2_PLACEMENT_3D ( 'NONE', #11410, #9111, #15006 ) ;
#13439=CARTESIAN_POINT ( 'NONE',  ( -16.41401162527548507, -4.478243707298169340, 56.85231026484398598 ) ) ;
#13440=CARTESIAN_POINT ( 'NONE',  ( -11.08622897860377776, -4.561882931743227232, 54.00231026484399166 ) ) ;
#13442=PLANE ( 'NONE',  #3372 ) ;
#13445=CARTESIAN_POINT ( 'NONE',  ( -13.26502611401716081, -13.76954925274777075, 51.25231026484399166 ) ) ;
#13446=ORIENTED_EDGE ( 'NONE', *, *, #8917, .F. ) ;
#13447=DIRECTION ( 'NONE',  ( -0.4587843131450204948, 0.8885476655824671166, -8.987940462991649850E-16 ) ) ;
#13449=ORIENTED_EDGE ( 'NONE', *, *, #6966, .F. ) ;
#13450=CIRCLE ( 'NONE', #13934, 9.974999999999999645 ) ;
#13451=CARTESIAN_POINT ( 'NONE',  ( -15.49969986081092088, -13.50737899243822504, 57.00231026484397745 ) ) ;
#13452=CARTESIAN_POINT ( 'NONE',  ( -7.480766807389218620, -12.55450823271226746, 56.85231026484400019 ) ) ;
#13454=CARTESIAN_POINT ( 'NONE',  ( -15.49969986081092088, -13.50737899243822504, 56.85231026484398598 ) ) ;
#13455=CARTESIAN_POINT ( 'NONE',  ( -12.84854673063650132, -12.36513540471286454, 56.75231026484397745 ) ) ;
#13456=EDGE_CURVE ( 'NONE', #33, #10747, #6159, .T. ) ;
#13460=CARTESIAN_POINT ( 'NONE',  ( -18.72761429428784297, -5.025526694139714756, 56.85231026484398598 ) ) ;
#13462=ORIENTED_EDGE ( 'NONE', *, *, #14813, .T. ) ;
#13465=ORIENTED_EDGE ( 'NONE', *, *, #10761, .T. ) ;
#13470=VERTEX_POINT ( 'NONE', #14206 ) ;
#13474=DIRECTION ( 'NONE',  ( 0.5975035461963189576, 0.8018662683283437342, 0.000000000000000000 ) ) ;
#13475=EDGE_CURVE ( 'NONE', #12986, #3416, #8613, .T. ) ;
#13476=CARTESIAN_POINT ( 'NONE',  ( -14.26755283655060680, -21.48817241857114269, 56.85231026484400019 ) ) ;
#13479=CARTESIAN_POINT ( 'NONE',  ( -15.83606446161809522, -16.37446674635458166, 56.75231026484397745 ) ) ;
#13480=ORIENTED_EDGE ( 'NONE', *, *, #13847, .F. ) ;
#13481=PLANE ( 'NONE',  #5901 ) ;
#13482=ORIENTED_EDGE ( 'NONE', *, *, #3571, .T. ) ;
#13483=DIRECTION ( 'NONE',  ( -0.9645173894937584258, -0.2640193276336892381, -6.156614753256587028E-16 ) ) ;
#13485=VERTEX_POINT ( 'NONE', #14132 ) ;
#13487=CARTESIAN_POINT ( 'NONE',  ( -20.60611791317904107, -19.76323582219775687, 56.85231026484398598 ) ) ;
#13489=CIRCLE ( 'NONE', #6625, 9.974999999999999645 ) ;
#13491=CARTESIAN_POINT ( 'NONE',  ( -22.08930316869620825, -18.17457871440291228, 56.85231026484398598 ) ) ;
#13492=DIRECTION ( 'NONE',  ( 0.8885476655824650072, 0.4587843131450243805, 4.383711467890778149E-16 ) ) ;
#13493=ADVANCED_FACE ( 'NONE', ( #3655 ), #8304, .F. ) ;
#13494=VECTOR ( 'NONE', #991, 1000.000000000000000 ) ;
#13495=SHAPE_REPRESENTATION ( 'Dial Adjustment Screw', ( #6789 ), #8995 ) ;
#13496=VECTOR ( 'NONE', #14296, 1000.000000000000000 ) ;
#13497=AXIS2_PLACEMENT_3D ( 'NONE', #4478, #5763, #11509 ) ;
#13498=FACE_OUTER_BOUND ( 'NONE', #14207, .T. ) ;
#13499=VERTEX_POINT ( 'NONE', #11285 ) ;
#13501=EDGE_LOOP ( 'NONE', ( #4891, #10791, #5220, #11365 ) ) ;
#13503=LINE ( 'NONE', #3015, #56 ) ;
#13504=ORIENTED_EDGE ( 'NONE', *, *, #9908, .F. ) ;
#13505=LINE ( 'NONE', #506, #10806 ) ;
#13506=ADVANCED_FACE ( 'NONE', ( #1726 ), #12363, .F. ) ;
#13507=VECTOR ( 'NONE', #14797, 1000.000000000000000 ) ;
#13508=AXIS2_PLACEMENT_3D ( 'NONE', #1789, #11120, #6292 ) ;
#13511=DIRECTION ( 'NONE',  ( -8.018662683283439195E-16, 5.975035461963190001E-16, 1.000000000000000000 ) ) ;
#13513=CARTESIAN_POINT ( 'NONE',  ( -18.10194853779420399, -23.13696500758646835, 56.85231026484400019 ) ) ;
#13516=FACE_OUTER_BOUND ( 'NONE', #10053, .T. ) ;
#13518=DIRECTION ( 'NONE',  ( -8.018662683283438208E-16, 5.975035461963189015E-16, 1.000000000000000000 ) ) ;
#13521=LINE ( 'NONE', #14741, #4704 ) ;
#13522=CARTESIAN_POINT ( 'NONE',  ( -17.88573767796789582, -14.53539822139104842, 51.00231026484399166 ) ) ;
#13525=CARTESIAN_POINT ( 'NONE',  ( -15.47724068538499154, -13.46270701644446177, 56.85231026484398598 ) ) ;
#13526=EDGE_CURVE ( 'NONE', #4722, #11072, #8980, .T. ) ;
#13527=EDGE_CURVE ( 'NONE', #612, #7478, #580, .T. ) ;
#13532=LINE ( 'NONE', #7774, #3037 ) ;
#13533=VERTEX_POINT ( 'NONE', #13513 ) ;
#13536=VECTOR ( 'NONE', #657, 1000.000000000000114 ) ;
#13541=VECTOR ( 'NONE', #13633, 1000.000000000000114 ) ;
#13542=EDGE_CURVE ( 'NONE', #10935, #8839, #6378, .T. ) ;
#13543=CARTESIAN_POINT ( 'NONE',  ( -21.79367780933653620, -21.24601366423100401, 57.00231026484397745 ) ) ;
#13546=CARTESIAN_POINT ( 'NONE',  ( -10.08476707729037614, -21.88467736064467672, 56.85231026484400019 ) ) ;
#13547=LINE ( 'NONE', #13618, #11843 ) ;
#13549=DIRECTION ( 'NONE',  ( -8.018662683283438208E-16, 5.975035461963189015E-16, 1.000000000000000000 ) ) ;
#13551=CARTESIAN_POINT ( 'NONE',  ( -15.49969986081091022, -13.50737899243823215, 46.00231026484398456 ) ) ;
#13553=DIRECTION ( 'NONE',  ( -8.018662683283438208E-16, 5.975035461963189015E-16, 1.000000000000000000 ) ) ;
#13555=VERTEX_POINT ( 'NONE', #7610 ) ;
#13557=ORIENTED_EDGE ( 'NONE', *, *, #7383, .T. ) ;
#13561=EDGE_CURVE ( 'NONE', #6010, #14217, #14877, .T. ) ;
#13567=MECHANICAL_DESIGN_GEOMETRIC_PRESENTATION_REPRESENTATION('',(#1096),#2802);
#13569=LINE ( 'NONE', #13491, #13694 ) ;
#13572=CARTESIAN_POINT ( 'NONE',  ( -17.12834591918736749, -6.622385381944812188, 57.00231026484397745 ) ) ;
#13573=LINE ( 'NONE', #4160, #12251 ) ;
#13577=DIRECTION ( 'NONE',  ( -0.8018662683283436232, 0.5975035461963189576, -9.999999999999998805E-16 ) ) ;
#13578=ORIENTED_EDGE ( 'NONE', *, *, #2797, .T. ) ;
#13584=CARTESIAN_POINT ( 'NONE',  ( -12.37415300023346809, -4.034703455804747207, 57.00231026484397745 ) ) ;
#13587=LINE ( 'NONE', #13660, #9959 ) ;
#13589=LINE ( 'NONE', #14580, #7901 ) ;
#13590=PLANE ( 'NONE',  #6661 ) ;
#13592=ORIENTED_EDGE ( 'NONE', *, *, #6252, .T. ) ;
#13594=DIRECTION ( 'NONE',  ( -0.9988970074402867549, 0.04695496274985035828, -8.290375725550441510E-16 ) ) ;
#13602=LINE ( 'NONE', #12454, #2445 ) ;
#13604=LINE ( 'NONE', #9150, #3343 ) ;
#13605=EDGE_CURVE ( 'NONE', #7024, #9434, #8865, .T. ) ;
#13607=CARTESIAN_POINT ( 'NONE',  ( -13.09722856071139496, -21.21670818843173478, 57.00231026484399166 ) ) ;
#13608=VERTEX_POINT ( 'NONE', #14581 ) ;
#13612=VERTEX_POINT ( 'NONE', #4100 ) ;
#13613=CARTESIAN_POINT ( 'NONE',  ( -15.36741682587554969, -22.58172476492607572, 56.85231026484400019 ) ) ;
#13614=EDGE_LOOP ( 'NONE', ( #12912, #1014, #7027, #15016 ) ) ;
#13616=CARTESIAN_POINT ( 'NONE',  ( -22.42051587769119791, -8.443926053929422082, 56.85231026484398598 ) ) ;
#13617=CARTESIAN_POINT ( 'NONE',  ( -8.131654986474892155, -16.81240013151894175, 57.00231026484399166 ) ) ;
#13618=CARTESIAN_POINT ( 'NONE',  ( -16.24959055444668365, -20.54292544936667397, 56.85231026484400019 ) ) ;
#13621=ADVANCED_FACE ( 'NONE', ( #8909 ), #13590, .T. ) ;
#13625=PLANE ( 'NONE',  #7391 ) ;
#13626=EDGE_CURVE ( 'NONE', #1039, #13227, #4486, .T. ) ;
#13630=LINE ( 'NONE', #8878, #5210 ) ;
#13632=CYLINDRICAL_SURFACE ( 'NONE', #13396, 9.974999999999999645 ) ;
#13633=DIRECTION ( 'NONE',  ( -0.5491495666976170531, 0.8357240892757724637, -9.396926207859082113E-16 ) ) ;
#13634=ORIENTED_EDGE ( 'NONE', *, *, #10566, .F. ) ;
#13640=AXIS2_PLACEMENT_3D ( 'NONE', #6345, #2914, #12171 ) ;
#13642=LINE ( 'NONE', #13572, #11507 ) ;
#13645=ORIENTED_EDGE ( 'NONE', *, *, #8439, .T. ) ;
#13647=VERTEX_POINT ( 'NONE', #2260 ) ;
#13651=CARTESIAN_POINT ( 'NONE',  ( -22.54723635769173384, -9.564857042577559199, 56.85231026484398598 ) ) ;
#13653=ORIENTED_EDGE ( 'NONE', *, *, #13153, .F. ) ;
#13654=ADVANCED_FACE ( 'NONE', ( #13735 ), #4406, .T. ) ;
#13659=EDGE_CURVE ( 'NONE', #3165, #8545, #9369, .T. ) ;
#13660=CARTESIAN_POINT ( 'NONE',  ( -16.84408283975263032, -15.31157809617700316, 51.00231026484399166 ) ) ;
#13663=CARTESIAN_POINT ( 'NONE',  ( -15.49969986081092088, -13.50737899243822504, 56.85231026484398598 ) ) ;
#13665=VERTEX_POINT ( 'NONE', #3556 ) ;
#13667=VECTOR ( 'NONE', #1361, 1000.000000000000000 ) ;
#13669=EDGE_LOOP ( 'NONE', ( #9298, #10490, #782, #2098 ) ) ;
#13671=ORIENTED_EDGE ( 'NONE', *, *, #9627, .T. ) ;
#13674=DIRECTION ( 'NONE',  ( -0.3857661296576155308, -0.9225966037272105291, 2.419218955996680478E-16 ) ) ;
#13678=SHAPE_DEFINITION_REPRESENTATION ( #423, #13495 ) ;
#13680=DIRECTION ( 'NONE',  ( -8.018662683283438208E-16, 5.975035461963189015E-16, 1.000000000000000000 ) ) ;
#13681=LINE ( 'NONE', #7841, #7671 ) ;
#13682=EDGE_CURVE ( 'NONE', #9718, #5071, #11657, .T. ) ;
#13683=ORIENTED_EDGE ( 'NONE', *, *, #12174, .F. ) ;
#13686=LINE ( 'NONE', #7846, #8149 ) ;
#13687=ORIENTED_EDGE ( 'NONE', *, *, #9889, .F. ) ;
#13689=VERTEX_POINT ( 'NONE', #6904 ) ;
#13690=ORIENTED_EDGE ( 'NONE', *, *, #10584, .F. ) ;
#13691=DIRECTION ( 'NONE',  ( 8.018662683283438208E-16, -5.975035461963189015E-16, -1.000000000000000000 ) ) ;
#13692=DIRECTION ( 'NONE',  ( 8.018662683283438208E-16, -5.975035461963189015E-16, -1.000000000000000000 ) ) ;
#13693=EDGE_CURVE ( 'NONE', #7394, #337, #2412, .T. ) ;
#13694=VECTOR ( 'NONE', #6358, 1000.000000000000114 ) ;
#13695=PLANE ( 'NONE',  #6881 ) ;
#13699=DIRECTION ( 'NONE',  ( 0.7953815700667019595, 0.6061090314442014737, 2.756373558169989438E-16 ) ) ;
#13700=DIRECTION ( 'NONE',  ( -0.1960948578651675878, 0.9805849309054466278, -7.431448254773955467E-16 ) ) ;
#13702=LINE ( 'NONE', #5434, #10298 ) ;
#13704=DIRECTION ( 'NONE',  ( -8.018662683283438208E-16, 5.975035461963189015E-16, 1.000000000000000000 ) ) ;
#13705=DIRECTION ( 'NONE',  ( -0.01206535623792160013, -0.9999272109403024578, 5.877852522924710079E-16 ) ) ;
#13706=ORIENTED_EDGE ( 'NONE', *, *, #12823, .F. ) ;
#13713=FACE_OUTER_BOUND ( 'NONE', #8512, .T. ) ;
#13714=ORIENTED_EDGE ( 'NONE', *, *, #12063, .F. ) ;
#13717=ORIENTED_EDGE ( 'NONE', *, *, #6626, .F. ) ;
#13719=ORIENTED_EDGE ( 'NONE', *, *, #8347, .T. ) ;
#13720=LINE ( 'NONE', #13945, #4566 ) ;
#13721=ORIENTED_EDGE ( 'NONE', *, *, #5260, .F. ) ;
#13723=AXIS2_PLACEMENT_3D ( 'NONE', #3753, #10484, #11555 ) ;
#13724=DIRECTION ( 'NONE',  ( 8.018662683283438208E-16, -5.975035461963189015E-16, -1.000000000000000000 ) ) ;
#13725=VERTEX_POINT ( 'NONE', #5540 ) ;
#13728=EDGE_CURVE ( 'NONE', #10111, #8833, #2183, .T. ) ;
#13729=CARTESIAN_POINT ( 'NONE',  ( -25.43486656742121355, -12.61682438329676081, 56.85231026484398598 ) ) ;
#13731=DIRECTION ( 'NONE',  ( -0.1617534816134024167, 0.9868311969055004740, -7.193398003386505973E-16 ) ) ;
#13732=AXIS2_PLACEMENT_3D ( 'NONE', #3404, #10436, #12393 ) ;
#13735=FACE_OUTER_BOUND ( 'NONE', #10138, .T. ) ;
#13736=CARTESIAN_POINT ( 'NONE',  ( -17.72867398697626129, -22.30470383268854562, 57.00231026484399166 ) ) ;
#13737=ORIENTED_EDGE ( 'NONE', *, *, #1688, .T. ) ;
#13742=AXIS2_PLACEMENT_3D ( 'NONE', #9214, #9141, #11371 ) ;
#13744=CIRCLE ( 'NONE', #9834, 9.974999999999999645 ) ;
#13749=AXIS2_PLACEMENT_3D ( 'NONE', #9576, #9424, #5894 ) ;
#13751=EDGE_CURVE ( 'NONE', #13829, #5017, #3258, .T. ) ;
#13753=CARTESIAN_POINT ( 'NONE',  ( -7.594860258898399330, -10.18326093375929631, 57.00231026484399166 ) ) ;
#13754=CARTESIAN_POINT ( 'NONE',  ( -21.17290370923395670, -9.280041403099277275, 56.85231026484398598 ) ) ;
#13759=LINE ( 'NONE', #3282, #7663 ) ;
#13761=PLANE ( 'NONE',  #2048 ) ;
#13762=ORIENTED_EDGE ( 'NONE', *, *, #4779, .F. ) ;
#13763=CARTESIAN_POINT ( 'NONE',  ( -21.89842656004739396, -7.071732433740530510, 56.85231026484398598 ) ) ;
#13765=EDGE_CURVE ( 'NONE', #8005, #3663, #12595, .T. ) ;
#13766=ADVANCED_FACE ( 'NONE', ( #10285 ), #14956, .T. ) ;
#13767=VECTOR ( 'NONE', #3861, 1000.000000000000114 ) ;
#13768=VECTOR ( 'NONE', #13784, 999.9999999999998863 ) ;
#13769=ADVANCED_FACE ( 'NONE', ( #10515 ), #1037, .T. ) ;
#13771=VECTOR ( 'NONE', #812, 1000.000000000000000 ) ;
#13774=DIRECTION ( 'NONE',  ( 8.018662683283438208E-16, -5.975035461963189015E-16, -1.000000000000000000 ) ) ;
#13776=FACE_OUTER_BOUND ( 'NONE', #8671, .T. ) ;
#13777=EDGE_CURVE ( 'NONE', #11236, #11735, #10012, .T. ) ;
#13779=DIRECTION ( 'NONE',  ( 0.9988970074402866439, -0.04695496274985035134, 8.290375725550441510E-16 ) ) ;
#13780=ORIENTED_EDGE ( 'NONE', *, *, #6770, .F. ) ;
#13784=DIRECTION ( 'NONE',  ( 0.6334982226805337957, -0.7737441449604673949, 9.702957262759957177E-16 ) ) ;
#13786=ORIENTED_EDGE ( 'NONE', *, *, #13847, .T. ) ;
#13787=CARTESIAN_POINT ( 'NONE',  ( -12.58343141761905670, -12.25091104594033098, 57.00231026484397745 ) ) ;
#13788=ORIENTED_EDGE ( 'NONE', *, *, #5026, .T. ) ;
#13790=CARTESIAN_POINT ( 'NONE',  ( -16.49725497239786520, -3.582384846377123733, 56.85231026484398598 ) ) ;
#13791=VECTOR ( 'NONE', #6327, 1000.000000000000000 ) ;
#13793=ORIENTED_EDGE ( 'NONE', *, *, #13682, .T. ) ;
#13796=EDGE_LOOP ( 'NONE', ( #4753, #7933, #1129, #6949 ) ) ;
#13799=PLANE ( 'NONE',  #7491 ) ;
#13805=ADVANCED_FACE ( 'NONE', ( #6710 ), #12552, .F. ) ;
#13806=CARTESIAN_POINT ( 'NONE',  ( -18.72761429428784297, -5.025526694139714756, 56.85231026484398598 ) ) ;
#13808=VECTOR ( 'NONE', #2464, 1000.000000000000000 ) ;
#13809=DIRECTION ( 'NONE',  ( 8.018662683283438208E-16, -5.975035461963189015E-16, -1.000000000000000000 ) ) ;
#13811=DIRECTION ( 'NONE',  ( -0.3204693369899910826, -0.9472588896649086765, 3.090169943749478258E-16 ) ) ;
#13812=CARTESIAN_POINT ( 'NONE',  ( -12.98295438134161195, -5.834228258119843247, 57.00231026484397745 ) ) ;
#13816=EDGE_LOOP ( 'NONE', ( #11630, #8309, #5419, #396 ) ) ;
#13819=EDGE_CURVE ( 'NONE', #9794, #7829, #2980, .T. ) ;
#13821=PLANE ( 'NONE',  #7424 ) ;
#13825=CARTESIAN_POINT ( 'NONE',  ( -20.64795620320353109, -18.36032465801230273, 56.85231026484398598 ) ) ;
#13826=PLANE ( 'NONE',  #8692 ) ;
#13829=VERTEX_POINT ( 'NONE', #13546 ) ;
#13831=ADVANCED_FACE ( 'NONE', ( #689 ), #2068, .F. ) ;
#13835=EDGE_CURVE ( 'NONE', #9099, #4294, #13268, .T. ) ;
#13838=PLANE ( 'NONE',  #14748 ) ;
#13839=VERTEX_POINT ( 'NONE', #13617 ) ;
#13840=FACE_OUTER_BOUND ( 'NONE', #11497, .T. ) ;
#13847=EDGE_CURVE ( 'NONE', #8177, #5325, #12473, .T. ) ;
#13848=ADVANCED_FACE ( 'NONE', ( #845 ), #5424, .F. ) ;
#13849=CARTESIAN_POINT ( 'NONE',  ( -15.49969986081086226, -13.50737899243826767, -13.99768973515600301 ) ) ;
#13854=VERTEX_POINT ( 'NONE', #9015 ) ;
#13856=ORIENTED_EDGE ( 'NONE', *, *, #2144, .F. ) ;
#13858=ORIENTED_EDGE ( 'NONE', *, *, #2608, .T. ) ;
#13859=AXIS2_PLACEMENT_3D ( 'NONE', #12172, #1690, #11020 ) ;
#13866=ORIENTED_EDGE ( 'NONE', *, *, #936, .F. ) ;
#13868=ORIENTED_EDGE ( 'NONE', *, *, #9359, .T. ) ;
#13869=ADVANCED_FACE ( 'NONE', ( #8864 ), #13695, .F. ) ;
#13871=ORIENTED_EDGE ( 'NONE', *, *, #13835, .T. ) ;
#13872=DIRECTION ( 'NONE',  ( -8.018662683283439195E-16, 5.975035461963190001E-16, 1.000000000000000000 ) ) ;
#13873=ORIENTED_EDGE ( 'NONE', *, *, #14393, .T. ) ;
#13874=ORIENTED_EDGE ( 'NONE', *, *, #8645, .T. ) ;
#13876=ORIENTED_EDGE ( 'NONE', *, *, #8917, .T. ) ;
#13877=VECTOR ( 'NONE', #10235, 1000.000000000000000 ) ;
#13880=AXIS2_PLACEMENT_3D ( 'NONE', #7263, #7345, #8267 ) ;
#13881=EDGE_CURVE ( 'NONE', #14240, #11857, #5204, .T. ) ;
#13882=EDGE_CURVE ( 'NONE', #8949, #4751, #14541, .T. ) ;
#13885=LINE ( 'NONE', #8131, #2931 ) ;
#13886=CARTESIAN_POINT ( 'NONE',  ( -19.41680297924232335, -22.68108752059492517, 54.00231026484399166 ) ) ;
#13887=DIRECTION ( 'NONE',  ( -8.018662683283439195E-16, 5.975035461963190001E-16, 1.000000000000000000 ) ) ;
#13893=ORIENTED_EDGE ( 'NONE', *, *, #3136, .F. ) ;
#13894=DIRECTION ( 'NONE',  ( 0.9868311969055004740, 0.1617534816134024167, 6.946583704589977600E-16 ) ) ;
#13895=CARTESIAN_POINT ( 'NONE',  ( -15.19690733689918538, -23.47778227853769550, 56.85231026484400019 ) ) ;
#13896=CARTESIAN_POINT ( 'NONE',  ( -20.64795620320353109, -18.36032465801230273, 56.85231026484398598 ) ) ;
#13897=ORIENTED_EDGE ( 'NONE', *, *, #13137, .T. ) ;
#13901=CARTESIAN_POINT ( 'NONE',  ( -21.05979293892203330, -6.334749421441233430, 56.85231026484398598 ) ) ;
#13902=CARTESIAN_POINT ( 'NONE',  ( -22.70913108387521007, -17.14542124616560770, 56.85231026484398598 ) ) ;
#13905=LINE ( 'NONE', #4498, #6474 ) ;
#13907=ORIENTED_EDGE ( 'NONE', *, *, #14845, .F. ) ;
#13908=PLANE ( 'NONE',  #8972 ) ;
#13912=DIRECTION ( 'NONE',  ( 0.5975035461963188466, 0.8018662683283437342, 0.000000000000000000 ) ) ;
#13913=VERTEX_POINT ( 'NONE', #5647 ) ;
#13914=ORIENTED_EDGE ( 'NONE', *, *, #12435, .T. ) ;
#13916=LINE ( 'NONE', #3433, #9224 ) ;
#13917=AXIS2_PLACEMENT_3D ( 'NONE', #417, #11033, #2848 ) ;
#13919=ADVANCED_FACE ( 'NONE', ( #6787, #2294 ), #4740, .T. ) ;
#13921=FACE_OUTER_BOUND ( 'NONE', #8182, .T. ) ;
#13922=EDGE_CURVE ( 'NONE', #6446, #12986, #4663, .T. ) ;
#13923=DIRECTION ( 'NONE',  ( 0.5975035461963189576, 0.8018662683283437342, 0.000000000000000000 ) ) ;
#13925=CARTESIAN_POINT ( 'NONE',  ( -5.966797098401851684, -16.44411015522000596, 54.00231026484400587 ) ) ;
#13926=LINE ( 'NONE', #11475, #80 ) ;
#13928=DIRECTION ( 'NONE',  ( -8.018662683283439195E-16, 5.975035461963190001E-16, 1.000000000000000000 ) ) ;
#13930=DIRECTION ( 'NONE',  ( 0.9966498018049937402, -0.08178736187251965661, 8.480480961564258050E-16 ) ) ;
#13934=AXIS2_PLACEMENT_3D ( 'NONE', #3627, #6131, #10741 ) ;
#13935=DIRECTION ( 'NONE',  ( -0.5975035461963190686, -0.8018662683283436232, -2.958228394578794270E-31 ) ) ;
#13936=VERTEX_POINT ( 'NONE', #9091 ) ;
#13940=PLANE ( 'NONE',  #5982 ) ;
#13941=DIRECTION ( 'NONE',  ( -8.018662683283438208E-16, 5.975035461963189015E-16, 1.000000000000000000 ) ) ;
#13942=VERTEX_POINT ( 'NONE', #3361 ) ;
#13944=VERTEX_POINT ( 'NONE', #5726 ) ;
#13945=CARTESIAN_POINT ( 'NONE',  ( -25.43486656742120999, -12.61682438329676259, 54.00231026484397745 ) ) ;
#13946=EDGE_LOOP ( 'NONE', ( #11384, #6869, #796, #8141 ) ) ;
#13949=CARTESIAN_POINT ( 'NONE',  ( -20.60611791317904107, -19.76323582219775687, 56.85231026484398598 ) ) ;
#13951=CARTESIAN_POINT ( 'NONE',  ( -7.499849062438288527, -12.40572695854698360, 56.85231026484400019 ) ) ;
#13956=PLANE ( 'NONE',  #3514 ) ;
#13966=DIRECTION ( 'NONE',  ( -0.02283895005205794151, 0.9997391571607663341, -6.156614753256579139E-16 ) ) ;
#13967=VERTEX_POINT ( 'NONE', #5798 ) ;
#13969=ORIENTED_EDGE ( 'NONE', *, *, #12518, .T. ) ;
#13971=APPLICATION_CONTEXT ( 'automotive_design' ) ;
#13972=AXIS2_PLACEMENT_3D ( 'NONE', #3062, #10253, #14996 ) ;
#13973=LINE ( 'NONE', #8150, #8038 ) ;
#13975=DIRECTION ( 'NONE',  ( -0.8599296884906633132, 0.5104125104778984845, -9.945218953682734920E-16 ) ) ;
#13979=ORIENTED_EDGE ( 'NONE', *, *, #1407, .F. ) ;
#13984=DIRECTION ( 'NONE',  ( 0.5975035461963188466, 0.8018662683283437342, 0.000000000000000000 ) ) ;
#13985=VECTOR ( 'NONE', #8472, 1000.000000000000000 ) ;
#13990=CARTESIAN_POINT ( 'NONE',  ( -15.31527533914055539, -21.58027268651140673, 56.85231026484400019 ) ) ;
#13991=ORIENTED_EDGE ( 'NONE', *, *, #7676, .F. ) ;
#13993=DIRECTION ( 'NONE',  ( 8.018662683283438208E-16, -5.975035461963189015E-16, -1.000000000000000000 ) ) ;
#13995=SURFACE_STYLE_FILL_AREA ( #1368 ) ;
#13996=VECTOR ( 'NONE', #6743, 999.9999999999998863 ) ;
#13997=VECTOR ( 'NONE', #3768, 1000.000000000000114 ) ;
#13998=CARTESIAN_POINT ( 'NONE',  ( -17.58300953724144122, -11.95501924286632267, 51.00231026484399166 ) ) ;
#13999=DIRECTION ( 'NONE',  ( 0.5975035461963189576, 0.8018662683283437342, 0.000000000000000000 ) ) ;
#14000=DIRECTION ( 'NONE',  ( 0.9983330752162417054, 0.05771543059946734194, 7.660444431189781397E-16 ) ) ;
#14003=ORIENTED_EDGE ( 'NONE', *, *, #378, .F. ) ;
#14004=DIRECTION ( 'NONE',  ( -0.7350174335289139105, 0.6780482080269578660, -9.945218953682732947E-16 ) ) ;
#14007=VERTEX_POINT ( 'NONE', #11692 ) ;
#14009=AXIS2_PLACEMENT_3D ( 'NONE', #3600, #7023, #13025 ) ;
#14010=ADVANCED_FACE ( 'NONE', ( #3511 ), #14914, .F. ) ;
#14012=VERTEX_POINT ( 'NONE', #3291 ) ;
#14013=LINE ( 'NONE', #3686, #1935 ) ;
#14014=CARTESIAN_POINT ( 'NONE',  ( -9.031792552787408113, -10.63903015472410374, 57.00231026484399166 ) ) ;
#14015=CARTESIAN_POINT ( 'NONE',  ( -8.569834614884436874, -19.36726104528708703, 56.85231026484400019 ) ) ;
#14017=CARTESIAN_POINT ( 'NONE',  ( -11.68798435751175369, -21.74340199640734994, 56.85231026484400019 ) ) ;
#14019=DIRECTION ( 'NONE',  ( 0.5975035461963189576, 0.8018662683283437342, 0.000000000000000000 ) ) ;
#14021=EDGE_CURVE ( 'NONE', #11608, #2388, #6153, .T. ) ;
#14022=EDGE_LOOP ( 'NONE', ( #1306, #3727, #13288, #11127 ) ) ;
#14024=EDGE_CURVE ( 'NONE', #6873, #7651, #6861, .T. ) ;
#14025=EDGE_LOOP ( 'NONE', ( #8417, #6820, #10810, #3465 ) ) ;
#14026=CARTESIAN_POINT ( 'NONE',  ( -16.32407967933980686, -20.53418644068968746, 56.85231026484400019 ) ) ;
#14027=ORIENTED_EDGE ( 'NONE', *, *, #14429, .F. ) ;
#14030=EDGE_CURVE ( 'NONE', #7744, #7558, #12626, .T. ) ;
#14031=CARTESIAN_POINT ( 'NONE',  ( -15.54961651457173488, -13.51026476396819831, 56.85231026484398598 ) ) ;
#14032=VERTEX_POINT ( 'NONE', #10544 ) ;
#14033=DIRECTION ( 'NONE',  ( 8.018662683283438208E-16, -5.975035461963189015E-16, -1.000000000000000000 ) ) ;
#14034=VECTOR ( 'NONE', #4489, 1000.000000000000000 ) ;
#14035=EDGE_CURVE ( 'NONE', #9929, #2365, #14068, .T. ) ;
#14036=DIRECTION ( 'NONE',  ( -8.018662683283438208E-16, 5.975035461963189015E-16, 1.000000000000000000 ) ) ;
#14041=CARTESIAN_POINT ( 'NONE',  ( -13.92794721577312878, -5.586467200048621073, 56.85231026484398598 ) ) ;
#14042=VERTEX_POINT ( 'NONE', #8246 ) ;
#14043=CARTESIAN_POINT ( 'NONE',  ( -15.16333526000374832, -10.64029123852186487, 51.25231026484399166 ) ) ;
#14045=CARTESIAN_POINT ( 'NONE',  ( -21.67659902633305791, -21.33978230808610022, 54.00231026484399166 ) ) ;
#14047=ORIENTED_EDGE ( 'NONE', *, *, #6157, .F. ) ;
#14048=CARTESIAN_POINT ( 'NONE',  ( -7.902754534677060683, -18.47202114588016642, 56.85231026484400019 ) ) ;
#14050=LINE ( 'NONE', #6000, #4509 ) ;
#14052=VECTOR ( 'NONE', #6038, 1000.000000000000000 ) ;
#14054=EDGE_CURVE ( 'NONE', #13179, #505, #10624, .T. ) ;
#14055=CARTESIAN_POINT ( 'NONE',  ( -19.62128088291994388, -20.45131122700032833, 57.00231026484397745 ) ) ;
#14058=CARTESIAN_POINT ( 'NONE',  ( -9.299228256956212135, -8.333850033420862502, 56.85231026484398598 ) ) ;
#14063=CARTESIAN_POINT ( 'NONE',  ( -12.84854673063649599, -12.36513540471286809, 51.25231026484399166 ) ) ;
#14065=DIRECTION ( 'NONE',  ( -8.018662683283439195E-16, 5.975035461963190001E-16, 1.000000000000000000 ) ) ;
#14067=DIRECTION ( 'NONE',  ( -0.5975035461963189576, -0.8018662683283438453, 9.860761315262649757E-32 ) ) ;
#14068=LINE ( 'NONE', #8013, #3971 ) ;
#14069=ADVANCED_FACE ( 'NONE', ( #154, #2820 ), #9550, .F. ) ;
#14076=CARTESIAN_POINT ( 'NONE',  ( -15.49969986081086226, -13.50737899243826767, -13.99768973515600301 ) ) ;
#14081=ORIENTED_EDGE ( 'NONE', *, *, #5905, .T. ) ;
#14083=DIRECTION ( 'NONE',  ( 0.5975035461963188466, 0.8018662683283437342, 0.000000000000000000 ) ) ;
#14084=ORIENTED_EDGE ( 'NONE', *, *, #8456, .T. ) ;
#14085=VECTOR ( 'NONE', #11174, 999.9999999999998863 ) ;
#14086=LINE ( 'NONE', #13115, #5352 ) ;
#14087=DIRECTION ( 'NONE',  ( 8.018662683283438208E-16, -5.975035461963189015E-16, -1.000000000000000000 ) ) ;
#14088=EDGE_CURVE ( 'NONE', #10261, #12780, #1289, .T. ) ;
#14091=CARTESIAN_POINT ( 'NONE',  ( -16.57334897777262483, -22.01522992987520766, 57.00231026484399166 ) ) ;
#14096=ORIENTED_EDGE ( 'NONE', *, *, #13765, .T. ) ;
#14104=LINE ( 'NONE', #9588, #10069 ) ;
#14108=CARTESIAN_POINT ( 'NONE',  ( -16.58746603607634640, -23.42289157363888208, 57.00231026484399166 ) ) ;
#14113=CARTESIAN_POINT ( 'NONE',  ( -12.51218212982926836, -9.498047650796548780, -13.49768973515600301 ) ) ;
#14116=DIRECTION ( 'NONE',  ( 0.8719950447285823580, 0.4895147004624046394, 4.067366430758000189E-16 ) ) ;
#14123=VERTEX_POINT ( 'NONE', #10924 ) ;
#14124=EDGE_CURVE ( 'NONE', #11072, #6628, #14444, .T. ) ;
#14128=AXIS2_PLACEMENT_3D ( 'NONE', #10164, #13553, #12400 ) ;
#14129=CARTESIAN_POINT ( 'NONE',  ( -20.19618812003464470, -21.27295997720514720, 56.85231026484398598 ) ) ;
#14132=CARTESIAN_POINT ( 'NONE',  ( -21.60512016940287694, -5.619130273271677467, 56.85231026484398598 ) ) ;
#14137=ORIENTED_EDGE ( 'NONE', *, *, #6229, .F. ) ;
#14138=VECTOR ( 'NONE', #5227, 999.9999999999998863 ) ;
#14139=FACE_OUTER_BOUND ( 'NONE', #2229, .T. ) ;
#14140=EDGE_LOOP ( 'NONE', ( #4979, #343, #5088, #8057 ) ) ;
#14142=FACE_OUTER_BOUND ( 'NONE', #12408, .T. ) ;
#14146=DIRECTION ( 'NONE',  ( 8.018662683283438208E-16, -5.975035461963189015E-16, -1.000000000000000000 ) ) ;
#14147=CARTESIAN_POINT ( 'NONE',  ( -15.49969986081091733, -13.50737899243822682, 54.00231026484399166 ) ) ;
#14149=FILL_AREA_STYLE_COLOUR ( '', #124 ) ;
#14150=AXIS2_PLACEMENT_3D ( 'NONE', #5640, #10312, #13912 ) ;
#14151=CARTESIAN_POINT ( 'NONE',  ( -15.49969986081086226, -13.50737899243826767, -13.99768973515600301 ) ) ;
#14156=DIRECTION ( 'NONE',  ( -8.018662683283438208E-16, 5.975035461963189015E-16, 1.000000000000000000 ) ) ;
#14157=ORIENTED_EDGE ( 'NONE', *, *, #11079, .T. ) ;
#14158=CARTESIAN_POINT ( 'NONE',  ( -6.405625242116718354, -17.60596799715946759, 57.00231026484399166 ) ) ;
#14160=VECTOR ( 'NONE', #1783, 1000.000000000000000 ) ;
#14163=ORIENTED_EDGE ( 'NONE', *, *, #14611, .F. ) ;
#14164=VERTEX_POINT ( 'NONE', #6017 ) ;
#14165=VECTOR ( 'NONE', #10299, 1000.000000000000114 ) ;
#14166=EDGE_CURVE ( 'NONE', #2405, #4751, #10700, .T. ) ;
#14167=DIRECTION ( 'NONE',  ( 8.018662683283438208E-16, -5.975035461963189015E-16, -1.000000000000000000 ) ) ;
#14168=ORIENTED_EDGE ( 'NONE', *, *, #11594, .T. ) ;
#14170=CARTESIAN_POINT ( 'NONE',  ( -13.09722856071139496, -21.21670818843173478, 56.85231026484400019 ) ) ;
#14171=CARTESIAN_POINT ( 'NONE',  ( -6.309378268457432881, -9.629413800598410234, 54.00231026484399166 ) ) ;
#14176=AXIS2_PLACEMENT_3D ( 'NONE', #7729, #711, #9815 ) ;
#14177=ORIENTED_EDGE ( 'NONE', *, *, #9802, .F. ) ;
#14179=EDGE_LOOP ( 'NONE', ( #2475, #224, #3639, #6225 ) ) ;
#14181=CARTESIAN_POINT ( 'NONE',  ( -10.85342163307452523, -20.71489927548028476, 57.00231026484399166 ) ) ;
#14182=ORIENTED_EDGE ( 'NONE', *, *, #5549, .T. ) ;
#14186=VECTOR ( 'NONE', #8266, 1000.000000000000114 ) ;
#14191=CARTESIAN_POINT ( 'NONE',  ( -17.47506273705024071, -21.33739760717825718, 57.00231026484399166 ) ) ;
#14192=CARTESIAN_POINT ( 'NONE',  ( -19.41680297924232690, -22.68108752059492517, 56.85231026484400019 ) ) ;
#14193=VERTEX_POINT ( 'NONE', #4970 ) ;
#14195=DIRECTION ( 'NONE',  ( 0.6251242923673516749, 0.7805252200231699300, 3.489949670249872777E-17 ) ) ;
#14199=DIRECTION ( 'NONE',  ( 0.9966498018049937402, -0.08178736187251965661, 8.480480961564258050E-16 ) ) ;
#14201=DIRECTION ( 'NONE',  ( 0.5975035461963189576, 0.8018662683283437342, 0.000000000000000000 ) ) ;
#14203=FACE_OUTER_BOUND ( 'NONE', #14926, .T. ) ;
#14205=CARTESIAN_POINT ( 'NONE',  ( -12.51218212982926836, -9.498047650796547003, -13.99768973515600301 ) ) ;
#14206=CARTESIAN_POINT ( 'NONE',  ( -20.48903913017556633, -19.85700446605285308, 57.00231026484397745 ) ) ;
#14207=EDGE_LOOP ( 'NONE', ( #7047, #14695, #10887, #127 ) ) ;
#14209=CARTESIAN_POINT ( 'NONE',  ( -7.223083447440863836, -17.23012942000294245, 56.85231026484400019 ) ) ;
#14210=ORIENTED_EDGE ( 'NONE', *, *, #8868, .T. ) ;
#14211=ADVANCED_FACE ( 'NONE', ( #457 ), #12082, .T. ) ;
#14212=DIRECTION ( 'NONE',  ( -8.018662683283438208E-16, 5.975035461963189015E-16, 1.000000000000000000 ) ) ;
#14215=ORIENTED_EDGE ( 'NONE', *, *, #3515, .T. ) ;
#14217=VERTEX_POINT ( 'NONE', #13455 ) ;
#14219=ADVANCED_FACE ( 'NONE', ( #523 ), #4266, .F. ) ;
#14223=FACE_OUTER_BOUND ( 'NONE', #13796, .T. ) ;
#14225=CARTESIAN_POINT ( 'NONE',  ( -12.51218212982932165, -9.498047650796509700, 51.00031026484398922 ) ) ;
#14226=VECTOR ( 'NONE', #1330, 1000.000000000000000 ) ;
#14227=CIRCLE ( 'NONE', #7619, 4.500000000000000000 ) ;
#14229=CARTESIAN_POINT ( 'NONE',  ( -18.61476135779618346, -20.95734656753543845, 57.00231026484397745 ) ) ;
#14230=ORIENTED_EDGE ( 'NONE', *, *, #10869, .T. ) ;
#14233=PLANE ( 'NONE',  #10084 ) ;
#14234=ORIENTED_EDGE ( 'NONE', *, *, #7282, .T. ) ;
#14235=LINE ( 'NONE', #5734, #4199 ) ;
#14236=EDGE_CURVE ( 'NONE', #11873, #6817, #13602, .T. ) ;
#14238=EDGE_LOOP ( 'NONE', ( #2732, #4470, #13322, #5105 ) ) ;
#14240=VERTEX_POINT ( 'NONE', #2888 ) ;
#14241=ORIENTED_EDGE ( 'NONE', *, *, #11245, .T. ) ;
#14242=LINE ( 'NONE', #5965, #7513 ) ;
#14244=VECTOR ( 'NONE', #6190, 1000.000000000000000 ) ;
#14245=AXIS2_PLACEMENT_3D ( 'NONE', #8723, #2991, #8874 ) ;
#14246=CARTESIAN_POINT ( 'NONE',  ( -18.48721759179245439, -17.51671033407998479, -13.49768973515600301 ) ) ;
#14247=FACE_OUTER_BOUND ( 'NONE', #10173, .T. ) ;
#14249=PRODUCT_DEFINITION ( 'UNKNOWN', '', #9259, #12794 ) ;
#14250=FACE_OUTER_BOUND ( 'NONE', #9850, .T. ) ;
#14252=VECTOR ( 'NONE', #10940, 1000.000000000000000 ) ;
#14253=DIRECTION ( 'NONE',  ( 0.3956847857120158740, -0.9183863840214728791, 0.000000000000000000 ) ) ;
#14254=CARTESIAN_POINT ( 'NONE',  ( -25.24719169991952583, -11.38911842147176756, 56.85231026484398598 ) ) ;
#14255=ORIENTED_EDGE ( 'NONE', *, *, #5564, .T. ) ;
#14256=ORIENTED_EDGE ( 'NONE', *, *, #12346, .T. ) ;
#14258=CARTESIAN_POINT ( 'NONE',  ( -6.507973901336479017, -12.27851192488648024, 56.85231026484400019 ) ) ;
#14260=CARTESIAN_POINT ( 'NONE',  ( -7.711221940648826489, -11.37542292179617753, 56.85231026484400019 ) ) ;
#14262=VECTOR ( 'NONE', #12299, 1000.000000000000114 ) ;
#14263=DIRECTION ( 'NONE',  ( 0.5975035461963188466, 0.8018662683283438453, 0.000000000000000000 ) ) ;
#14265=VECTOR ( 'NONE', #12135, 999.9999999999998863 ) ;
#14271=DIRECTION ( 'NONE',  ( 0.09252159378508259535, -0.9957106782009863544, 6.691306063588661357E-16 ) ) ;
#14272=CARTESIAN_POINT ( 'NONE',  ( -6.517576446443361426, -14.80457171870128974, 57.00231026484399166 ) ) ;
#14274=VERTEX_POINT ( 'NONE', #14523 ) ;
#14275=FACE_OUTER_BOUND ( 'NONE', #801, .T. ) ;
#14276=LINE ( 'NONE', #3793, #8103 ) ;
#14279=VECTOR ( 'NONE', #6064, 1000.000000000000114 ) ;
#14280=DIRECTION ( 'NONE',  ( 0.5975035461963188466, 0.8018662683283437342, 0.000000000000000000 ) ) ;
#14281=VECTOR ( 'NONE', #14823, 1000.000000000000000 ) ;
#14282=EDGE_CURVE ( 'NONE', #1866, #2020, #7692, .T. ) ;
#14285=DIRECTION ( 'NONE',  ( 0.5401126942952622079, 0.8415927028326187775, -6.975647374412502487E-17 ) ) ;
#14287=ORIENTED_EDGE ( 'NONE', *, *, #10761, .F. ) ;
#14290=EDGE_LOOP ( 'NONE', ( #7105, #2169, #1849, #3574 ) ) ;
#14296=DIRECTION ( 'NONE',  ( -8.018662683283438208E-16, 5.975035461963189015E-16, 1.000000000000000000 ) ) ;
#14297=VECTOR ( 'NONE', #7788, 1000.000000000000000 ) ;
#14298=PLANE ( 'NONE',  #15026 ) ;
#14299=DIRECTION ( 'NONE',  ( -0.9183863840214729901, -0.3956847857120157075, -4.999999999999999402E-16 ) ) ;
#14301=CARTESIAN_POINT ( 'NONE',  ( -23.55378106252664239, -12.92169478045303066, 57.00231026484397745 ) ) ;
#14302=EDGE_CURVE ( 'NONE', #14910, #150, #14411, .T. ) ;
#14303=DIRECTION ( 'NONE',  ( -8.018662683283438208E-16, 5.975035461963189015E-16, 1.000000000000000000 ) ) ;
#14310=CARTESIAN_POINT ( 'NONE',  ( -18.93133274217424855, -21.90887563098697655, 57.00231026484399166 ) ) ;
#14312=DIRECTION ( 'NONE',  ( -8.018662683283439195E-16, 5.975035461963190001E-16, 1.000000000000000000 ) ) ;
#14316=DIRECTION ( 'NONE',  ( 0.05771543059946734194, -0.9983330752162417054, 6.427876096865391919E-16 ) ) ;
#14317=DIRECTION ( 'NONE',  ( 0.5975035461963188466, 0.8018662683283437342, 0.000000000000000000 ) ) ;
#14318=LINE ( 'NONE', #9937, #5259 ) ;
#14319=AXIS2_PLACEMENT_3D ( 'NONE', #12991, #212, #13221 ) ;
#14320=EDGE_CURVE ( 'NONE', #14012, #7355, #1739, .T. ) ;
#14321=LINE ( 'NONE', #1236, #2216 ) ;
#14323=ADVANCED_FACE ( 'NONE', ( #600 ), #668, .T. ) ;
#14325=DIRECTION ( 'NONE',  ( -0.5975035461963187355, -0.8018662683283439563, 0.000000000000000000 ) ) ;
#14329=AXIS2_PLACEMENT_3D ( 'NONE', #12789, #4667, #13999 ) ;
#14331=ORIENTED_EDGE ( 'NONE', *, *, #4, .T. ) ;
#14332=ORIENTED_EDGE ( 'NONE', *, *, #14916, .F. ) ;
#14333=CARTESIAN_POINT ( 'NONE',  ( -10.11292913755864475, -19.52351987967747959, 57.00231026484399166 ) ) ;
#14334=ORIENTED_EDGE ( 'NONE', *, *, #378, .T. ) ;
#14336=CARTESIAN_POINT ( 'NONE',  ( -15.49969986081092088, -13.50737899243822504, 56.85231026484398598 ) ) ;
#14340=CIRCLE ( 'NONE', #7970, 9.974999999999999645 ) ;
#14342=AXIS2_PLACEMENT_3D ( 'NONE', #8352, #11801, #3065 ) ;
#14345=ORIENTED_EDGE ( 'NONE', *, *, #5030, .T. ) ;
#14346=LINE ( 'NONE', #1186, #3126 ) ;
#14353=ORIENTED_EDGE ( 'NONE', *, *, #1666, .T. ) ;
#14360=VECTOR ( 'NONE', #8704, 1000.000000000000000 ) ;
#14364=ORIENTED_EDGE ( 'NONE', *, *, #5321, .T. ) ;
#14365=DIRECTION ( 'NONE',  ( 0.5975035461963189576, 0.8018662683283437342, 0.000000000000000000 ) ) ;
#14366=DIRECTION ( 'NONE',  ( 0.5975035461963189576, 0.8018662683283437342, 0.000000000000000000 ) ) ;
#14368=LINE ( 'NONE', #2586, #14887 ) ;
#14371=DIRECTION ( 'NONE',  ( 0.6251242923673534513, 0.7805252200231685977, 3.489949670250099574E-17 ) ) ;
#14373=ADVANCED_FACE ( 'NONE', ( #8069 ), #3272, .F. ) ;
#14374=VECTOR ( 'NONE', #5051, 1000.000000000000000 ) ;
#14375=VECTOR ( 'NONE', #6139, 1000.000000000000114 ) ;
#14380=CARTESIAN_POINT ( 'NONE',  ( -6.540243082598547808, -14.95284924095401458, 57.00231026484399166 ) ) ;
#14384=ORIENTED_EDGE ( 'NONE', *, *, #7187, .F. ) ;
#14385=LINE ( 'NONE', #14310, #3466 ) ;
#14386=ORIENTED_EDGE ( 'NONE', *, *, #8312, .F. ) ;
#14387=CARTESIAN_POINT ( 'NONE',  ( -8.744338604334316756, -15.61126689213601360, 56.85231026484400019 ) ) ;
#14388=VERTEX_POINT ( 'NONE', #5552 ) ;
#14393=EDGE_CURVE ( 'NONE', #13485, #11236, #14897, .T. ) ;
#14394=DIRECTION ( 'NONE',  ( -0.6601155939154559338, 0.7511640317997426708, -9.781476007338054812E-16 ) ) ;
#14397=PLANE ( 'NONE',  #13640 ) ;
#14398=VECTOR ( 'NONE', #12851, 1000.000000000000227 ) ;
#14399=LINE ( 'NONE', #11681, #8721 ) ;
#14400=DIRECTION ( 'NONE',  ( -8.018662683283438208E-16, 5.975035461963189015E-16, 1.000000000000000000 ) ) ;
#14403=CARTESIAN_POINT ( 'NONE',  ( -7.307539508764906877, -16.04208977798462854, 57.00231026484399166 ) ) ;
#14404=ORIENTED_EDGE ( 'NONE', *, *, #7834, .T. ) ;
#14405=ORIENTED_EDGE ( 'NONE', *, *, #4454, .T. ) ;
#14407=FACE_OUTER_BOUND ( 'NONE', #12054, .T. ) ;
#14410=DIRECTION ( 'NONE',  ( -0.1165201156931293391, -0.9931883319083343320, 4.999999999999998416E-16 ) ) ;
#14411=CIRCLE ( 'NONE', #9764, 9.974999999999999645 ) ;
#14413=DIRECTION ( 'NONE',  ( 0.9472588896649083434, -0.3204693369899919708, 9.510565162951537596E-16 ) ) ;
#14415=DIRECTION ( 'NONE',  ( 0.9988970074402869770, -0.04695496274984588270, 8.290375725550417844E-16 ) ) ;
#14417=ORIENTED_EDGE ( 'NONE', *, *, #7017, .F. ) ;
#14419=ORIENTED_EDGE ( 'NONE', *, *, #354, .T. ) ;
#14420=DIRECTION ( 'NONE',  ( -0.9183863840214729901, -0.3956847857120157075, -4.999999999999999402E-16 ) ) ;
#14424=DIRECTION ( 'NONE',  ( -0.6251242923673536733, -0.7805252200231682647, -3.489949670250128540E-17 ) ) ;
#14427=LINE ( 'NONE', #13295, #2199 ) ;
#14428=DIRECTION ( 'NONE',  ( 8.018662683283438208E-16, -5.975035461963189015E-16, -1.000000000000000000 ) ) ;
#14429=EDGE_CURVE ( 'NONE', #2863, #11333, #5630, .T. ) ;
#14430=DIRECTION ( 'NONE',  ( -0.7032868978765995926, -0.7109061395677416240, -1.391731009600651544E-16 ) ) ;
#14431=DIRECTION ( 'NONE',  ( -8.018662683283438208E-16, 5.975035461963189015E-16, 1.000000000000000000 ) ) ;
#14432=ORIENTED_EDGE ( 'NONE', *, *, #12487, .F. ) ;
#14433=DIRECTION ( 'NONE',  ( 0.9183863840214729901, 0.3956847857120157075, 5.000000000000000389E-16 ) ) ;
#14434=PLANE ( 'NONE',  #12889 ) ;
#14439=ORIENTED_EDGE ( 'NONE', *, *, #8012, .F. ) ;
#14442=CARTESIAN_POINT ( 'NONE',  ( -11.71495923925436955, -5.812446346369147143, 57.00231026484397745 ) ) ;
#14443=CIRCLE ( 'NONE', #14930, 9.974999999999999645 ) ;
#14444=LINE ( 'NONE', #4897, #5189 ) ;
#14446=EDGE_CURVE ( 'NONE', #8466, #8073, #976, .T. ) ;
#14449=ORIENTED_EDGE ( 'NONE', *, *, #6252, .F. ) ;
#14453=VECTOR ( 'NONE', #791, 1000.000000000000227 ) ;
#14457=ORIENTED_EDGE ( 'NONE', *, *, #12824, .F. ) ;
#14458=ORIENTED_EDGE ( 'NONE', *, *, #4190, .T. ) ;
#14459=DIRECTION ( 'NONE',  ( -0.9354976265738682573, 0.3533329742249642913, -9.612616959383187437E-16 ) ) ;
#14460=LINE ( 'NONE', #401, #2667 ) ;
#14461=VECTOR ( 'NONE', #2404, 1000.000000000000000 ) ;
#14464=CARTESIAN_POINT ( 'NONE',  ( -15.49969986081092088, -13.50737899243822504, 57.00231026484397745 ) ) ;
#14468=EDGE_CURVE ( 'NONE', #6205, #11933, #13973, .T. ) ;
#14469=CIRCLE ( 'NONE', #13261, 9.974999999999999645 ) ;
#14470=ORIENTED_EDGE ( 'NONE', *, *, #9314, .T. ) ;
#14473=ORIENTED_EDGE ( 'NONE', *, *, #3928, .T. ) ;
#14477=AXIS2_PLACEMENT_3D ( 'NONE', #10292, #10216, #3187 ) ;
#14478=VECTOR ( 'NONE', #5614, 999.9999999999998863 ) ;
#14480=EDGE_LOOP ( 'NONE', ( #13482, #1169, #12136, #2585 ) ) ;
#14481=CARTESIAN_POINT ( 'NONE',  ( -7.734307812155742923, -7.246443652516327383, 56.85231026484400019 ) ) ;
#14482=CARTESIAN_POINT ( 'NONE',  ( -20.06719866676104402, -21.34952185377683165, 56.85231026484398598 ) ) ;
#14483=DIRECTION ( 'NONE',  ( 0.2640193276337003403, -0.9645173894937555392, 7.880107536067285830E-16 ) ) ;
#14484=VECTOR ( 'NONE', #12740, 1000.000000000000000 ) ;
#14485=VECTOR ( 'NONE', #2014, 1000.000000000000114 ) ;
#14489=CARTESIAN_POINT ( 'NONE',  ( -23.68291657637574588, -19.21137664199072148, 56.85231026484398598 ) ) ;
#14490=EDGE_CURVE ( 'NONE', #6732, #4531, #15042, .T. ) ;
#14491=VERTEX_POINT ( 'NONE', #1120 ) ;
#14494=EDGE_LOOP ( 'NONE', ( #1017, #13914, #2435, #5896 ) ) ;
#14495=VERTEX_POINT ( 'NONE', #10453 ) ;
#14496=LINE ( 'NONE', #3943, #10064 ) ;
#14498=ORIENTED_EDGE ( 'NONE', *, *, #1134, .T. ) ;
#14499=EDGE_CURVE ( 'NONE', #2398, #11181, #15116, .T. ) ;
#14502=CIRCLE ( 'NONE', #12297, 9.974999999999999645 ) ;
#14503=VECTOR ( 'NONE', #6308, 1000.000000000000000 ) ;
#14509=ADVANCED_FACE ( 'NONE', ( #8533 ), #4878, .T. ) ;
#14510=VECTOR ( 'NONE', #8766, 1000.000000000000114 ) ;
#14511=FACE_OUTER_BOUND ( 'NONE', #2610, .T. ) ;
#14512=ORIENTED_EDGE ( 'NONE', *, *, #12043, .T. ) ;
#14513=LINE ( 'NONE', #10054, #3851 ) ;
#14514=DIRECTION ( 'NONE',  ( 8.018662683283438208E-16, -5.975035461963189015E-16, -1.000000000000000000 ) ) ;
#14515=ORIENTED_EDGE ( 'NONE', *, *, #4397, .T. ) ;
#14518=ORIENTED_EDGE ( 'NONE', *, *, #4624, .F. ) ;
#14520=CIRCLE ( 'NONE', #9631, 9.974999999999999645 ) ;
#14523=CARTESIAN_POINT ( 'NONE',  ( -13.16883223745437448, -21.23902216335526916, 56.85231026484400019 ) ) ;
#14525=VECTOR ( 'NONE', #1254, 1000.000000000000000 ) ;
#14526=DIRECTION ( 'NONE',  ( -8.018662683283438208E-16, 5.975035461963189015E-16, 1.000000000000000000 ) ) ;
#14529=DIRECTION ( 'NONE',  ( 8.018662683283438208E-16, -5.975035461963189015E-16, -1.000000000000000000 ) ) ;
#14530=CARTESIAN_POINT ( 'NONE',  ( -9.328067836852527606, -18.71527762440592468, 57.00231026484399166 ) ) ;
#14531=VECTOR ( 'NONE', #1722, 1000.000000000000114 ) ;
#14533=VERTEX_POINT ( 'NONE', #8376 ) ;
#14535=EDGE_LOOP ( 'NONE', ( #5481, #13856, #2501, #5585 ) ) ;
#14536=ORIENTED_EDGE ( 'NONE', *, *, #9534, .F. ) ;
#14537=LINE ( 'NONE', #2686, #14244 ) ;
#14541=LINE ( 'NONE', #4058, #6639 ) ;
#14543=AXIS2_PLACEMENT_3D ( 'NONE', #785, #14706, #8957 ) ;
#14544=LINE ( 'NONE', #5355, #6108 ) ;
#14548=EDGE_LOOP ( 'NONE', ( #3747, #11720, #5938, #13578 ) ) ;
#14550=ORIENTED_EDGE ( 'NONE', *, *, #7938, .F. ) ;
#14551=CARTESIAN_POINT ( 'NONE',  ( -20.00744539586189319, -5.630737564061013778, 57.00231026484397745 ) ) ;
#14554=VERTEX_POINT ( 'NONE', #5101 ) ;
#14555=CARTESIAN_POINT ( 'NONE',  ( -14.26755283655060680, -21.48817241857114269, 57.00231026484399166 ) ) ;
#14556=ORIENTED_EDGE ( 'NONE', *, *, #5314, .F. ) ;
#14558=ADVANCED_FACE ( 'NONE', ( #3569 ), #9608, .F. ) ;
#14559=CARTESIAN_POINT ( 'NONE',  ( -15.49969986081092088, -13.50737899243822504, 57.00231026484397745 ) ) ;
#14561=VECTOR ( 'NONE', #9859, 1000.000000000000000 ) ;
#14562=CARTESIAN_POINT ( 'NONE',  ( -14.19354049678269192, -21.47604090745013750, 56.85231026484400019 ) ) ;
#14564=VERTEX_POINT ( 'NONE', #2576 ) ;
#14568=ORIENTED_EDGE ( 'NONE', *, *, #97, .T. ) ;
#14572=ORIENTED_EDGE ( 'NONE', *, *, #7898, .T. ) ;
#14580=CARTESIAN_POINT ( 'NONE',  ( -25.29546517631142777, -15.38982603914036318, 54.00231026484397745 ) ) ;
#14581=CARTESIAN_POINT ( 'NONE',  ( -10.96544185377836911, -6.825182173602284408, 56.85231026484398598 ) ) ;
#14582=ORIENTED_EDGE ( 'NONE', *, *, #3646, .T. ) ;
#14586=EDGE_LOOP ( 'NONE', ( #13873, #2226, #11842, #10992 ) ) ;
#14588=LINE ( 'NONE', #14666, #14510 ) ;
#14589=EDGE_LOOP ( 'NONE', ( #3412, #5213, #8136, #14439 ) ) ;
#14590=AXIS2_PLACEMENT_3D ( 'NONE', #8044, #32, #9354 ) ;
#14593=EDGE_CURVE ( 'NONE', #5527, #1243, #2917, .T. ) ;
#14595=VECTOR ( 'NONE', #9862, 1000.000000000000000 ) ;
#14596=CARTESIAN_POINT ( 'NONE',  ( -10.39628701978575975, -6.002951807498697612, 56.85231026484398598 ) ) ;
#14597=VECTOR ( 'NONE', #2871, 1000.000000000000000 ) ;
#14598=DIRECTION ( 'NONE',  ( 8.018662683283438208E-16, -5.975035461963189015E-16, -1.000000000000000000 ) ) ;
#14599=DIRECTION ( 'NONE',  ( -0.9085715390340232123, 0.4177292884839972631, -9.781476007338056784E-16 ) ) ;
#14602=CARTESIAN_POINT ( 'NONE',  ( -15.49969986081092088, -13.50737899243822504, 56.85231026484398598 ) ) ;
#14604=VECTOR ( 'NONE', #9825, 1000.000000000000227 ) ;
#14608=ORIENTED_EDGE ( 'NONE', *, *, #6440, .T. ) ;
#14609=FACE_OUTER_BOUND ( 'NONE', #14480, .T. ) ;
#14610=ORIENTED_EDGE ( 'NONE', *, *, #2051, .T. ) ;
#14611=EDGE_CURVE ( 'NONE', #2532, #8256, #1215, .T. ) ;
#14613=CARTESIAN_POINT ( 'NONE',  ( -6.766506000727597225, -11.03906478995046214, 56.85231026484400019 ) ) ;
#14615=VECTOR ( 'NONE', #10552, 1000.000000000000000 ) ;
#14616=CARTESIAN_POINT ( 'NONE',  ( -23.49646891012291050, -9.216349422280851300, 56.85231026484398598 ) ) ;
#14618=ADVANCED_FACE ( 'NONE', ( #11986 ), #1352, .F. ) ;
#14621=DIRECTION ( 'NONE',  ( 0.5975035461963189576, 0.8018662683283437342, 0.000000000000000000 ) ) ;
#14625=EDGE_LOOP ( 'NONE', ( #9460, #2451, #3717, #165 ) ) ;
#14626=ORIENTED_EDGE ( 'NONE', *, *, #12893, .T. ) ;
#14628=CARTESIAN_POINT ( 'NONE',  ( -19.38713143869018296, -6.429305403720261936, 57.00231026484397745 ) ) ;
#14629=CARTESIAN_POINT ( 'NONE',  ( -10.85342163307452523, -20.71489927548028476, 56.85231026484400019 ) ) ;
#14631=LINE ( 'NONE', #10891, #14160 ) ;
#14632=DIRECTION ( 'NONE',  ( 8.018662683283438208E-16, -5.975035461963189015E-16, -1.000000000000000000 ) ) ;
#14633=CARTESIAN_POINT ( 'NONE',  ( -13.85656510877104353, -11.30224675453528072, 56.75231026484397745 ) ) ;
#14637=DIRECTION ( 'NONE',  ( -8.018662683283438208E-16, 5.975035461963189015E-16, 1.000000000000000000 ) ) ;
#14641=ORIENTED_EDGE ( 'NONE', *, *, #11730, .T. ) ;
#14644=ORIENTED_EDGE ( 'NONE', *, *, #13882, .F. ) ;
#14645=ORIENTED_EDGE ( 'NONE', *, *, #11931, .T. ) ;
#14649=VECTOR ( 'NONE', #6694, 1000.000000000000227 ) ;
#14650=DIRECTION ( 'NONE',  ( -8.018662683283438208E-16, 5.975035461963189015E-16, 1.000000000000000000 ) ) ;
#14652=DIRECTION ( 'NONE',  ( -8.018662683283438208E-16, 5.975035461963189015E-16, 1.000000000000000000 ) ) ;
#14655=DIRECTION ( 'NONE',  ( -0.9988970074402869770, 0.04695496274984588270, -8.290375725550417844E-16 ) ) ;
#14656=ADVANCED_FACE ( 'NONE', ( #4172 ), #731, .T. ) ;
#14657=CARTESIAN_POINT ( 'NONE',  ( -13.01672903104007872, -13.79867928167105440, 51.25231026484399166 ) ) ;
#14658=ORIENTED_EDGE ( 'NONE', *, *, #14030, .T. ) ;
#14660=LINE ( 'NONE', #6381, #9497 ) ;
#14661=VERTEX_POINT ( 'NONE', #9907 ) ;
#14662=DIRECTION ( 'NONE',  ( 8.018662683283438208E-16, -5.975035461963189015E-16, -1.000000000000000000 ) ) ;
#14665=DIRECTION ( 'NONE',  ( 0.8543800322332385511, 0.5196486895212286683, 3.746065934159130275E-16 ) ) ;
#14666=CARTESIAN_POINT ( 'NONE',  ( -23.37741044072812713, -11.73331557219068877, 56.85231026484398598 ) ) ;
#14667=ORIENTED_EDGE ( 'NONE', *, *, #1617, .F. ) ;
#14669=DIRECTION ( 'NONE',  ( 0.8160499452489514693, 0.5779813897169900905, 3.090169943749478258E-16 ) ) ;
#14672=VECTOR ( 'NONE', #6953, 1000.000000000000000 ) ;
#14673=PLANE ( 'NONE',  #6959 ) ;
#14675=CARTESIAN_POINT ( 'NONE',  ( -21.79090396836353705, -19.33464257641254136, 56.85231026484398598 ) ) ;
#14678=EDGE_CURVE ( 'NONE', #3877, #2114, #12434, .T. ) ;
#14680=ADVANCED_FACE ( 'NONE', ( #12209 ), #1806, .F. ) ;
#14681=ORIENTED_EDGE ( 'NONE', *, *, #2454, .F. ) ;
#14685=PLANE ( 'NONE',  #5336 ) ;
#14689=PLANE ( 'NONE',  #2615 ) ;
#14691=EDGE_CURVE ( 'NONE', #9086, #532, #8906, .T. ) ;
#14692=CARTESIAN_POINT ( 'NONE',  ( -20.94048570341206883, -6.243833066724571168, 56.85231026484398598 ) ) ;
#14693=PLANE ( 'NONE',  #12786 ) ;
#14695=ORIENTED_EDGE ( 'NONE', *, *, #14799, .T. ) ;
#14696=FACE_OUTER_BOUND ( 'NONE', #6142, .T. ) ;
#14701=DIRECTION ( 'NONE',  ( -0.2536112499260171349, -0.9673062255102895524, 3.746065934159117949E-16 ) ) ;
#14704=AXIS2_PLACEMENT_3D ( 'NONE', #8896, #7738, #2094 ) ;
#14705=DIRECTION ( 'NONE',  ( -0.3956847857120157075, 0.9183863840214729901, -8.660254037844388394E-16 ) ) ;
#14706=DIRECTION ( 'NONE',  ( 0.9547156899063180546, 0.2975196656470009415, 5.877852522924732759E-16 ) ) ;
#14708=EDGE_CURVE ( 'NONE', #14274, #10935, #14427, .T. ) ;
#14711=VECTOR ( 'NONE', #1498, 1000.000000000000114 ) ;
#14715=VECTOR ( 'NONE', #1759, 1000.000000000000000 ) ;
#14717=ORIENTED_EDGE ( 'NONE', *, *, #13036, .T. ) ;
#14719=CARTESIAN_POINT ( 'NONE',  ( -23.42445533997705454, -9.084766574938008432, 56.85231026484398598 ) ) ;
#14725=AXIS2_PLACEMENT_3D ( 'NONE', #12890, #7048, #11727 ) ;
#14727=AXIS2_PLACEMENT_3D ( 'NONE', #10034, #7735, #12422 ) ;
#14728=CARTESIAN_POINT ( 'NONE',  ( -20.52642601085533869, -22.12321610861327770, 56.85231026484398598 ) ) ;
#14733=DIRECTION ( 'NONE',  ( 0.2536112499260171349, 0.9673062255102895524, -3.746065934159117949E-16 ) ) ;
#14736=PLANE ( 'NONE',  #10223 ) ;
#14738=CARTESIAN_POINT ( 'NONE',  ( -14.11952815701478059, -21.46390939632912875, 56.85231026484400019 ) ) ;
#14740=AXIS2_PLACEMENT_3D ( 'NONE', #4499, #7070, #3345 ) ;
#14741=CARTESIAN_POINT ( 'NONE',  ( -21.60512016940287339, -5.619130273271679243, 54.00231026484397745 ) ) ;
#14744=FACE_OUTER_BOUND ( 'NONE', #13946, .T. ) ;
#14745=EDGE_CURVE ( 'NONE', #5367, #6300, #8678, .T. ) ;
#14746=DIRECTION ( 'NONE',  ( -0.9983330752162417054, -0.05771543059946733500, -7.660444431189781397E-16 ) ) ;
#14748=AXIS2_PLACEMENT_3D ( 'NONE', #11541, #1061, #5720 ) ;
#14751=FACE_OUTER_BOUND ( 'NONE', #9375, .T. ) ;
#14752=DIRECTION ( 'NONE',  ( -0.5104125104778984845, -0.8599296884906632021, 1.045284632676530333E-16 ) ) ;
#14755=CARTESIAN_POINT ( 'NONE',  ( -12.23206416678372932, -4.082773856353237640, 56.85231026484398598 ) ) ;
#14756=VECTOR ( 'NONE', #9006, 1000.000000000000227 ) ;
#14759=ORIENTED_EDGE ( 'NONE', *, *, #12561, .T. ) ;
#14760=ORIENTED_EDGE ( 'NONE', *, *, #2978, .T. ) ;
#14762=DIRECTION ( 'NONE',  ( -0.6251242923673533403, -0.7805252200231684867, -3.489949670250098342E-17 ) ) ;
#14764=EDGE_CURVE ( 'NONE', #5306, #14217, #3946, .T. ) ;
#14765=DIRECTION ( 'NONE',  ( -0.7953815700667045130, -0.6061090314441981430, -2.756373558170028881E-16 ) ) ;
#14768=VECTOR ( 'NONE', #12897, 1000.000000000000227 ) ;
#14771=CARTESIAN_POINT ( 'NONE',  ( -23.45327702811275827, -7.487309620431346069, 57.00231026484397745 ) ) ;
#14774=DIRECTION ( 'NONE',  ( -0.1855175943453168941, -0.9826409426582662920, 4.383711467890769768E-16 ) ) ;
#14777=ORIENTED_EDGE ( 'NONE', *, *, #5602, .T. ) ;
#14779=CARTESIAN_POINT ( 'NONE',  ( -7.425287632467987287, -13.60480674405941492, 56.85231026484400019 ) ) ;
#14780=DIRECTION ( 'NONE',  ( -8.018662683283438208E-16, 5.975035461963189015E-16, 1.000000000000000000 ) ) ;
#14781=ORIENTED_EDGE ( 'NONE', *, *, #2103, .F. ) ;
#14787=CARTESIAN_POINT ( 'NONE',  ( -24.06473463808513813, -13.92741382918746496, 57.00231026484397745 ) ) ;
#14788=CARTESIAN_POINT ( 'NONE',  ( -12.25471857405102405, -7.219983152459794162, 57.00231026484397745 ) ) ;
#14789=ORIENTED_EDGE ( 'NONE', *, *, #10546, .T. ) ;
#14792=DIRECTION ( 'NONE',  ( 0.5975035461963188466, 0.8018662683283437342, 0.000000000000000000 ) ) ;
#14793=ORIENTED_EDGE ( 'NONE', *, *, #11585, .F. ) ;
#14794=ORIENTED_EDGE ( 'NONE', *, *, #6626, .T. ) ;
#14795=FACE_OUTER_BOUND ( 'NONE', #3906, .T. ) ;
#14796=ORIENTED_EDGE ( 'NONE', *, *, #14024, .F. ) ;
#14797=DIRECTION ( 'NONE',  ( 0.1165201156931293391, 0.9931883319083343320, -4.999999999999998416E-16 ) ) ;
#14799=EDGE_CURVE ( 'NONE', #1039, #10194, #1031, .T. ) ;
#14802=CARTESIAN_POINT ( 'NONE',  ( -10.27295246487022240, -6.088325032597582620, 56.85231026484398598 ) ) ;
#14809=EDGE_CURVE ( 'NONE', #4418, #14123, #13885, .T. ) ;
#14810=ORIENTED_EDGE ( 'NONE', *, *, #55, .F. ) ;
#14811=ORIENTED_EDGE ( 'NONE', *, *, #8260, .F. ) ;
#14812=CARTESIAN_POINT ( 'NONE',  ( -22.64353467404651354, -6.545608444567306172, 57.00231026484397745 ) ) ;
#14813=EDGE_CURVE ( 'NONE', #9717, #13190, #6337, .T. ) ;
#14814=FACE_OUTER_BOUND ( 'NONE', #1676, .T. ) ;
#14821=AXIS2_PLACEMENT_3D ( 'NONE', #2297, #5869, #9244 ) ;
#14822=DIRECTION ( 'NONE',  ( 0.5975035461963188466, 0.8018662683283437342, 0.000000000000000000 ) ) ;
#14823=DIRECTION ( 'NONE',  ( 0.2301973227387160703, -0.9731439732146149879, 7.660444431189776467E-16 ) ) ;
#14826=CARTESIAN_POINT ( 'NONE',  ( -21.60512016940287694, -5.619130273271677467, 57.00231026484397745 ) ) ;
#14827=VECTOR ( 'NONE', #500, 1000.000000000000000 ) ;
#14828=EDGE_CURVE ( 'NONE', #1753, #2020, #10752, .T. ) ;
#14831=ORIENTED_EDGE ( 'NONE', *, *, #7673, .F. ) ;
#14832=ORIENTED_EDGE ( 'NONE', *, *, #391, .F. ) ;
#14833=DIRECTION ( 'NONE',  ( 0.6859287159822015090, -0.7276687409742212953, 9.848077530122081084E-16 ) ) ;
#14839=CARTESIAN_POINT ( 'NONE',  ( -12.04767799572592502, -20.80732214584531548, 57.00231026484399166 ) ) ;
#14841=AXIS2_PLACEMENT_3D ( 'NONE', #1675, #8705, #4049 ) ;
#14842=AXIS2_PLACEMENT_3D ( 'NONE', #2485, #14271, #3788 ) ;
#14844=CARTESIAN_POINT ( 'NONE',  ( -18.48721759179250412, -17.51671033407995282, 45.50231026484398456 ) ) ;
#14845=EDGE_CURVE ( 'NONE', #9275, #8949, #4476, .T. ) ;
#14846=VECTOR ( 'NONE', #6375, 1000.000000000000000 ) ;
#14849=VERTEX_POINT ( 'NONE', #3402 ) ;
#14850=CARTESIAN_POINT ( 'NONE',  ( -10.22560374232860347, -19.62253721876480128, 57.00231026484399166 ) ) ;
#14855=DIRECTION ( 'NONE',  ( 8.018662683283438208E-16, -5.975035461963189015E-16, -1.000000000000000000 ) ) ;
#14856=ORIENTED_EDGE ( 'NONE', *, *, #14691, .T. ) ;
#14860=ORIENTED_EDGE ( 'NONE', *, *, #4614, .F. ) ;
#14861=LINE ( 'NONE', #10186, #769 ) ;
#14862=AXIS2_PLACEMENT_3D ( 'NONE', #10281, #6747, #10123 ) ;
#14864=EDGE_CURVE ( 'NONE', #10177, #2863, #12960, .T. ) ;
#14867=EDGE_CURVE ( 'NONE', #8690, #10111, #11582, .T. ) ;
#14868=ORIENTED_EDGE ( 'NONE', *, *, #5821, .T. ) ;
#14870=DIRECTION ( 'NONE',  ( -0.9931883319083343320, 0.1165201156931293391, -8.660254037844386422E-16 ) ) ;
#14871=ORIENTED_EDGE ( 'NONE', *, *, #14499, .F. ) ;
#14872=ORIENTED_EDGE ( 'NONE', *, *, #2331, .T. ) ;
#14874=CARTESIAN_POINT ( 'NONE',  ( -7.264457220180047692, -15.89840986842769333, 56.85231026484400019 ) ) ;
#14875=EDGE_LOOP ( 'NONE', ( #3381, #2076, #13897, #4129 ) ) ;
#14877=( BOUNDED_CURVE ( )  B_SPLINE_CURVE ( 3, ( #5392, #7822, #8682, #13364 ),
 .UNSPECIFIED., .F., .T. ) 
 B_SPLINE_CURVE_WITH_KNOTS ( ( 4, 4 ),
 ( 4.712388980384689674, 6.283185307179585344 ),
 .UNSPECIFIED. ) 
 CURVE ( )  GEOMETRIC_REPRESENTATION_ITEM ( )  RATIONAL_B_SPLINE_CURVE ( ( 1.000000000000000000, 0.8047378541243649375, 0.8047378541243649375, 1.000000000000000000 ) ) 
 REPRESENTATION_ITEM ( '' )  );
#14878=CARTESIAN_POINT ( 'NONE',  ( -15.50552586659557797, -13.55703840903364288, 56.85231026484398598 ) ) ;
#14887=VECTOR ( 'NONE', #295, 1000.000000000000114 ) ;
#14888=DIRECTION ( 'NONE',  ( -0.8160499452489514693, -0.5779813897169900905, -3.090169943749478258E-16 ) ) ;
#14889=ORIENTED_EDGE ( 'NONE', *, *, #743, .F. ) ;
#14893=CARTESIAN_POINT ( 'NONE',  ( -18.04103863274072594, -14.60230930160663121, 51.00231026484399166 ) ) ;
#14894=CARTESIAN_POINT ( 'NONE',  ( -19.06972223273333711, -21.85101071153832919, 57.00231026484399166 ) ) ;
#14896=DIRECTION ( 'NONE',  ( 0.5975035461963190686, 0.8018662683283437342, 1.972152263052529514E-31 ) ) ;
#14897=LINE ( 'NONE', #13901, #7061 ) ;
#14900=DIRECTION ( 'NONE',  ( 8.018662683283438208E-16, -5.975035461963189015E-16, -1.000000000000000000 ) ) ;
#14901=CARTESIAN_POINT ( 'NONE',  ( -5.923714809816990723, -16.30043024566306187, 57.00231026484399166 ) ) ;
#14902=DIRECTION ( 'NONE',  ( 0.3857661296576155308, 0.9225966037272105291, -2.419218955996680478E-16 ) ) ;
#14904=VERTEX_POINT ( 'NONE', #9669 ) ;
#14906=CARTESIAN_POINT ( 'NONE',  ( -21.45979773411919567, -21.50599501901345789, 51.00231026484399166 ) ) ;
#14907=LINE ( 'NONE', #6776, #11828 ) ;
#14908=ORIENTED_EDGE ( 'NONE', *, *, #5212, .F. ) ;
#14910=VERTEX_POINT ( 'NONE', #14108 ) ;
#14911=CARTESIAN_POINT ( 'NONE',  ( -20.31707134655588121, -4.772760685475331499, 54.00231026484397745 ) ) ;
#14912=CARTESIAN_POINT ( 'NONE',  ( -11.97987666612771207, -20.77526002325937782, 56.85231026484400019 ) ) ;
#14914=PLANE ( 'NONE',  #68 ) ;
#14916=EDGE_CURVE ( 'NONE', #12154, #14904, #11887, .T. ) ;
#14917=DIRECTION ( 'NONE',  ( -0.8543800322332379960, -0.5196486895212294455, -3.746065934159121401E-16 ) ) ;
#14918=CARTESIAN_POINT ( 'NONE',  ( -15.19697172008446096, -10.92700001391350284, 51.00231026484399166 ) ) ;
#14919=DIRECTION ( 'NONE',  ( -8.018662683283438208E-16, 5.975035461963189015E-16, 1.000000000000000000 ) ) ;
#14921=ORIENTED_EDGE ( 'NONE', *, *, #13085, .T. ) ;
#14924=PLANE ( 'NONE',  #5930 ) ;
#14926=EDGE_LOOP ( 'NONE', ( #2883, #13136, #7890, #4557 ) ) ;
#14928=ORIENTED_EDGE ( 'NONE', *, *, #12178, .F. ) ;
#14930=AXIS2_PLACEMENT_3D ( 'NONE', #10110, #14637, #13348 ) ;
#14931=EDGE_CURVE ( 'NONE', #10921, #3108, #4932, .T. ) ;
#14932=DIRECTION ( 'NONE',  ( -0.6334982226805353500, 0.7737441449604661736, -9.702957262759963093E-16 ) ) ;
#14933=EDGE_CURVE ( 'NONE', #5527, #3941, #1410, .T. ) ;
#14934=EDGE_LOOP ( 'NONE', ( #3391, #6837, #3224, #10713 ) ) ;
#14936=ORIENTED_EDGE ( 'NONE', *, *, #12891, .F. ) ;
#14939=DIRECTION ( 'NONE',  ( -0.9085715390340231012, 0.4177292884839972076, -9.781476007338054812E-16 ) ) ;
#14940=ORIENTED_EDGE ( 'NONE', *, *, #10357, .F. ) ;
#14941=VERTEX_POINT ( 'NONE', #10742 ) ;
#14942=AXIS2_PLACEMENT_3D ( 'NONE', #11624, #14004, #7179 ) ;
#14946=ADVANCED_FACE ( 'NONE', ( #7359 ), #6132, .F. ) ;
#14953=EDGE_CURVE ( 'NONE', #6669, #11993, #12184, .T. ) ;
#14956=PLANE ( 'NONE',  #13497 ) ;
#14961=ORIENTED_EDGE ( 'NONE', *, *, #1554, .T. ) ;
#14963=ORIENTED_EDGE ( 'NONE', *, *, #2541, .F. ) ;
#14966=ORIENTED_EDGE ( 'NONE', *, *, #8456, .F. ) ;
#14968=AXIS2_PLACEMENT_3D ( 'NONE', #13159, #6171, #1820 ) ;
#14971=EDGE_CURVE ( 'NONE', #6233, #6222, #6302, .T. ) ;
#14972=CARTESIAN_POINT ( 'NONE',  ( -7.734307812155742923, -7.246443652516327383, 57.00231026484399166 ) ) ;
#14975=FACE_OUTER_BOUND ( 'NONE', #6668, .T. ) ;
#14976=ORIENTED_EDGE ( 'NONE', *, *, #12641, .T. ) ;
#14977=DIRECTION ( 'NONE',  ( -8.018662683283438208E-16, 5.975035461963189015E-16, 1.000000000000000000 ) ) ;
#14978=DIRECTION ( 'NONE',  ( -8.018662683283438208E-16, 5.975035461963189015E-16, 1.000000000000000000 ) ) ;
#14979=FACE_OUTER_BOUND ( 'NONE', #6049, .T. ) ;
#14982=FACE_OUTER_BOUND ( 'NONE', #1497, .T. ) ;
#14985=CARTESIAN_POINT ( 'NONE',  ( -15.49969986081091200, -13.50737899243823215, 48.00231026484398456 ) ) ;
#14986=CARTESIAN_POINT ( 'NONE',  ( -22.53804163936502647, -6.438972523632137346, 54.00231026484397745 ) ) ;
#14987=AXIS2_PLACEMENT_3D ( 'NONE', #8164, #11688, #10693 ) ;
#14989=VECTOR ( 'NONE', #13811, 1000.000000000000000 ) ;
#14990=DIRECTION ( 'NONE',  ( -8.018662683283438208E-16, 5.975035461963189015E-16, 1.000000000000000000 ) ) ;
#14994=DIRECTION ( 'NONE',  ( -8.018662683283438208E-16, 5.975035461963189015E-16, 1.000000000000000000 ) ) ;
#14995=ORIENTED_EDGE ( 'NONE', *, *, #1554, .F. ) ;
#14996=DIRECTION ( 'NONE',  ( -0.5975035461963217331, -0.8018662683283416248, 0.000000000000000000 ) ) ;
#14997=ORIENTED_EDGE ( 'NONE', *, *, #8139, .T. ) ;
#14998=DIRECTION ( 'NONE',  ( 0.6519834208811541298, 0.7582332219680880669, 6.975647374412577675E-17 ) ) ;
#15000=ADVANCED_FACE ( 'NONE', ( #2633 ), #8515, .F. ) ;
#15004=ORIENTED_EDGE ( 'NONE', *, *, #11324, .T. ) ;
#15006=DIRECTION ( 'NONE',  ( 0.5975035461963188466, 0.8018662683283437342, 0.000000000000000000 ) ) ;
#15007=AXIS2_PLACEMENT_3D ( 'NONE', #7925, #2125, #9304 ) ;
#15013=CARTESIAN_POINT ( 'NONE',  ( -24.36945568363038461, -11.58678490633884373, 57.00231026484397745 ) ) ;
#15014=VERTEX_POINT ( 'NONE', #5149 ) ;
#15015=DIRECTION ( 'NONE',  ( 8.018662683283438208E-16, -5.975035461963189015E-16, -1.000000000000000000 ) ) ;
#15016=ORIENTED_EDGE ( 'NONE', *, *, #15040, .T. ) ;
#15017=VERTEX_POINT ( 'NONE', #6506 ) ;
#15018=DIRECTION ( 'NONE',  ( -0.7737441449604673949, -0.6334982226805337957, -2.419218955996708581E-16 ) ) ;
#15021=LINE ( 'NONE', #12429, #3719 ) ;
#15022=VERTEX_POINT ( 'NONE', #2850 ) ;
#15026=AXIS2_PLACEMENT_3D ( 'NONE', #13006, #14067, #4895 ) ;
#15029=LINE ( 'NONE', #2261, #5807 ) ;
#15030=VERTEX_POINT ( 'NONE', #8812 ) ;
#15033=VERTEX_POINT ( 'NONE', #7438 ) ;
#15035=LINE ( 'NONE', #3265, #2257 ) ;
#15038=ORIENTED_EDGE ( 'NONE', *, *, #3088, .F. ) ;
#15039=LINE ( 'NONE', #5777, #3206 ) ;
#15040=EDGE_CURVE ( 'NONE', #7558, #8222, #12268, .T. ) ;
#15041=AXIS2_PLACEMENT_3D ( 'NONE', #11832, #14430, #10910 ) ;
#15042=LINE ( 'NONE', #6917, #12701 ) ;
#15043=EDGE_CURVE ( 'NONE', #13555, #7254, #9816, .T. ) ;
#15044=CARTESIAN_POINT ( 'NONE',  ( -8.791486474964742115, -6.124933722071904896, 56.85231026484398598 ) ) ;
#15045=DIRECTION ( 'NONE',  ( -8.018662683283438208E-16, 5.975035461963189015E-16, 1.000000000000000000 ) ) ;
#15046=FACE_OUTER_BOUND ( 'NONE', #6032, .T. ) ;
#15050=DIRECTION ( 'NONE',  ( 0.5975035461963189576, 0.8018662683283437342, 0.000000000000000000 ) ) ;
#15052=EDGE_CURVE ( 'NONE', #6890, #11369, #1560, .T. ) ;
#15054=CARTESIAN_POINT ( 'NONE',  ( -20.06719866676104402, -21.34952185377683165, 56.85231026484398598 ) ) ;
#15055=EDGE_CURVE ( 'NONE', #3406, #3165, #11195, .T. ) ;
#15057=FACE_OUTER_BOUND ( 'NONE', #11465, .T. ) ;
#15059=EDGE_CURVE ( 'NONE', #9104, #3051, #2783, .T. ) ;
#15060=DIRECTION ( 'NONE',  ( -0.5491495666976170531, 0.8357240892757724637, -9.396926207859082113E-16 ) ) ;
#15061=DIRECTION ( 'NONE',  ( 0.5975035461963189576, 0.8018662683283437342, 0.000000000000000000 ) ) ;
#15064=FACE_OUTER_BOUND ( 'NONE', #4791, .T. ) ;
#15065=VECTOR ( 'NONE', #4313, 1000.000000000000114 ) ;
#15068=DIRECTION ( 'NONE',  ( -8.018662683283438208E-16, 5.975035461963189015E-16, 1.000000000000000000 ) ) ;
#15069=ORIENTED_EDGE ( 'NONE', *, *, #12529, .F. ) ;
#15070=CARTESIAN_POINT ( 'NONE',  ( -15.49969986081092088, -13.50737899243822504, 57.00231026484397745 ) ) ;
#15071=VECTOR ( 'NONE', #3275, 999.9999999999998863 ) ;
#15072=EDGE_CURVE ( 'NONE', #6605, #10753, #7661, .T. ) ;
#15073=ORIENTED_EDGE ( 'NONE', *, *, #13765, .F. ) ;
#15076=ORIENTED_EDGE ( 'NONE', *, *, #13137, .F. ) ;
#15077=EDGE_CURVE ( 'NONE', #3452, #13179, #11116, .T. ) ;
#15079=ORIENTED_EDGE ( 'NONE', *, *, #7017, .T. ) ;
#15080=LINE ( 'NONE', #1931, #11230 ) ;
#15081=CARTESIAN_POINT ( 'NONE',  ( -6.426265323245524463, -13.69186664111786200, 56.85231026484400019 ) ) ;
#15082=PLANE ( 'NONE',  #982 ) ;
#15083=VECTOR ( 'NONE', #63, 1000.000000000000227 ) ;
#15084=EDGE_CURVE ( 'NONE', #858, #15022, #7514, .T. ) ;
#15085=VECTOR ( 'NONE', #14701, 1000.000000000000227 ) ;
#15091=ORIENTED_EDGE ( 'NONE', *, *, #8012, .T. ) ;
#15094=ORIENTED_EDGE ( 'NONE', *, *, #11504, .F. ) ;
#15095=AXIS2_PLACEMENT_3D ( 'NONE', #2186, #4409, #12598 ) ;
#15097=VECTOR ( 'NONE', #14733, 1000.000000000000227 ) ;
#15098=VECTOR ( 'NONE', #9799, 1000.000000000000114 ) ;
#15101=ADVANCED_FACE ( 'NONE', ( #5083 ), #5299, .F. ) ;
#15104=DIRECTION ( 'NONE',  ( -8.018662683283438208E-16, 5.975035461963189015E-16, 1.000000000000000000 ) ) ;
#15107=DIRECTION ( 'NONE',  ( 8.018662683283438208E-16, -5.975035461963189015E-16, -1.000000000000000000 ) ) ;
#15109=ORIENTED_EDGE ( 'NONE', *, *, #5100, .F. ) ;
#15110=PLANE ( 'NONE',  #14477 ) ;
#15111=CARTESIAN_POINT ( 'NONE',  ( -15.21745595230144232, -22.57829892241827352, 57.00231026484399166 ) ) ;
#15113=CARTESIAN_POINT ( 'NONE',  ( -13.41639018438039699, -15.05973874201012741, 51.00231026484399166 ) ) ;
#15114=ORIENTED_EDGE ( 'NONE', *, *, #3830, .F. ) ;
#15115=DIRECTION ( 'NONE',  ( -0.9578660637129379207, 0.2872152572324145892, -9.396926207859088029E-16 ) ) ;
#15116=LINE ( 'NONE', #3492, #1462 ) ;
#15119=CIRCLE ( 'NONE', #3401, 9.974999999999999645 ) ;
#15121=DIRECTION ( 'NONE',  ( -0.8357240892757725748, -0.5491495666976171641, -3.420201433256691137E-16 ) ) ;
#15122=DIRECTION ( 'NONE',  ( 8.018662683283438208E-16, -5.975035461963189015E-16, -1.000000000000000000 ) ) ;
#15123=ADVANCED_FACE ( 'NONE', ( #712 ), #5374, .T. ) ;
#15124=EDGE_LOOP ( 'NONE', ( #10597, #14976, #2761, #1832 ) ) ;
#15125=CARTESIAN_POINT ( 'NONE',  ( -15.49969986081092088, -13.50737899243822504, 57.00231026484397745 ) ) ;
ENDSEC;
END-ISO-10303-21;
